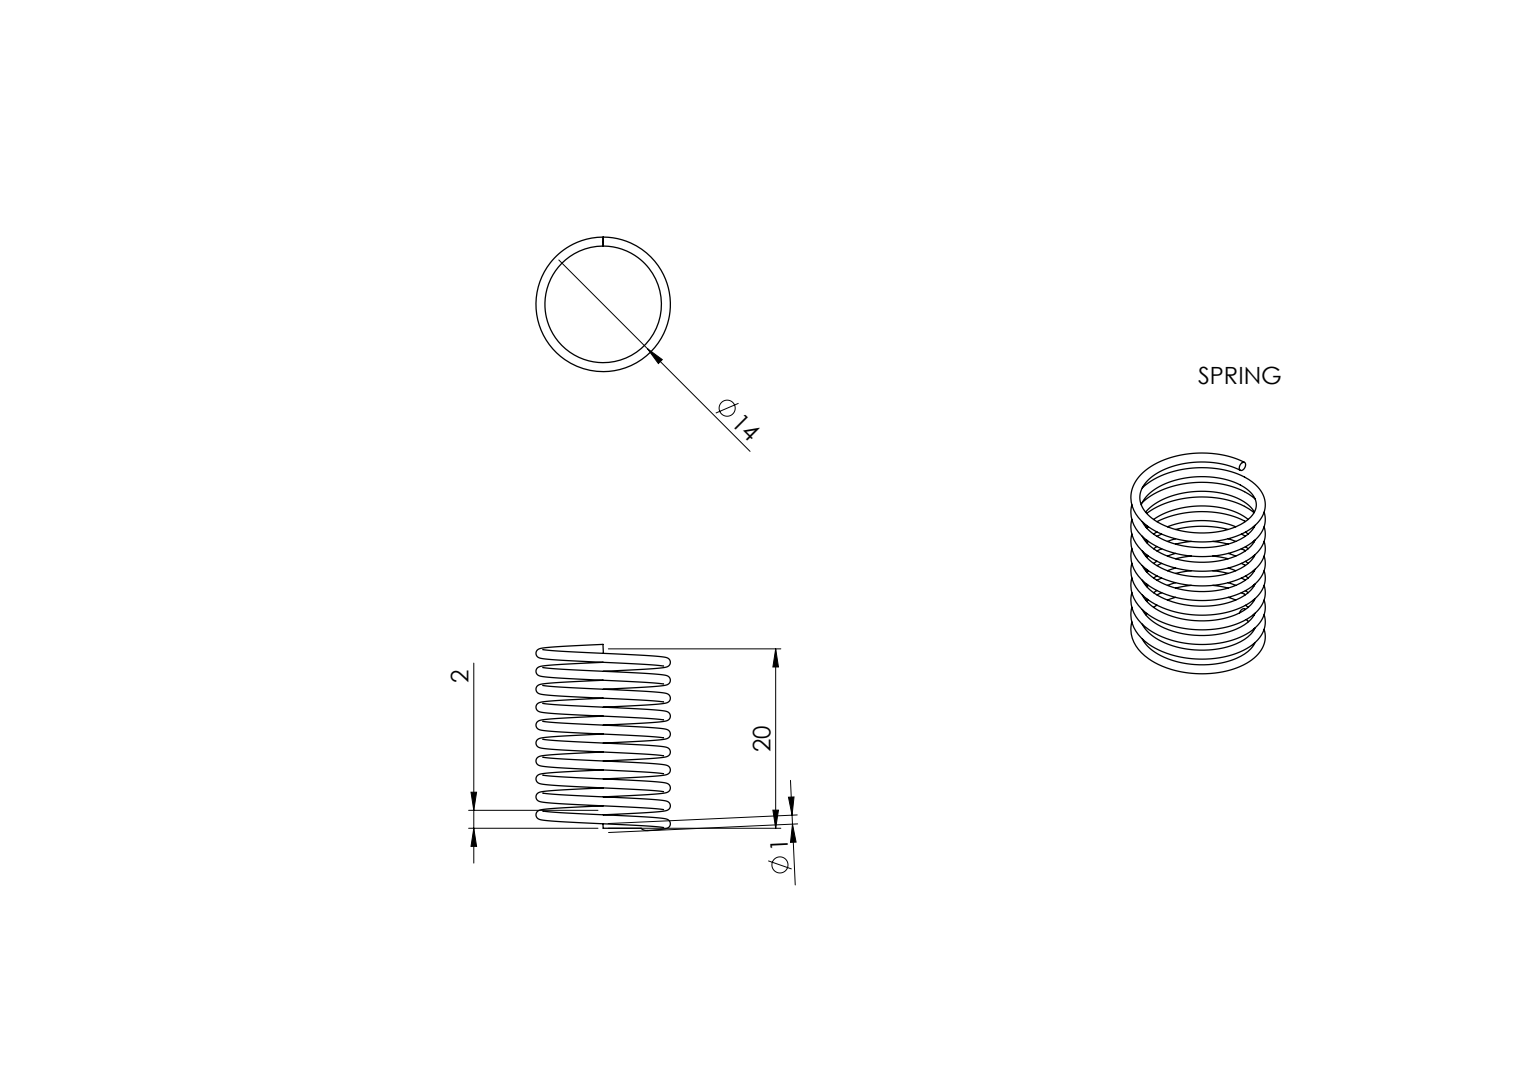
ISO-10303-21;
HEADER;
FILE_DESCRIPTION (('STEP AP214'),
    '1' );
FILE_NAME ('spring.step',
    '2026-10-25T07:12:54',
    ( '' ),
    ( '' ),
    'SwSTEP 2.0',
    'SolidWorks 2026',
    '' );
FILE_SCHEMA (( 'AUTOMOTIVE_DESIGN' ));
ENDSEC;

DATA;
#1=CARTESIAN_POINT ( 'NONE',  ( 44.30067958973594955, 46.10051614449766078, -1.875703265242155693 ) ) ;
#2=CARTESIAN_POINT ( 'NONE',  ( 43.33558569842706021, 59.90051614449766504, 2.141517661632167169 ) ) ;
#3=CARTESIAN_POINT ( 'NONE',  ( 56.81924384183011512, 48.19948385550240744, 4.924951120819313743 ) ) ;
#5=CARTESIAN_POINT ( 'NONE',  ( 49.97728705011495265, 53.50051614449767357, 8.000000000000001776 ) ) ;
#17=CARTESIAN_POINT ( 'NONE',  ( 44.28664221472220675, 51.09948385550240602, -1.832500667257165317 ) ) ;
#18=CARTESIAN_POINT ( 'NONE',  ( 44.03140696652193498, 63.19948385550240744, -4.306917132069424170 ) ) ;
#20=CARTESIAN_POINT ( 'NONE',  ( 47.70284917648459100, 63.60051614449766078, 6.992620115222796251 ) ) ;
#22=EDGE_CURVE ( 'NONE', #9726, #725, #6704, .T. ) ;
#26=CARTESIAN_POINT ( 'NONE',  ( 57.36023556966787851, 57.00051614449766646, 0.02388180880515038476 ) ) ;
#27=CARTESIAN_POINT ( 'NONE',  ( 55.69932041026404335, 55.89948385550241028, -1.875703265242203432 ) ) ;
#39=CARTESIAN_POINT ( 'NONE',  ( 54.13287192849676188, 50.29948385550240175, 5.649768623646098220 ) ) ;
#42=CARTESIAN_POINT ( 'NONE',  ( 51.97223112728249816, 54.60051614449766788, -5.992620115222793586 ) ) ;
#44=CARTESIAN_POINT ( 'NONE',  ( 49.97728705011488159, 65.49948385550240459, -7.000000000000000888 ) ) ;
#45=CARTESIAN_POINT ( 'NONE',  ( 56.65037692655918988, 61.89948385550241028, -2.184720259617163762 ) ) ;
#46=CARTESIAN_POINT ( 'NONE',  ( 56.65037692655918988, 57.89948385550240317, -2.184720259617163762 ) ) ;
#58=CARTESIAN_POINT ( 'NONE',  ( 56.66441430157296821, 48.09948385550240602, 2.141517661632100111 ) ) ;
#60=CARTESIAN_POINT ( 'NONE',  ( 56.66441430157294690, 48.90051614449766504, -2.141517661632166281 ) ) ;
#62=CARTESIAN_POINT ( 'NONE',  ( 47.42335538002188144, 62.59948385550238470, 8.007379884777233059 ) ) ;
#64=CARTESIAN_POINT ( 'NONE',  ( 56.79116909180255135, 53.79948385550241596, -4.963592699179005585 ) ) ;
#72=CARTESIAN_POINT ( 'NONE',  ( 55.08986747509849380, 47.20051614449766220, 3.727524721679155384 ) ) ;
#73=CARTESIAN_POINT ( 'NONE',  ( 52.25172492374528588, 57.40051614449765793, 7.007379884777204637 ) ) ;
#74=CARTESIAN_POINT ( 'NONE',  ( 52.57664461997811856, 45.59948385550240602, -8.007379884777229506 ) ) ;
#76=CARTESIAN_POINT ( 'NONE',  ( 58.41169779390614281, 55.00051614449766646, 0.02388180880515032231 ) ) ;
#86=CARTESIAN_POINT ( 'NONE',  ( 48.02776887271745210, 49.39948385550241028, -5.992620115222778487 ) ) ;
#88=CARTESIAN_POINT ( 'NONE',  ( 54.72065718078918906, 48.70051614449766930, -6.458785618021089192 ) ) ;
#91=CARTESIAN_POINT ( 'NONE',  ( 47.74827507625469281, 54.40051614449766504, -7.007379884777203749 ) ) ;
#92=CARTESIAN_POINT ( 'NONE',  ( 50.02271294988511841, 56.49948385550240459, 6.000000000000000888 ) ) ;
#107=CARTESIAN_POINT ( 'NONE',  ( 54.13287192849676188, 52.29948385550240886, 5.649768623646098220 ) ) ;
#109=CARTESIAN_POINT ( 'NONE',  ( 53.50833635130544508, 51.30051614449765651, 4.867452303228181343 ) ) ;
#113=CARTESIAN_POINT ( 'NONE',  ( 47.74827507625478518, 60.59948385550239891, 7.007379884777227730 ) ) ;
#125=CARTESIAN_POINT ( 'NONE',  ( 56.65037692655918988, 49.89948385550240317, -2.184720259617163762 ) ) ;
#126=CARTESIAN_POINT ( 'NONE',  ( 56.65037692655921120, 45.10051614449766078, 2.184720259617097593 ) ) ;
#128=CARTESIAN_POINT ( 'NONE',  ( 50.02271294988512551, 48.49948385550240459, 7.000000000000000888 ) ) ;
#130=CARTESIAN_POINT ( 'NONE',  ( 56.81924384183011512, 54.19948385550241454, 4.924951120819313743 ) ) ;
#138=CARTESIAN_POINT ( 'NONE',  ( 46.45491332379576477, 49.70051614449766220, 4.840751629271188961 ) ) ;
#139=CARTESIAN_POINT ( 'NONE',  ( 47.74827507625470702, 60.40051614449766504, -7.007379884777204637 ) ) ;
#140=CARTESIAN_POINT ( 'NONE',  ( 47.37792948025170858, 63.60051614449764656, 7.992620115222797139 ) ) ;
#143=CARTESIAN_POINT ( 'NONE',  ( 47.37792948025170858, 53.60051614449765367, 7.992620115222797139 ) ) ;
#144=B_SPLINE_CURVE_WITH_KNOTS ( 'NONE', 3,
 ( #13141, #2570, #7772, #10101, #12115, #12051, #4654, #11983, #6798, #4863, #3822, #8039 ),
 .UNSPECIFIED., .F., .F.,
 ( 4, 2, 2, 2, 2, 4 ),
 ( 0.01755862241325779893, 0.01812962329865995884, 0.01870062418406211874, 0.01984262595486643854, 0.02098462772567075835, 0.02212662949647507815 ),
 .UNSPECIFIED. ) ;
#155=CARTESIAN_POINT ( 'NONE',  ( 55.71335778527780747, 50.09948385550240602, 1.832500667257165983 ) ) ;
#156=CARTESIAN_POINT ( 'NONE',  ( 47.74827507625477807, 64.59948385550239891, 7.007379884777229506 ) ) ;
#158=CARTESIAN_POINT ( 'NONE',  ( 45.90387839640208512, 64.30051614449766362, -5.676469297603124353 ) ) ;
#161=CARTESIAN_POINT ( 'NONE',  ( 45.90387839640208512, 54.30051614449765651, -5.676469297603124353 ) ) ;
#162=CARTESIAN_POINT ( 'NONE',  ( 55.11794222512601493, 60.19948385550240744, 3.688883143319541702 ) ) ;
#170=CARTESIAN_POINT ( 'NONE',  ( 45.86712807150323812, 53.29948385550240886, -5.649768623646098220 ) ) ;
#172=CARTESIAN_POINT ( 'NONE',  ( 48.02776887271750184, 51.60051614449766788, 5.992620115222795363 ) ) ;
#176=CARTESIAN_POINT ( 'NONE',  ( 55.94051828345050836, 57.79948385550238754, -4.345558710429104465 ) ) ;
#185=( NAMED_UNIT ( * ) SI_UNIT ( $, .STERADIAN. ) SOLID_ANGLE_UNIT ( ) );
#187=CARTESIAN_POINT ( 'NONE',  ( 45.86712807150323812, 51.29948385550240175, -5.649768623646098220 ) ) ;
#188=CARTESIAN_POINT ( 'NONE',  ( 47.74827507625469281, 56.40051614449766504, -7.007379884777203749 ) ) ;
#191=CARTESIAN_POINT ( 'NONE',  ( 54.72065718078924590, 64.29948385550240175, 6.458785618021043895 ) ) ;
#196=CARTESIAN_POINT ( 'NONE',  ( 45.27934281921075410, 57.29948385550240175, -6.458785618021043895 ) ) ;
#203=CARTESIAN_POINT ( 'NONE',  ( 43.69122665457040000, 56.00051614449765935, -0.02388180880515696977 ) ) ;
#206=CARTESIAN_POINT ( 'NONE',  ( 54.68390685589033495, 45.69948385550240033, -6.485486291978119766 ) ) ;
#209=CARTESIAN_POINT ( 'NONE',  ( 45.27934281921082516, 53.70051614449766220, 6.458785618021089192 ) ) ;
#210=ORIENTED_EDGE ( 'NONE', *, *, #1266, .T. ) ;
#222=CARTESIAN_POINT ( 'NONE',  ( 51.97223112728254790, 50.39948385550241738, 5.992620115222778487 ) ) ;
#223=CARTESIAN_POINT ( 'NONE',  ( 43.33558569842703179, 63.09948385550240602, -2.141517661632099223 ) ) ;
#224=CARTESIAN_POINT ( 'NONE',  ( 41.58830220609386430, 48.00051614449766646, -0.02388180880514929535 ) ) ;
#228=CARTESIAN_POINT ( 'NONE',  ( 56.65037692655921120, 57.10051614449766078, 2.184720259617097593 ) ) ;
#230=CARTESIAN_POINT ( 'NONE',  ( 55.71335778527780747, 58.09948385550241312, 1.832500667257165983 ) ) ;
#238=CARTESIAN_POINT ( 'NONE',  ( 45.90387839640214196, 48.69948385550240744, 5.676469297603166098 ) ) ;
#240=CARTESIAN_POINT ( 'NONE',  ( 43.69122665457040000, 60.00051614449765935, -0.02388180880515696977 ) ) ;
#243=CARTESIAN_POINT ( 'NONE',  ( 52.29715082351547295, 60.39948385550239607, 6.992620115222774047 ) ) ;
#253=CARTESIAN_POINT ( 'NONE',  ( 43.34962307344081012, 54.89948385550240317, 2.184720259617164650 ) ) ;
#254=CARTESIAN_POINT ( 'NONE',  ( 56.65037692655921120, 55.10051614449766078, 2.184720259617097593 ) ) ;
#257=CARTESIAN_POINT ( 'NONE',  ( 43.33558569842703179, 49.09948385550240602, -2.141517661632099223 ) ) ;
#259=CARTESIAN_POINT ( 'NONE',  ( 47.42335538002188144, 62.59948385550238470, 8.007379884777233059 ) ) ;
#269=CARTESIAN_POINT ( 'NONE',  ( 46.45491332379576477, 51.70051614449765509, 4.840751629271188961 ) ) ;
#271=CARTESIAN_POINT ( 'NONE',  ( 52.57664461997811856, 51.59948385550240602, -8.007379884777229506 ) ) ;
#273=CARTESIAN_POINT ( 'NONE',  ( 55.96859303347804371, 56.19948385550241454, 4.306917132069425946 ) ) ;
#275=CARTESIAN_POINT ( 'NONE',  ( 47.42335538002180328, 58.40051614449765793, -8.007379884777206414 ) ) ;
#287=CARTESIAN_POINT ( 'NONE',  ( 50.02271294988511841, 54.49948385550240459, 6.000000000000000888 ) ) ;
#288=CARTESIAN_POINT ( 'NONE',  ( 44.03140696652198471, 47.80051614449764941, 4.306917132069485454 ) ) ;
#289=CARTESIAN_POINT ( 'NONE',  ( 52.25172492374527877, 63.40051614449765793, 7.007379884777203749 ) ) ;
#292=CARTESIAN_POINT ( 'NONE',  ( 47.70284917648459100, 59.60051614449765367, 6.992620115222796251 ) ) ;
#300=CARTESIAN_POINT ( 'NONE',  ( 55.94051828345050836, 55.79948385550238044, -4.345558710429104465 ) ) ;
#302=CARTESIAN_POINT ( 'NONE',  ( 48.07319477248762496, 60.40051614449765793, -6.007379884777208190 ) ) ;
#307=CARTESIAN_POINT ( 'NONE',  ( 56.65037692655918988, 63.89948385550239607, -2.184720259617163762 ) ) ;
#321=CARTESIAN_POINT ( 'NONE',  ( 50.02271294988512551, 54.49948385550240459, 7.000000000000000888 ) ) ;
#323=CARTESIAN_POINT ( 'NONE',  ( 56.66441430157294690, 54.90051614449765793, -2.141517661632166281 ) ) ;
#326=CARTESIAN_POINT ( 'NONE',  ( 45.90387839640214196, 54.69948385550240744, 5.676469297603166098 ) ) ;
#327=CARTESIAN_POINT ( 'NONE',  ( 55.94051828345050836, 49.79948385550240175, -4.345558710429104465 ) ) ;
#329=CARTESIAN_POINT ( 'NONE',  ( 50.02271294988513972, 64.49948385550239038, 8.000000000000001776 ) ) ;
#334=AXIS2_PLACEMENT_3D ( 'NONE', #11503, #2020, #12598 ) ;
#336=CARTESIAN_POINT ( 'NONE',  ( 48.07319477248762496, 54.40051614449765793, -6.007379884777208190 ) ) ;
#337=CARTESIAN_POINT ( 'NONE',  ( 47.74827507625470702, 64.40051614449765793, -7.007379884777204637 ) ) ;
#338=CARTESIAN_POINT ( 'NONE',  ( 56.79116909180255135, 49.79948385550240175, -4.963592699179005585 ) ) ;
#339=CARTESIAN_POINT ( 'NONE',  ( 43.33558569842703179, 59.09948385550240602, -2.141517661632099223 ) ) ;
#342=CARTESIAN_POINT ( 'NONE',  ( 47.42335538002180328, 60.40051614449765793, -8.007379884777206414 ) ) ;
#353=CARTESIAN_POINT ( 'NONE',  ( 53.50833635130540955, 59.69948385550240744, -4.867452303228209765 ) ) ;
#354=CARTESIAN_POINT ( 'NONE',  ( 43.34962307344078880, 50.10051614449766078, -2.184720259617096705 ) ) ;
#355=CARTESIAN_POINT ( 'NONE',  ( 52.57664461997821093, 55.40051614449767214, 8.007379884777206414 ) ) ;
#359=CARTESIAN_POINT ( 'NONE',  ( 52.29715082351538769, 62.60051614449766078, -6.992620115222796251 ) ) ;
#368=CARTESIAN_POINT ( 'NONE',  ( 47.74827507625478518, 54.59948385550239180, 7.007379884777227730 ) ) ;
#369=CARTESIAN_POINT ( 'NONE',  ( 44.91013252490150620, 58.20051614449766220, -3.727524721679154940 ) ) ;
#372=CARTESIAN_POINT ( 'NONE',  ( 43.33558569842706021, 45.90051614449765793, 2.141517661632167169 ) ) ;
#373=CARTESIAN_POINT ( 'NONE',  ( 55.71335778527780747, 46.09948385550240602, 1.832500667257165983 ) ) ;
#383=ADVANCED_BREP_SHAPE_REPRESENTATION ( '', ( #5648, #430 ), #3304 ) ;
#384=CARTESIAN_POINT ( 'NONE',  ( 44.05948171654945611, 52.20051614449764799, -4.345558710429044069 ) ) ;
#386=CARTESIAN_POINT ( 'NONE',  ( 55.94051828345050836, 49.79948385550240175, -4.345558710429104465 ) ) ;
#387=CARTESIAN_POINT ( 'NONE',  ( 57.36023556966787851, 47.99948385550239038, -0.02388180880522424582 ) ) ;
#388=CARTESIAN_POINT ( 'NONE',  ( 58.41169779390614281, 59.99948385550241170, -0.02388180880523160798 ) ) ;
#397=STYLED_ITEM('',(#13705),#5648);
#398=CARTESIAN_POINT ( 'NONE',  ( 48.02776887271750184, 55.60051614449765367, 5.992620115222795363 ) ) ;
#399=CARTESIAN_POINT ( 'NONE',  ( 45.86712807150329496, 63.70051614449766220, 5.649768623646139964 ) ) ;
#400=CARTESIAN_POINT ( 'NONE',  ( 49.97728705011486738, 51.49948385550240459, -8.000000000000001776 ) ) ;
#401=CARTESIAN_POINT ( 'NONE',  ( 54.13287192849676188, 56.29948385550240175, 5.649768623646098220 ) ) ;
#403=CARTESIAN_POINT ( 'NONE',  ( 56.81924384183006538, 60.80051614449766362, -4.924951120819380357 ) ) ;
#412=CARTESIAN_POINT ( 'NONE',  ( 49.97728705011488870, 53.49948385550240459, -6.000000000000000888 ) ) ;
#413=CARTESIAN_POINT ( 'NONE',  ( 56.13503143586221000, 44.82443585060838132, -3.788959942617806220 ) ) ;
#414=CARTESIAN_POINT ( 'NONE',  ( 56.79116909180259398, 53.20051614449766220, 4.963592699178938972 ) ) ;
#418=CARTESIAN_POINT ( 'NONE',  ( 54.13287192849671214, 60.70051614449766220, -5.649768623646139964 ) ) ;
#429=CARTESIAN_POINT ( 'NONE',  ( 52.29715082351547295, 60.39948385550239607, 6.992620115222774047 ) ) ;
#430=AXIS2_PLACEMENT_3D ( 'NONE', #5828, #10990, #3471 ) ;
#433=CARTESIAN_POINT ( 'NONE',  ( 43.69122665457040000, 56.00051614449765935, -0.02388180880515696977 ) ) ;
#436=CARTESIAN_POINT ( 'NONE',  ( 55.71335778527780036, 62.90051614449765083, -1.832500667257213056 ) ) ;
#437=CARTESIAN_POINT ( 'NONE',  ( 55.08986747509847248, 45.79948385550240886, -3.727524721679197572 ) ) ;
#449=CARTESIAN_POINT ( 'NONE',  ( 52.29715082351538769, 54.60051614449766788, -6.992620115222796251 ) ) ;
#451=CARTESIAN_POINT ( 'NONE',  ( 55.96859303347804371, 54.19948385550240033, 4.306917132069425946 ) ) ;
#452=CARTESIAN_POINT ( 'NONE',  ( 55.96859303347804371, 50.19948385550240744, 4.306917132069425946 ) ) ;
#455=CARTESIAN_POINT ( 'NONE',  ( 57.36023556966787851, 45.99948385550238328, -0.02388180880522424582 ) ) ;
#464=CARTESIAN_POINT ( 'NONE',  ( 50.02271294988506156, 52.50051614449766646, -6.000000000000000888 ) ) ;
#466=CARTESIAN_POINT ( 'NONE',  ( 52.62207051974839089, 50.39948385550241738, 7.992620115222770494 ) ) ;
#467=CARTESIAN_POINT ( 'NONE',  ( 43.34962307344081012, 58.89948385550241028, 2.184720259617164650 ) ) ;
#469=CARTESIAN_POINT ( 'NONE',  ( 45.31609314410960820, 64.30051614449766362, -6.485486291978072693 ) ) ;
#479=CARTESIAN_POINT ( 'NONE',  ( 48.07319477248768180, 54.59948385550240602, 6.007379884777225953 ) ) ;
#480=CARTESIAN_POINT ( 'NONE',  ( 42.63976443033212149, 48.00051614449766646, -0.02388180880514948964 ) ) ;
#481=CARTESIAN_POINT ( 'NONE',  ( 52.62207051974829852, 54.60051614449766788, -7.992620115222797139 ) ) ;
#485=CARTESIAN_POINT ( 'NONE',  ( 45.90387839640208512, 64.30051614449766362, -5.676469297603124353 ) ) ;
#494=CARTESIAN_POINT ( 'NONE',  ( 43.33558569842703179, 55.09948385550241312, -2.141517661632099223 ) ) ;
#496=CARTESIAN_POINT ( 'NONE',  ( 49.97728705011494554, 57.50051614449766646, 6.000000000000000888 ) ) ;
#500=CARTESIAN_POINT ( 'NONE',  ( 48.02776887271750184, 63.60051614449764656, 5.992620115222795363 ) ) ;
#501=CARTESIAN_POINT ( 'NONE',  ( 47.70284917648453415, 63.39948385550240317, -6.992620115222774047 ) ) ;
#506=UNCERTAINTY_MEASURE_WITH_UNIT (LENGTH_MEASURE( 1.000000000000000082E-05 ), #4482, 'distance_accuracy_value', 'NONE');
#514=CARTESIAN_POINT ( 'NONE',  ( 57.36023556966787851, 57.00051614449766646, 0.02388180880515038476 ) ) ;
#518=CARTESIAN_POINT ( 'NONE',  ( 43.34962307344081012, 48.89948385550240317, 2.184720259617164650 ) ) ;
#519=CARTESIAN_POINT ( 'NONE',  ( 56.81924384183011512, 60.19948385550240744, 4.924951120819313743 ) ) ;
#527=CARTESIAN_POINT ( 'NONE',  ( 43.69122665457040000, 64.00051614449765225, -0.02388180880515696977 ) ) ;
#530=CARTESIAN_POINT ( 'NONE',  ( 45.27934281921075410, 53.29948385550240886, -6.458785618021043895 ) ) ;
#531=CARTESIAN_POINT ( 'NONE',  ( 54.09612160359786515, 53.69948385550240744, -5.676469297603166098 ) ) ;
#534=CARTESIAN_POINT ( 'NONE',  ( 42.39856655714564226, 62.10051614449765367, -2.493737253992044156 ) ) ;
#544=CARTESIAN_POINT ( 'NONE',  ( 51.97223112728254790, 56.39948385550241028, 5.992620115222778487 ) ) ;
#545=CARTESIAN_POINT ( 'NONE',  ( 56.65037692655921120, 53.10051614449766078, 2.184720259617097593 ) ) ;
#546=CARTESIAN_POINT ( 'NONE',  ( 41.58830220609386430, 54.00051614449765935, -0.02388180880514929535 ) ) ;
#549=CARTESIAN_POINT ( 'NONE',  ( 43.33558569842706021, 63.90051614449765793, 2.141517661632167169 ) ) ;
#556=CARTESIAN_POINT ( 'NONE',  ( 55.96859303347804371, 58.19948385550241454, 4.306917132069425946 ) ) ;
#557=CARTESIAN_POINT ( 'NONE',  ( 43.33558569842703179, 55.09948385550241312, -2.141517661632099223 ) ) ;
#563=CARTESIAN_POINT ( 'NONE',  ( 44.03140696652198471, 45.80051614449764230, 4.306917132069485454 ) ) ;
#564=CARTESIAN_POINT ( 'NONE',  ( 47.70284917648453415, 65.39948385550239607, -6.992620115222774047 ) ) ;
#574=CARTESIAN_POINT ( 'NONE',  ( 54.09612160359792199, 61.30051614449766362, 5.676469297603124353 ) ) ;
#577=CARTESIAN_POINT ( 'NONE',  ( 45.90387839640214196, 60.69948385550240033, 5.676469297603166098 ) ) ;
#578=CARTESIAN_POINT ( 'NONE',  ( 47.74827507625478518, 50.59948385550238470, 7.007379884777227730 ) ) ;
#586=CARTESIAN_POINT ( 'NONE',  ( 51.92680522751238925, 59.40051614449765793, 6.007379884777208190 ) ) ;
#589=CARTESIAN_POINT ( 'NONE',  ( 50.02271294988513972, 62.49948385550240459, 8.000000000000001776 ) ) ;
#591=CARTESIAN_POINT ( 'NONE',  ( 43.34962307344081012, 62.89948385550241028, 2.184720259617164650 ) ) ;
#593=CARTESIAN_POINT ( 'NONE',  ( 43.20883090819745576, 50.79948385550240175, 4.963592699179006473 ) ) ;
#605=CARTESIAN_POINT ( 'NONE',  ( 51.97223112728254790, 60.39948385550241028, 5.992620115222778487 ) ) ;
#606=CARTESIAN_POINT ( 'NONE',  ( 56.66441430157294690, 52.90051614449765793, -2.141517661632166281 ) ) ;
#607=CARTESIAN_POINT ( 'NONE',  ( 42.38452918213190657, 61.90051614449766504, 2.450534656007115508 ) ) ;
#611=CARTESIAN_POINT ( 'NONE',  ( 54.09612160359792199, 63.30051614449766362, 5.676469297603124353 ) ) ;
#621=CARTESIAN_POINT ( 'NONE',  ( 53.50833635130540955, 45.69948385550240033, -4.867452303228209765 ) ) ;
#622=CARTESIAN_POINT ( 'NONE',  ( 56.66441430157296821, 56.09948385550240602, 2.141517661632100111 ) ) ;
#628=CARTESIAN_POINT ( 'NONE',  ( 53.50833635130544508, 63.30051614449767072, 4.867452303228181343 ) ) ;
#629=CARTESIAN_POINT ( 'NONE',  ( 48.02776887271745210, 51.39948385550241028, -5.992620115222778487 ) ) ;
#641=CARTESIAN_POINT ( 'NONE',  ( 45.86712807150329496, 59.70051614449766220, 5.649768623646139964 ) ) ;
#643=CARTESIAN_POINT ( 'NONE',  ( 44.88205777487398507, 65.19948385550240744, -3.688883143319540814 ) ) ;
#645=CARTESIAN_POINT ( 'NONE',  ( 44.03140696652192787, 61.19948385550239323, -4.306917132069425058 ) ) ;
#646=CARTESIAN_POINT ( 'NONE',  ( 54.09612160359786515, 51.69948385550240744, -5.676469297603166098 ) ) ;
#647=CARTESIAN_POINT ( 'NONE',  ( 56.66441430157296821, 50.09948385550240602, 2.141517661632100111 ) ) ;
#657=CARTESIAN_POINT ( 'NONE',  ( 55.11794222512599362, 60.80051614449766362, -3.688883143319583446 ) ) ;
#659=CARTESIAN_POINT ( 'NONE',  ( 47.37792948025162332, 61.39948385550240317, -7.992620115222770494 ) ) ;
#663=CARTESIAN_POINT ( 'NONE',  ( 56.79116909180255135, 47.79948385550240886, -4.963592699179005585 ) ) ;
#676=CARTESIAN_POINT ( 'NONE',  ( 55.11794222512599362, 44.80051614449766362, -3.688883143319583446 ) ) ;
#677=CARTESIAN_POINT ( 'NONE',  ( 45.86712807150329496, 53.70051614449766220, 5.649768623646139964 ) ) ;
#678=CARTESIAN_POINT ( 'NONE',  ( 42.39856655714564226, 56.10051614449766078, -2.493737253992044156 ) ) ;
#684=CARTESIAN_POINT ( 'NONE',  ( 42.38452918213190657, 49.90051614449766504, 2.450534656007115508 ) ) ;
#697=CARTESIAN_POINT ( 'NONE',  ( 43.33558569842703179, 65.09948385550239891, -2.141517661632099223 ) ) ;
#698=CARTESIAN_POINT ( 'NONE',  ( 42.63976443033212149, 58.99948385550239038, 0.02388180880522514787 ) ) ;
#702=CARTESIAN_POINT ( 'NONE',  ( 49.97728705011495265, 53.50051614449765935, 7.000000000000000888 ) ) ;
#703=CARTESIAN_POINT ( 'NONE',  ( 51.92680522751233951, 49.59948385550241312, -6.007379884777223289 ) ) ;
#716=CARTESIAN_POINT ( 'NONE',  ( 55.71335778527780036, 44.90051614449765793, -1.832500667257213056 ) ) ;
#718=CARTESIAN_POINT ( 'NONE',  ( 43.33558569842703179, 57.09948385550240602, -2.141517661632099223 ) ) ;
#719=CARTESIAN_POINT ( 'NONE',  ( 44.03140696652192787, 53.19948385550238612, -4.306917132069425058 ) ) ;
#721=CARTESIAN_POINT ( 'NONE',  ( 44.03140696652192787, 51.19948385550238612, -4.306917132069425058 ) ) ;
#724=CARTESIAN_POINT ( 'NONE',  ( 62.49999999999998579, 45.00000000000001421, -5.000000000000000000 ) ) ;
#725=VERTEX_POINT ( 'NONE', #11778 ) ;
#731=CARTESIAN_POINT ( 'NONE',  ( 44.28664221472221385, 57.90051614449765793, 1.832500667257213722 ) ) ;
#733=CARTESIAN_POINT ( 'NONE',  ( 42.39856655714566358, 56.89948385550240317, 2.493737253992119207 ) ) ;
#734=CARTESIAN_POINT ( 'NONE',  ( 45.86712807150323812, 63.29948385550240886, -5.649768623646098220 ) ) ;
#737=CARTESIAN_POINT ( 'NONE',  ( 54.68390685589033495, 51.69948385550241454, -6.485486291978119766 ) ) ;
#745=B_SPLINE_CURVE_WITH_KNOTS ( 'NONE', 3,
 ( #13610, #3044, #9471, #11483, #1864, #10442 ),
 .UNSPECIFIED., .F., .F.,
 ( 4, 2, 4 ),
 ( 0.000000000000000000, 0.0003657767439067419277, 0.0007315534878134838555 ),
 .UNSPECIFIED. ) ;
#750=CARTESIAN_POINT ( 'NONE',  ( 43.69122665457040000, 64.99948385550240459, 0.02388180880521036456 ) ) ;
#751=CARTESIAN_POINT ( 'NONE',  ( 47.74827507625470702, 52.40051614449765083, -7.007379884777204637 ) ) ;
#753=CARTESIAN_POINT ( 'NONE',  ( 45.27934281921082516, 57.70051614449766930, 6.458785618021089192 ) ) ;
#756=CARTESIAN_POINT ( 'NONE',  ( 56.81924384183006538, 52.80051614449766362, -4.924951120819380357 ) ) ;
#767=CARTESIAN_POINT ( 'NONE',  ( 44.91013252490152752, 46.79948385550240886, 3.727524721679198461 ) ) ;
#768=CARTESIAN_POINT ( 'NONE',  ( 45.90387839640214196, 60.69948385550240033, 5.676469297603166098 ) ) ;
#774=CARTESIAN_POINT ( 'NONE',  ( 47.70284917648459100, 53.60051614449765367, 6.992620115222796251 ) ) ;
#775=CARTESIAN_POINT ( 'NONE',  ( 44.28664221472220675, 55.09948385550241312, -1.832500667257165317 ) ) ;
#786=CARTESIAN_POINT ( 'NONE',  ( 49.97728705011488159, 47.49948385550240459, -7.000000000000000888 ) ) ;
#789=CARTESIAN_POINT ( 'NONE',  ( 48.02776887271750184, 45.60051614449765367, 5.992620115222795363 ) ) ;
#791=CARTESIAN_POINT ( 'NONE',  ( 54.09612160359786515, 55.69948385550240744, -5.676469297603166098 ) ) ;
#792=CARTESIAN_POINT ( 'NONE',  ( 55.94051828345050836, 51.79948385550240175, -4.345558710429104465 ) ) ;
#794=CARTESIAN_POINT ( 'NONE',  ( 54.13287192849676188, 52.29948385550240886, 5.649768623646098220 ) ) ;
#797=LINE ( 'NONE', #724, #5719 ) ;
#802=CARTESIAN_POINT ( 'NONE',  ( 43.69122665457040000, 60.00051614449765935, -0.02388180880515696977 ) ) ;
#804=CARTESIAN_POINT ( 'NONE',  ( 58.41169779390614281, 61.99948385550241170, -0.02388180880523160798 ) ) ;
#806=CARTESIAN_POINT ( 'NONE',  ( 45.31609314410967926, 50.69948385550240744, 6.485486291978119766 ) ) ;
#815=CARTESIAN_POINT ( 'NONE',  ( 46.49166364869460466, 64.69948385550240744, 4.867452303228209765 ) ) ;
#816=CARTESIAN_POINT ( 'NONE',  ( 44.05948171654945611, 56.20051614449765509, -4.345558710429044069 ) ) ;
#817=CARTESIAN_POINT ( 'NONE',  ( 52.57664461997821093, 61.40051614449765793, 8.007379884777206414 ) ) ;
#819=CARTESIAN_POINT ( 'NONE',  ( 57.60143344285435774, 47.10051614449766078, 2.493737253992045044 ) ) ;
#829=CARTESIAN_POINT ( 'NONE',  ( 47.74827507625478518, 64.59948385550239891, 7.007379884777227730 ) ) ;
#831=CARTESIAN_POINT ( 'NONE',  ( 52.29715082351547295, 56.39948385550239607, 6.992620115222774047 ) ) ;
#836=CARTESIAN_POINT ( 'NONE',  ( 55.48859070151218020, 45.00000000000002132, -4.999999999999993783 ) ) ;
#837=CARTESIAN_POINT ( 'NONE',  ( 54.13287192849671214, 50.70051614449766220, -5.649768623646139964 ) ) ;
#838=CARTESIAN_POINT ( 'NONE',  ( 49.97728705011488870, 49.49948385550241170, -6.000000000000000888 ) ) ;
#839=CARTESIAN_POINT ( 'NONE',  ( 55.00886502606627459, 44.74918607449495767, -5.000000000000008882 ) ) ;
#858=CARTESIAN_POINT ( 'NONE',  ( 51.92680522751233951, 63.59948385550239891, -6.007379884777223289 ) ) ;
#861=CARTESIAN_POINT ( 'NONE',  ( 55.96859303347804371, 56.19948385550241454, 4.306917132069425946 ) ) ;
#863=CARTESIAN_POINT ( 'NONE',  ( 44.05948171654949874, 50.79948385550238754, 4.345558710429105354 ) ) ;
#872=CARTESIAN_POINT ( 'NONE',  ( 55.96859303347805081, 46.19948385550240033, 4.306917132069425058 ) ) ;
#873=CARTESIAN_POINT ( 'NONE',  ( 54.09612160359792199, 49.30051614449765651, 5.676469297603124353 ) ) ;
#874=CARTESIAN_POINT ( 'NONE',  ( 54.23491683972284960, 45.00000000000001421, -4.999999999999999112 ) ) ;
#875=CARTESIAN_POINT ( 'NONE',  ( 56.79116909180255135, 61.79948385550240175, -4.963592699179005585 ) ) ;
#879=CARTESIAN_POINT ( 'NONE',  ( 47.42335538002188144, 48.59948385550239891, 8.007379884777233059 ) ) ;
#890=CARTESIAN_POINT ( 'NONE',  ( 55.71335778527780747, 60.09948385550240602, 1.832500667257165983 ) ) ;
#891=CARTESIAN_POINT ( 'NONE',  ( 55.94051828345054389, 57.20051614449766220, 4.345558710429044957 ) ) ;
#892=CARTESIAN_POINT ( 'NONE',  ( 42.38452918213190657, 57.90051614449765793, 2.450534656007115508 ) ) ;
#894=CARTESIAN_POINT ( 'NONE',  ( 50.02271294988505446, 52.50051614449766646, -8.000000000000001776 ) ) ;
#903=DIRECTION ( 'NONE',  ( -0.04542589977017699732, 0.9989677110047501252, 0.000000000000000000 ) ) ;
#906=CARTESIAN_POINT ( 'NONE',  ( 49.97728705011488159, 61.49948385550240459, -7.000000000000000888 ) ) ;
#908=CARTESIAN_POINT ( 'NONE',  ( 43.33558569842703179, 57.09948385550240602, -2.141517661632099223 ) ) ;
#911=CARTESIAN_POINT ( 'NONE',  ( 54.09612160359792199, 57.30051614449765651, 5.676469297603124353 ) ) ;
#915=CARTESIAN_POINT ( 'NONE',  ( 47.74827507625469281, 50.40051614449764372, -7.007379884777203749 ) ) ;
#916=CARTESIAN_POINT ( 'NONE',  ( 55.71335778527780747, 50.09948385550240602, 1.832500667257165983 ) ) ;
#930=CARTESIAN_POINT ( 'NONE',  ( 44.91013252490150620, 48.20051614449766930, -3.727524721679154940 ) ) ;
#933=CARTESIAN_POINT ( 'NONE',  ( 55.94051828345050836, 61.79948385550239465, -4.345558710429104465 ) ) ;
#934=CARTESIAN_POINT ( 'NONE',  ( 55.96859303347804371, 54.19948385550240033, 4.306917132069425946 ) ) ;
#937=ORIENTED_EDGE ( 'NONE', *, *, #11649, .F. ) ;
#938=CARTESIAN_POINT ( 'NONE',  ( 49.97728705011488159, 53.49948385550240459, -7.000000000000000888 ) ) ;
#946=CARTESIAN_POINT ( 'NONE',  ( 55.96859303347802239, 48.80051614449766362, -4.306917132069484566 ) ) ;
#948=CARTESIAN_POINT ( 'NONE',  ( 42.38452918213188525, 65.09948385550239891, -2.450534656007040013 ) ) ;
#949=CARTESIAN_POINT ( 'NONE',  ( 42.39856655714566358, 56.89948385550240317, 2.493737253992119207 ) ) ;
#956=CARTESIAN_POINT ( 'NONE',  ( 44.28664221472221385, 47.90051614449765793, 1.832500667257213722 ) ) ;
#957=CARTESIAN_POINT ( 'NONE',  ( 44.05948171654945611, 62.20051614449765509, -4.345558710429044069 ) ) ;
#959=CARTESIAN_POINT ( 'NONE',  ( 47.42335538002188144, 46.59948385550239891, 8.007379884777233059 ) ) ;
#964=CARTESIAN_POINT ( 'NONE',  ( 52.57664461997821093, 47.40051614449765793, 8.007379884777206414 ) ) ;
#976=CARTESIAN_POINT ( 'NONE',  ( 49.97728705011488870, 47.49948385550240459, -6.000000000000000888 ) ) ;
#978=CARTESIAN_POINT ( 'NONE',  ( 42.63976443033212860, 58.00051614449765225, -0.02388180880514948964 ) ) ;
#982=CARTESIAN_POINT ( 'NONE',  ( 50.02271294988505446, 52.50051614449765935, -7.000000000000000888 ) ) ;
#983=CARTESIAN_POINT ( 'NONE',  ( 55.71335778527780747, 56.09948385550240602, 1.832500667257165983 ) ) ;
#997=CARTESIAN_POINT ( 'NONE',  ( 49.97728705011494554, 53.50051614449767357, 6.000000000000000888 ) ) ;
#999=CARTESIAN_POINT ( 'NONE',  ( 54.13287192849676188, 62.29948385550240886, 5.649768623646098220 ) ) ;
#1000=CARTESIAN_POINT ( 'NONE',  ( 45.90387839640214196, 60.69948385550240033, 5.676469297603166098 ) ) ;
#1001=CARTESIAN_POINT ( 'NONE',  ( 52.25172492374522903, 61.59948385550239891, -7.007379884777225953 ) ) ;
#1008=CARTESIAN_POINT ( 'NONE',  ( 50.02271294988512551, 46.49948385550240459, 7.000000000000000888 ) ) ;
#1010=CARTESIAN_POINT ( 'NONE',  ( 45.90387839640208512, 50.30051614449766362, -5.676469297603124353 ) ) ;
#1014=CARTESIAN_POINT ( 'NONE',  ( 45.90387839640214196, 46.69948385550240744, 5.676469297603166098 ) ) ;
#1016=PLANE ( 'NONE',  #1563 ) ;
#1017=CARTESIAN_POINT ( 'NONE',  ( 42.39856655714566358, 58.89948385550241028, 2.493737253992119207 ) ) ;
#1026=CARTESIAN_POINT ( 'NONE',  ( 44.30067958973594955, 50.10051614449766078, -1.875703265242155693 ) ) ;
#1027=CARTESIAN_POINT ( 'NONE',  ( 45.90387839640208512, 58.30051614449766362, -5.676469297603124353 ) ) ;
#1028=CARTESIAN_POINT ( 'NONE',  ( 42.39856655714566358, 46.89948385550240317, 2.493737253992119207 ) ) ;
#1031=CARTESIAN_POINT ( 'NONE',  ( 45.27934281921082516, 57.70051614449766930, 6.458785618021089192 ) ) ;
#1039=CARTESIAN_POINT ( 'NONE',  ( 49.97728705011488870, 51.49948385550240459, -6.000000000000000888 ) ) ;
#1041=CARTESIAN_POINT ( 'NONE',  ( 50.02271294988505446, 46.50051614449766646, -8.000000000000001776 ) ) ;
#1045=CARTESIAN_POINT ( 'NONE',  ( 52.25172492374527877, 55.40051614449764372, 7.007379884777203749 ) ) ;
#1046=CARTESIAN_POINT ( 'NONE',  ( 46.45491332379572924, 61.29948385550240886, -4.840751629271157874 ) ) ;
#1058=CARTESIAN_POINT ( 'NONE',  ( 42.63976443033212860, 50.99948385550240459, 0.02388180880522514787 ) ) ;
#1060=CARTESIAN_POINT ( 'NONE',  ( 44.30067958973594955, 52.10051614449766788, -1.875703265242155693 ) ) ;
#1062=CARTESIAN_POINT ( 'NONE',  ( 43.33558569842703179, 63.09948385550240602, -2.141517661632099223 ) ) ;
#1063=CARTESIAN_POINT ( 'NONE',  ( 54.09612160359786515, 61.69948385550240744, -5.676469297603166098 ) ) ;
#1064=CARTESIAN_POINT ( 'NONE',  ( 45.90387839640214196, 62.69948385550240744, 5.676469297603166098 ) ) ;
#1072=CARTESIAN_POINT ( 'NONE',  ( 44.05948171654949874, 46.79948385550240175, 4.345558710429104465 ) ) ;
#1073=CARTESIAN_POINT ( 'NONE',  ( 47.70284917648459100, 49.60051614449763946, 6.992620115222796251 ) ) ;
#1075=CARTESIAN_POINT ( 'NONE',  ( 43.33558569842703179, 47.09948385550240602, -2.141517661632099223 ) ) ;
#1078=CARTESIAN_POINT ( 'NONE',  ( 42.38452918213188525, 59.09948385550240602, -2.450534656007040013 ) ) ;
#1089=CARTESIAN_POINT ( 'NONE',  ( 48.02776887271750184, 49.60051614449766788, 5.992620115222795363 ) ) ;
#1090=CARTESIAN_POINT ( 'NONE',  ( 56.66441430157294690, 60.90051614449766504, -2.141517661632166281 ) ) ;
#1092=CARTESIAN_POINT ( 'NONE',  ( 57.61547081786810764, 62.90051614449765083, -2.450534656007114176 ) ) ;
#1096=CARTESIAN_POINT ( 'NONE',  ( 43.20883090819742023, 58.20051614449766220, -4.963592699178938972 ) ) ;
#1107=CARTESIAN_POINT ( 'NONE',  ( 55.69932041026404335, 47.89948385550240317, -1.875703265242203432 ) ) ;
#1108=CARTESIAN_POINT ( 'NONE',  ( 50.02271294988512551, 64.49948385550240459, 7.000000000000000888 ) ) ;
#1109=CARTESIAN_POINT ( 'NONE',  ( 56.81924384183006538, 46.80051614449766362, -4.924951120819380357 ) ) ;
#1113=CARTESIAN_POINT ( 'NONE',  ( 45.90387839640208512, 60.30051614449766362, -5.676469297603124353 ) ) ;
#1114=CARTESIAN_POINT ( 'NONE',  ( 48.02776887271745210, 61.39948385550240317, -5.992620115222778487 ) ) ;
#1126=CARTESIAN_POINT ( 'NONE',  ( 44.03140696652192787, 49.19948385550240033, -4.306917132069425058 ) ) ;
#1128=CARTESIAN_POINT ( 'NONE',  ( 43.69122665457040000, 50.00051614449765935, -0.02388180880515696977 ) ) ;
#1132=CARTESIAN_POINT ( 'NONE',  ( 52.25172492374522903, 59.59948385550240602, -7.007379884777225953 ) ) ;
#1147=CARTESIAN_POINT ( 'NONE',  ( 56.65037692655918988, 53.89948385550240317, -2.184720259617163762 ) ) ;
#1150=CARTESIAN_POINT ( 'NONE',  ( 52.29715082351538769, 44.60051614449766788, -6.992620115222796251 ) ) ;
#1152=CARTESIAN_POINT ( 'NONE',  ( 47.37792948025162332, 63.39948385550238896, -7.992620115222770494 ) ) ;
#1154=CARTESIAN_POINT ( 'NONE',  ( 45.31609314410967926, 58.69948385550240033, 6.485486291978119766 ) ) ;
#1157=ORIENTED_EDGE ( 'NONE', *, *, #10798, .T. ) ;
#1164=CARTESIAN_POINT ( 'NONE',  ( 48.07319477248762496, 48.40051614449766504, -6.007379884777208190 ) ) ;
#1165=CARTESIAN_POINT ( 'NONE',  ( 45.86712807150329496, 61.70051614449766220, 5.649768623646139964 ) ) ;
#1166=CARTESIAN_POINT ( 'NONE',  ( 47.37792948025162332, 47.39948385550241028, -7.992620115222770494 ) ) ;
#1168=CARTESIAN_POINT ( 'NONE',  ( 50.02271294988505446, 58.50051614449765225, -8.000000000000001776 ) ) ;
#1178=CARTESIAN_POINT ( 'NONE',  ( 44.28664221472220675, 47.09948385550240602, -1.832500667257165317 ) ) ;
#1179=CARTESIAN_POINT ( 'NONE',  ( 50.02271294988512551, 62.49948385550240459, 7.000000000000000888 ) ) ;
#1180=CARTESIAN_POINT ( 'NONE',  ( 49.97728705011495265, 45.50051614449766646, 8.000000000000001776 ) ) ;
#1183=CARTESIAN_POINT ( 'NONE',  ( 47.70284917648459100, 55.60051614449764656, 6.992620115222796251 ) ) ;
#1184=CARTESIAN_POINT ( 'NONE',  ( 44.30067958973596376, 60.89948385550241028, 1.875703265242204099 ) ) ;
#1198=CARTESIAN_POINT ( 'NONE',  ( 44.05948171654949874, 50.79948385550238754, 4.345558710429105354 ) ) ;
#1202=CARTESIAN_POINT ( 'NONE',  ( 43.69122665457040000, 52.00051614449766646, -0.02388180880515696977 ) ) ;
#1206=CARTESIAN_POINT ( 'NONE',  ( 50.02271294988512551, 58.49948385550241170, 7.000000000000000888 ) ) ;
#1216=CARTESIAN_POINT ( 'NONE',  ( 47.70284917648453415, 55.39948385550239607, -6.992620115222774047 ) ) ;
#1217=CARTESIAN_POINT ( 'NONE',  ( 47.70284917648459100, 55.60051614449764656, 6.992620115222796251 ) ) ;
#1219=CARTESIAN_POINT ( 'NONE',  ( 56.66441430157296821, 46.09948385550240602, 2.141517661632100111 ) ) ;
#1221=CARTESIAN_POINT ( 'NONE',  ( 42.38452918213188525, 57.09948385550240602, -2.450534656007040013 ) ) ;
#1222=ORIENTED_EDGE ( 'NONE', *, *, #8044, .T. ) ;
#1228=CARTESIAN_POINT ( 'NONE',  ( 44.91013252490150620, 46.20051614449766220, -3.727524721679154940 ) ) ;
#1229=CARTESIAN_POINT ( 'NONE',  ( 50.02271294988505446, 64.50051614449765225, -7.000000000000000888 ) ) ;
#1230=CARTESIAN_POINT ( 'NONE',  ( 49.97728705011486738, 47.49948385550240459, -8.000000000000001776 ) ) ;
#1231=CARTESIAN_POINT ( 'NONE',  ( 52.62207051974829852, 56.60051614449765367, -7.992620115222797139 ) ) ;
#1240=CARTESIAN_POINT ( 'NONE',  ( 55.11794222512601493, 52.19948385550240744, 3.688883143319541702 ) ) ;
#1241=CARTESIAN_POINT ( 'NONE',  ( 43.33558569842703179, 65.09948385550239891, -2.141517661632099223 ) ) ;
#1242=CARTESIAN_POINT ( 'NONE',  ( 43.18075615816994173, 47.80051614449764941, 4.924951120819380357 ) ) ;
#1245=CARTESIAN_POINT ( 'NONE',  ( 47.74827507625469281, 58.40051614449766504, -7.007379884777203749 ) ) ;
#1246=CARTESIAN_POINT ( 'NONE',  ( 55.08986747509847248, 55.79948385550239465, -3.727524721679197572 ) ) ;
#1253=CARTESIAN_POINT ( 'NONE',  ( 49.97728705011488159, 49.49948385550240459, -7.000000000000000888 ) ) ;
#1256=CARTESIAN_POINT ( 'NONE',  ( 56.30877334542961421, 49.00051614449765935, 0.02388180880515774693 ) ) ;
#1261=CARTESIAN_POINT ( 'NONE',  ( 43.34962307344081012, 58.89948385550241028, 2.184720259617164650 ) ) ;
#1266=EDGE_CURVE ( 'NONE', #9956, #9726, #6857, .T. ) ;
#1275=CARTESIAN_POINT ( 'NONE',  ( 47.70284917648453415, 53.39948385550239607, -6.992620115222774047 ) ) ;
#1277=CARTESIAN_POINT ( 'NONE',  ( 54.13287192849671214, 54.70051614449766220, -5.649768623646139964 ) ) ;
#1280=CARTESIAN_POINT ( 'NONE',  ( 45.90387839640214196, 52.69948385550240033, 5.676469297603166098 ) ) ;
#1284=CARTESIAN_POINT ( 'NONE',  ( 42.39856655714566358, 64.89948385550239607, 2.493737253992119207 ) ) ;
#1292=CARTESIAN_POINT ( 'NONE',  ( 55.08986747509849380, 53.20051614449766220, 3.727524721679155384 ) ) ;
#1295=CARTESIAN_POINT ( 'NONE',  ( 42.39856655714566358, 50.89948385550240317, 2.493737253992119207 ) ) ;
#1297=CARTESIAN_POINT ( 'NONE',  ( 52.29715082351547295, 54.39948385550239607, 6.992620115222774047 ) ) ;
#1299=CARTESIAN_POINT ( 'NONE',  ( 43.18075615816994173, 55.80051614449766362, 4.924951120819380357 ) ) ;
#1309=CARTESIAN_POINT ( 'NONE',  ( 51.92680522751233951, 53.59948385550240602, -6.007379884777223289 ) ) ;
#1310=CARTESIAN_POINT ( 'NONE',  ( 42.63976443033212149, 46.00051614449765225, -0.02388180880514948964 ) ) ;
#1311=CARTESIAN_POINT ( 'NONE',  ( 47.42335538002180328, 46.40051614449765793, -8.007379884777206414 ) ) ;
#1314=CARTESIAN_POINT ( 'NONE',  ( 52.29715082351538769, 58.60051614449766078, -6.992620115222796251 ) ) ;
#1316=CARTESIAN_POINT ( 'NONE',  ( 48.07319477248768180, 62.59948385550238470, 6.007379884777225953 ) ) ;
#1325=CARTESIAN_POINT ( 'NONE',  ( 44.03140696652192787, 51.19948385550238612, -4.306917132069425058 ) ) ;
#1327=CARTESIAN_POINT ( 'NONE',  ( 43.69122665457040000, 58.00051614449765935, -0.02388180880515696977 ) ) ;
#1332=CARTESIAN_POINT ( 'NONE',  ( 48.02776887271745210, 47.39948385550241028, -5.992620115222778487 ) ) ;
#1345=CARTESIAN_POINT ( 'NONE',  ( 57.36023556966787851, 51.99948385550239749, -0.02388180880522424582 ) ) ;
#1347=CARTESIAN_POINT ( 'NONE',  ( 43.33558569842706021, 55.90051614449765793, 2.141517661632167169 ) ) ;
#1352=CARTESIAN_POINT ( 'NONE',  ( 42.63976443033212860, 52.99948385550240459, 0.02388180880522514787 ) ) ;
#1354=CARTESIAN_POINT ( 'NONE',  ( 47.37792948025162332, 65.39948385550239607, -7.992620115222770494 ) ) ;
#1361=CARTESIAN_POINT ( 'NONE',  ( 48.07319477248762496, 52.40051614449767214, -6.007379884777208190 ) ) ;
#1364=CARTESIAN_POINT ( 'NONE',  ( 47.37792948025162332, 55.39948385550240317, -7.992620115222770494 ) ) ;
#1365=CARTESIAN_POINT ( 'NONE',  ( 56.66441430157296821, 56.09948385550240602, 2.141517661632100111 ) ) ;
#1367=CARTESIAN_POINT ( 'NONE',  ( 42.38452918213190657, 63.90051614449765793, 2.450534656007115508 ) ) ;
#1378=CARTESIAN_POINT ( 'NONE',  ( 46.49166364869460466, 58.69948385550240033, 4.867452303228209765 ) ) ;
#1379=CARTESIAN_POINT ( 'NONE',  ( 52.25172492374528588, 45.40051614449766504, 7.007379884777204637 ) ) ;
#1380=CARTESIAN_POINT ( 'NONE',  ( 52.62207051974829852, 50.60051614449765367, -7.992620115222797139 ) ) ;
#1383=CARTESIAN_POINT ( 'NONE',  ( 45.27934281921082516, 45.70051614449766220, 6.458785618021089192 ) ) ;
#1391=CARTESIAN_POINT ( 'NONE',  ( 47.70284917648453415, 55.39948385550238896, -6.992620115222774047 ) ) ;
#1393=CARTESIAN_POINT ( 'NONE',  ( 53.50833635130544508, 55.30051614449765651, 4.867452303228181343 ) ) ;
#1398=CARTESIAN_POINT ( 'NONE',  ( 52.29715082351547295, 64.39948385550239607, 6.992620115222774047 ) ) ;
#1415=CARTESIAN_POINT ( 'NONE',  ( 57.36023556966787851, 51.00051614449763804, 0.02388180880515038476 ) ) ;
#1417=CARTESIAN_POINT ( 'NONE',  ( 54.09612160359786515, 51.69948385550240744, -5.676469297603166098 ) ) ;
#1418=CARTESIAN_POINT ( 'NONE',  ( 45.90387839640214196, 46.69948385550240744, 5.676469297603166098 ) ) ;
#1420=CARTESIAN_POINT ( 'NONE',  ( 55.94051828345050836, 45.79948385550240886, -4.345558710429104465 ) ) ;
#1422=EDGE_LOOP ( 'NONE', ( #5240, #8901, #12422, #11501, #9871, #1222 ) ) ;
#1428=CARTESIAN_POINT ( 'NONE',  ( 56.30877334542961421, 53.00051614449765935, 0.02388180880515774693 ) ) ;
#1430=CARTESIAN_POINT ( 'NONE',  ( 57.60143344285433642, 55.89948385550241028, -2.493737253992118319 ) ) ;
#1431=CARTESIAN_POINT ( 'NONE',  ( 43.34962307344081012, 54.89948385550240317, 2.184720259617164650 ) ) ;
#1433=CARTESIAN_POINT ( 'NONE',  ( 41.58830220609386430, 64.00051614449765225, -0.02388180880514929535 ) ) ;
#1447=CARTESIAN_POINT ( 'NONE',  ( 48.07319477248768180, 58.59948385550239891, 6.007379884777225953 ) ) ;
#1448=CARTESIAN_POINT ( 'NONE',  ( 54.13287192849671214, 46.70051614449766220, -5.649768623646139964 ) ) ;
#1450=CARTESIAN_POINT ( 'NONE',  ( 42.38452918213190657, 55.90051614449766504, 2.450534656007115508 ) ) ;
#1454=CARTESIAN_POINT ( 'NONE',  ( 42.38452918213190657, 45.90051614449766504, 2.450534656007115508 ) ) ;
#1463=CARTESIAN_POINT ( 'NONE',  ( 54.09612160359786515, 59.69948385550240033, -5.676469297603166098 ) ) ;
#1465=CARTESIAN_POINT ( 'NONE',  ( 44.88205777487401349, 59.80051614449766362, 3.688883143319584779 ) ) ;
#1468=CARTESIAN_POINT ( 'NONE',  ( 56.66441430157294690, 46.90051614449765793, -2.141517661632166281 ) ) ;
#1469=CARTESIAN_POINT ( 'NONE',  ( 50.02271294988511841, 48.49948385550241170, 6.000000000000000888 ) ) ;
#1476=CARTESIAN_POINT ( 'NONE',  ( 54.89903213687075834, 44.74560054925188268, -5.000000000000007105 ) ) ;
#1480=CARTESIAN_POINT ( 'NONE',  ( 52.25172492374527877, 55.40051614449764372, 7.007379884777203749 ) ) ;
#1482=CARTESIAN_POINT ( 'NONE',  ( 57.36023556966787851, 53.99948385550239038, -0.02388180880522424582 ) ) ;
#1483=CARTESIAN_POINT ( 'NONE',  ( 54.13287192849676188, 48.29948385550240175, 5.649768623646098220 ) ) ;
#1485=CARTESIAN_POINT ( 'NONE',  ( 42.38452918213188525, 65.09948385550239891, -2.450534656007040013 ) ) ;
#1495=CARTESIAN_POINT ( 'NONE',  ( 53.50833635130544508, 57.30051614449767072, 4.867452303228181343 ) ) ;
#1497=CARTESIAN_POINT ( 'NONE',  ( 57.61547081786812896, 54.09948385550241312, 2.450534656007040901 ) ) ;
#1498=CARTESIAN_POINT ( 'NONE',  ( 44.05948171654949874, 58.79948385550240886, 4.345558710429105354 ) ) ;
#1501=CARTESIAN_POINT ( 'NONE',  ( 47.37792948025170858, 61.60051614449765367, 7.992620115222797139 ) ) ;
#1505=AXIS2_PLACEMENT_3D ( 'NONE', #10752, #2313, #13087 ) ;
#1517=CARTESIAN_POINT ( 'NONE',  ( 55.71335778527780747, 54.09948385550241312, 1.832500667257165983 ) ) ;
#1518=CARTESIAN_POINT ( 'NONE',  ( 43.33558569842706021, 47.90051614449765793, 2.141517661632167169 ) ) ;
#1520=CARTESIAN_POINT ( 'NONE',  ( 45.31609314410960820, 54.30051614449765651, -6.485486291978072693 ) ) ;
#1524=CARTESIAN_POINT ( 'NONE',  ( 42.63976443033212860, 62.00051614449764514, -0.02388180880514948964 ) ) ;
#1533=CARTESIAN_POINT ( 'NONE',  ( 45.86712807150323812, 59.29948385550240175, -5.649768623646098220 ) ) ;
#1535=CARTESIAN_POINT ( 'NONE',  ( 51.92680522751238925, 61.40051614449765793, 6.007379884777208190 ) ) ;
#1538=CARTESIAN_POINT ( 'NONE',  ( 55.94051828345053679, 47.20051614449766220, 4.345558710429044069 ) ) ;
#1539=CARTESIAN_POINT ( 'NONE',  ( 55.96859303347804371, 64.19948385550239323, 4.306917132069425946 ) ) ;
#1550=CARTESIAN_POINT ( 'NONE',  ( 43.33558569842706021, 61.90051614449766504, 2.141517661632167169 ) ) ;
#1553=CARTESIAN_POINT ( 'NONE',  ( 47.74827507625478518, 52.59948385550239180, 7.007379884777227730 ) ) ;
#1554=CARTESIAN_POINT ( 'NONE',  ( 54.09612160359786515, 45.69948385550240744, -5.676469297603166098 ) ) ;
#1556=CARTESIAN_POINT ( 'NONE',  ( 43.20883090819745576, 62.79948385550240175, 4.963592699179006473 ) ) ;
#1563=AXIS2_PLACEMENT_3D ( 'NONE', #6311, #8038, #3749 ) ;
#1566=CARTESIAN_POINT ( 'NONE',  ( 55.71335778527780036, 54.90051614449765793, -1.832500667257213056 ) ) ;
#1568=CARTESIAN_POINT ( 'NONE',  ( 43.20883090819745576, 52.79948385550240175, 4.963592699179006473 ) ) ;
#1569=CARTESIAN_POINT ( 'NONE',  ( 42.63976443033212860, 54.99948385550241170, 0.02388180880522514787 ) ) ;
#1571=CARTESIAN_POINT ( 'NONE',  ( 47.42335538002188144, 46.59948385550239891, 8.007379884777233059 ) ) ;
#1584=CARTESIAN_POINT ( 'NONE',  ( 43.69122665457040000, 58.99948385550239749, 0.02388180880521036456 ) ) ;
#1585=CARTESIAN_POINT ( 'NONE',  ( 56.66441430157294690, 48.90051614449766504, -2.141517661632166281 ) ) ;
#1586=CARTESIAN_POINT ( 'NONE',  ( 45.27934281921082516, 53.70051614449766220, 6.458785618021089192 ) ) ;
#1590=CARTESIAN_POINT ( 'NONE',  ( 55.96859303347802239, 60.80051614449764941, -4.306917132069484566 ) ) ;
#1599=CARTESIAN_POINT ( 'NONE',  ( 45.86712807150323812, 57.29948385550240175, -5.649768623646098220 ) ) ;
#1600=CARTESIAN_POINT ( 'NONE',  ( 54.13287192849676188, 52.29948385550240886, 5.649768623646098220 ) ) ;
#1601=CARTESIAN_POINT ( 'NONE',  ( 44.88205777487401349, 57.80051614449766362, 3.688883143319584779 ) ) ;
#1604=CARTESIAN_POINT ( 'NONE',  ( 51.92680522751238925, 63.40051614449765083, 6.007379884777208190 ) ) ;
#1605=CARTESIAN_POINT ( 'NONE',  ( 51.97223112728254790, 46.39948385550240317, 5.992620115222778487 ) ) ;
#1616=SURFACE_STYLE_FILL_AREA ( #7027 ) ;
#1621=CARTESIAN_POINT ( 'NONE',  ( 56.65037692655921120, 61.10051614449766078, 2.184720259617097593 ) ) ;
#1625=CARTESIAN_POINT ( 'NONE',  ( 54.09612160359786515, 59.69948385550240033, -5.676469297603166098 ) ) ;
#1626=CARTESIAN_POINT ( 'NONE',  ( 44.03140696652192787, 49.19948385550240033, -4.306917132069425058 ) ) ;
#1627=CARTESIAN_POINT ( 'NONE',  ( 52.25172492374522903, 51.59948385550240602, -7.007379884777225953 ) ) ;
#1636=CARTESIAN_POINT ( 'NONE',  ( 44.91013252490150620, 60.20051614449766220, -3.727524721679154940 ) ) ;
#1639=CARTESIAN_POINT ( 'NONE',  ( 52.62207051974839089, 58.39948385550241028, 7.992620115222770494 ) ) ;
#1641=CARTESIAN_POINT ( 'NONE',  ( 43.34962307344081012, 60.89948385550241028, 2.184720259617164650 ) ) ;
#1643=CARTESIAN_POINT ( 'NONE',  ( 56.79116909180259398, 63.20051614449766220, 4.963592699178938972 ) ) ;
#1655=CARTESIAN_POINT ( 'NONE',  ( 46.49166364869460466, 62.69948385550240744, 4.867452303228209765 ) ) ;
#1656=CARTESIAN_POINT ( 'NONE',  ( 57.36023556966787851, 53.00051614449765225, 0.02388180880515038476 ) ) ;
#1657=CARTESIAN_POINT ( 'NONE',  ( 42.38452918213190657, 53.90051614449765793, 2.450534656007115508 ) ) ;
#1660=CARTESIAN_POINT ( 'NONE',  ( 43.34962307344078880, 64.10051614449766078, -2.184720259617096705 ) ) ;
#1670=CARTESIAN_POINT ( 'NONE',  ( 55.94051828345050836, 59.79948385550238754, -4.345558710429104465 ) ) ;
#1671=CARTESIAN_POINT ( 'NONE',  ( 43.34962307344081012, 58.89948385550241028, 2.184720259617164650 ) ) ;
#1676=CARTESIAN_POINT ( 'NONE',  ( 54.13287192849671214, 46.70051614449766220, -5.649768623646139964 ) ) ;
#1677=CARTESIAN_POINT ( 'NONE',  ( 55.08986747509847248, 53.79948385550241596, -3.727524721679197572 ) ) ;
#1690=CARTESIAN_POINT ( 'NONE',  ( 52.25172492374527877, 57.40051614449765083, 7.007379884777203749 ) ) ;
#1692=CARTESIAN_POINT ( 'NONE',  ( 53.50833635130540955, 63.69948385550240033, -4.867452303228209765 ) ) ;
#1695=CARTESIAN_POINT ( 'NONE',  ( 43.33558569842703179, 59.09948385550240602, -2.141517661632099223 ) ) ;
#1696=CARTESIAN_POINT ( 'NONE',  ( 47.70284917648453415, 47.39948385550238896, -6.992620115222774047 ) ) ;
#1698=CARTESIAN_POINT ( 'NONE',  ( 43.33558569842703179, 47.09948385550240602, -2.141517661632099223 ) ) ;
#1706=CARTESIAN_POINT ( 'NONE',  ( 44.91013252490150620, 64.20051614449766930, -3.727524721679154940 ) ) ;
#1709=CARTESIAN_POINT ( 'NONE',  ( 45.31609314410967926, 56.69948385550240744, 6.485486291978119766 ) ) ;
#1713=CARTESIAN_POINT ( 'NONE',  ( 45.27934281921075410, 49.29948385550240886, -6.458785618021043895 ) ) ;
#1725=CARTESIAN_POINT ( 'NONE',  ( 48.02776887271745210, 65.39948385550239607, -5.992620115222778487 ) ) ;
#1726=CARTESIAN_POINT ( 'NONE',  ( 52.29715082351539479, 52.60051614449766078, -6.992620115222796251 ) ) ;
#1727=CARTESIAN_POINT ( 'NONE',  ( 45.31609314410960820, 56.30051614449766362, -6.485486291978072693 ) ) ;
#1732=CARTESIAN_POINT ( 'NONE',  ( 42.39856655714564226, 48.10051614449766078, -2.493737253992044156 ) ) ;
#1742=CARTESIAN_POINT ( 'NONE',  ( 51.92680522751233951, 45.59948385550240602, -6.007379884777223289 ) ) ;
#1743=CARTESIAN_POINT ( 'NONE',  ( 44.03140696652193498, 59.19948385550240033, -4.306917132069424170 ) ) ;
#1748=CARTESIAN_POINT ( 'NONE',  ( 54.13287192849671214, 44.70051614449766220, -5.649768623646139964 ) ) ;
#1749=CARTESIAN_POINT ( 'NONE',  ( 46.49166364869460466, 50.69948385550240744, 4.867452303228209765 ) ) ;
#1753=EDGE_CURVE ( 'NONE', #3958, #5739, #10479, .T. ) ;
#1761=CARTESIAN_POINT ( 'NONE',  ( 56.66441430157296821, 46.09948385550240602, 2.141517661632100111 ) ) ;
#1764=CARTESIAN_POINT ( 'NONE',  ( 55.11794222512601493, 64.19948385550240744, 3.688883143319541702 ) ) ;
#1766=CARTESIAN_POINT ( 'NONE',  ( 52.25172492374522903, 59.59948385550240602, -7.007379884777225953 ) ) ;
#1767=CARTESIAN_POINT ( 'NONE',  ( 45.86712807150323812, 55.29948385550240175, -5.649768623646098220 ) ) ;
#1769=CARTESIAN_POINT ( 'NONE',  ( 57.36023556966787851, 49.99948385550238328, -0.02388180880522424582 ) ) ;
#1781=CARTESIAN_POINT ( 'NONE',  ( 56.30877334542961421, 61.00051614449765935, 0.02388180880515774693 ) ) ;
#1783=CARTESIAN_POINT ( 'NONE',  ( 43.20883090819745576, 58.79948385550240175, 4.963592699179006473 ) ) ;
#1784=CARTESIAN_POINT ( 'NONE',  ( 44.05948171654949874, 60.79948385550240886, 4.345558710429105354 ) ) ;
#1786=CARTESIAN_POINT ( 'NONE',  ( 50.02271294988513972, 48.49948385550241170, 8.000000000000001776 ) ) ;
#1795=CARTESIAN_POINT ( 'NONE',  ( 49.99999999999997158, 45.00000000000003553, -7.000000000000000888 ) ) ;
#1797=CARTESIAN_POINT ( 'NONE',  ( 50.02271294988511841, 62.49948385550240459, 6.000000000000000888 ) ) ;
#1799=CARTESIAN_POINT ( 'NONE',  ( 43.34962307344078880, 56.10051614449766078, -2.184720259617096705 ) ) ;
#1800=CARTESIAN_POINT ( 'NONE',  ( 45.27934281921082516, 59.70051614449766220, 6.458785618021089192 ) ) ;
#1805=CARTESIAN_POINT ( 'NONE',  ( 43.18075615816994173, 49.80051614449765651, 4.924951120819380357 ) ) ;
#1807=ORIENTED_EDGE ( 'NONE', *, *, #4185, .F. ) ;
#1816=CARTESIAN_POINT ( 'NONE',  ( 47.70284917648453415, 65.39948385550239607, -6.992620115222774047 ) ) ;
#1817=CARTESIAN_POINT ( 'NONE',  ( 50.02271294988512551, 56.49948385550240459, 7.000000000000000888 ) ) ;
#1821=CARTESIAN_POINT ( 'NONE',  ( 54.09612160359792199, 53.30051614449766362, 5.676469297603124353 ) ) ;
#1822=CARTESIAN_POINT ( 'NONE',  ( 53.54508667620428497, 54.29948385550241596, 4.840751629271157874 ) ) ;
#1832=CARTESIAN_POINT ( 'NONE',  ( 45.90387839640214196, 46.69948385550240744, 5.676469297603166098 ) ) ;
#1835=CARTESIAN_POINT ( 'NONE',  ( 48.07319477248768180, 64.59948385550241312, 6.007379884777225953 ) ) ;
#1837=CARTESIAN_POINT ( 'NONE',  ( 54.13287192849676188, 58.29948385550240175, 5.649768623646098220 ) ) ;
#1838=CARTESIAN_POINT ( 'NONE',  ( 52.29715082351547295, 54.39948385550239607, 6.992620115222774047 ) ) ;
#1841=CARTESIAN_POINT ( 'NONE',  ( 56.66441430157296821, 52.09948385550240602, 2.141517661632100111 ) ) ;
#1850=CARTESIAN_POINT ( 'NONE',  ( 55.71335778527780036, 62.90051614449765083, -1.832500667257213056 ) ) ;
#1852=CARTESIAN_POINT ( 'NONE',  ( 58.41169779390614281, 57.99948385550241170, -0.02388180880523160798 ) ) ;
#1853=CARTESIAN_POINT ( 'NONE',  ( 47.74827507625478518, 60.59948385550239891, 7.007379884777227730 ) ) ;
#1856=CARTESIAN_POINT ( 'NONE',  ( 42.38452918213188525, 49.09948385550241312, -2.450534656007040013 ) ) ;
#1864=CARTESIAN_POINT ( 'NONE',  ( 54.77701766759913227, 44.74161735293615294, -5.000000000000010658 ) ) ;
#1870=CARTESIAN_POINT ( 'NONE',  ( 44.28664221472220675, 65.09948385550239891, -1.832500667257165317 ) ) ;
#1871=CARTESIAN_POINT ( 'NONE',  ( 56.66441430157294690, 54.90051614449765793, -2.141517661632166281 ) ) ;
#1873=CARTESIAN_POINT ( 'NONE',  ( 56.79116909180259398, 61.20051614449766220, 4.963592699178938972 ) ) ;
#1876=CARTESIAN_POINT ( 'NONE',  ( 52.62207051974829852, 48.60051614449766788, -7.992620115222797139 ) ) ;
#1887=CARTESIAN_POINT ( 'NONE',  ( 44.03140696652192787, 61.19948385550239323, -4.306917132069425058 ) ) ;
#1888=CARTESIAN_POINT ( 'NONE',  ( 44.03140696652193498, 61.19948385550240033, -4.306917132069424170 ) ) ;
#1891=CARTESIAN_POINT ( 'NONE',  ( 53.49409602498213445, 45.00000000000000711, -6.629536405711814240 ) ) ;
#1892=CARTESIAN_POINT ( 'NONE',  ( 44.05948171654945611, 48.20051614449764799, -4.345558710429044069 ) ) ;
#1893=CARTESIAN_POINT ( 'NONE',  ( 51.92680522751233951, 55.59948385550240602, -6.007379884777223289 ) ) ;
#1908=CARTESIAN_POINT ( 'NONE',  ( 43.69122665457040000, 46.00051614449764514, -0.02388180880515696977 ) ) ;
#1910=CARTESIAN_POINT ( 'NONE',  ( 52.25172492374522903, 57.59948385550241312, -7.007379884777225953 ) ) ;
#1911=CARTESIAN_POINT ( 'NONE',  ( 54.09612160359786515, 55.69948385550240744, -5.676469297603166098 ) ) ;
#1913=CARTESIAN_POINT ( 'NONE',  ( 43.33558569842703179, 49.09948385550240602, -2.141517661632099223 ) ) ;
#1921=CARTESIAN_POINT ( 'NONE',  ( 46.45491332379576477, 63.70051614449766930, 4.840751629271188961 ) ) ;
#1923=CARTESIAN_POINT ( 'NONE',  ( 47.37792948025162332, 57.39948385550241028, -7.992620115222770494 ) ) ;
#1925=CARTESIAN_POINT ( 'NONE',  ( 56.81924384183011512, 52.19948385550240744, 4.924951120819313743 ) ) ;
#1935=CARTESIAN_POINT ( 'NONE',  ( 53.54508667620428497, 64.29948385550240175, 4.840751629271157874 ) ) ;
#1936=CARTESIAN_POINT ( 'NONE',  ( 52.25172492374528588, 53.40051614449765083, 7.007379884777204637 ) ) ;
#1938=CARTESIAN_POINT ( 'NONE',  ( 41.58830220609386430, 62.00051614449766646, -0.02388180880514929535 ) ) ;
#1940=CARTESIAN_POINT ( 'NONE',  ( 45.31609314410960820, 52.30051614449766362, -6.485486291978072693 ) ) ;
#1954=CARTESIAN_POINT ( 'NONE',  ( 49.97728705011488159, 63.49948385550241170, -7.000000000000000888 ) ) ;
#1956=CARTESIAN_POINT ( 'NONE',  ( 45.86712807150323812, 57.29948385550240175, -5.649768623646098220 ) ) ;
#1957=CARTESIAN_POINT ( 'NONE',  ( 43.34962307344078880, 60.10051614449766078, -2.184720259617096705 ) ) ;
#1961=CARTESIAN_POINT ( 'NONE',  ( 55.13865474201621453, 45.00000000000007816, -5.383573523308436748 ) ) ;
#1962=CARTESIAN_POINT ( 'NONE',  ( 43.33558569842706021, 51.90051614449765793, 2.141517661632167169 ) ) ;
#1963=CARTESIAN_POINT ( 'NONE',  ( 44.30067958973596376, 54.89948385550240317, 1.875703265242204099 ) ) ;
#1978=CARTESIAN_POINT ( 'NONE',  ( 44.30067958973594955, 48.10051614449766078, -1.875703265242155693 ) ) ;
#1980=CARTESIAN_POINT ( 'NONE',  ( 52.25172492374522903, 63.59948385550237759, -7.007379884777225953 ) ) ;
#1981=CARTESIAN_POINT ( 'NONE',  ( 56.66441430157296821, 54.09948385550240602, 2.141517661632100111 ) ) ;
#1984=CARTESIAN_POINT ( 'NONE',  ( 44.03140696652192787, 53.19948385550238612, -4.306917132069425058 ) ) ;
#1994=CARTESIAN_POINT ( 'NONE',  ( 42.63976443033212860, 48.00051614449766646, -0.02388180880514948964 ) ) ;
#1996=CARTESIAN_POINT ( 'NONE',  ( 44.05948171654949874, 48.79948385550238754, 4.345558710429105354 ) ) ;
#2000=CARTESIAN_POINT ( 'NONE',  ( 47.37792948025162332, 49.39948385550241028, -7.992620115222770494 ) ) ;
#2009=CARTESIAN_POINT ( 'NONE',  ( 51.92680522751238925, 51.40051614449767214, 6.007379884777208190 ) ) ;
#2010=CARTESIAN_POINT ( 'NONE',  ( 55.96859303347802239, 56.80051614449764941, -4.306917132069484566 ) ) ;
#2011=CARTESIAN_POINT ( 'NONE',  ( 57.61547081786810764, 60.90051614449766504, -2.450534656007114176 ) ) ;
#2012=CARTESIAN_POINT ( 'NONE',  ( 54.72065718078918906, 48.70051614449766930, -6.458785618021089192 ) ) ;
#2020=DIRECTION ( 'NONE',  ( 0.9989677110047502362, 0.04542589977017699732, -6.931730960091013400E-15 ) ) ;
#2024=CARTESIAN_POINT ( 'NONE',  ( 44.30067958973596376, 52.89948385550241028, 1.875703265242204099 ) ) ;
#2028=CARTESIAN_POINT ( 'NONE',  ( 44.05948171654945611, 58.20051614449764799, -4.345558710429044069 ) ) ;
#2032=CARTESIAN_POINT ( 'NONE',  ( 47.74827507625469281, 48.40051614449764372, -7.007379884777203749 ) ) ;
#2033=CARTESIAN_POINT ( 'NONE',  ( 55.71335778527780747, 62.09948385550240602, 1.832500667257165983 ) ) ;
#2045=CARTESIAN_POINT ( 'NONE',  ( 55.69932041026405045, 53.10051614449767499, 1.875703265242156359 ) ) ;
#2047=CARTESIAN_POINT ( 'NONE',  ( 54.09612160359786515, 63.69948385550240744, -5.676469297603166098 ) ) ;
#2048=CARTESIAN_POINT ( 'NONE',  ( 57.36023556966787851, 55.99948385550239038, -0.02388180880522424582 ) ) ;
#2060=CARTESIAN_POINT ( 'NONE',  ( 52.29715082351547295, 48.39948385550240317, 6.992620115222774047 ) ) ;
#2062=CARTESIAN_POINT ( 'NONE',  ( 45.86712807150329496, 47.70051614449766220, 5.649768623646139964 ) ) ;
#2064=CARTESIAN_POINT ( 'NONE',  ( 45.86712807150323812, 47.29948385550240886, -5.649768623646098220 ) ) ;
#2066=CARTESIAN_POINT ( 'NONE',  ( 47.37792948025162332, 55.39948385550240317, -7.992620115222770494 ) ) ;
#2073=CARTESIAN_POINT ( 'NONE',  ( 53.54508667620424234, 50.70051614449766220, -4.840751629271188961 ) ) ;
#2074=CARTESIAN_POINT ( 'NONE',  ( 50.02271294988505446, 58.50051614449765935, -7.000000000000000888 ) ) ;
#2076=CARTESIAN_POINT ( 'NONE',  ( 43.20883090819742023, 64.20051614449766930, -4.963592699178938972 ) ) ;
#2079=CARTESIAN_POINT ( 'NONE',  ( 42.39856655714564226, 56.10051614449766078, -2.493737253992044156 ) ) ;
#2090=CARTESIAN_POINT ( 'NONE',  ( 44.30067958973596376, 48.89948385550241028, 1.875703265242204099 ) ) ;
#2092=CARTESIAN_POINT ( 'NONE',  ( 56.79116909180259398, 47.20051614449766220, 4.963592699178938972 ) ) ;
#2096=CARTESIAN_POINT ( 'NONE',  ( 56.65037692655921120, 53.10051614449766078, 2.184720259617097593 ) ) ;
#2097=CARTESIAN_POINT ( 'NONE',  ( 46.49166364869460466, 58.69948385550240033, 4.867452303228209765 ) ) ;
#2106=CARTESIAN_POINT ( 'NONE',  ( 47.74827507625478518, 50.59948385550238470, 7.007379884777227730 ) ) ;
#2108=CARTESIAN_POINT ( 'NONE',  ( 55.11794222512599362, 48.80051614449767072, -3.688883143319583446 ) ) ;
#2112=CARTESIAN_POINT ( 'NONE',  ( 47.74827507625478518, 62.59948385550240602, 7.007379884777227730 ) ) ;
#2113=CARTESIAN_POINT ( 'NONE',  ( 55.96859303347804371, 62.19948385550240744, 4.306917132069425946 ) ) ;
#2121=DIRECTION ( 'NONE',  ( -0.9989677110047502362, -0.04542589977017699732, 6.931730960091013400E-15 ) ) ;
#2123=CARTESIAN_POINT ( 'NONE',  ( 43.33558569842703179, 47.09948385550240602, -2.141517661632099223 ) ) ;
#2125=CARTESIAN_POINT ( 'NONE',  ( 54.09612160359792199, 45.30051614449766362, 5.676469297603124353 ) ) ;
#2128=CARTESIAN_POINT ( 'NONE',  ( 50.02271294988513972, 64.49948385550239038, 8.000000000000001776 ) ) ;
#2131=CARTESIAN_POINT ( 'NONE',  ( 56.81924384183011512, 58.19948385550240744, 4.924951120819313743 ) ) ;
#2133=ORIENTED_EDGE ( 'NONE', *, *, #1753, .F. ) ;
#2138=CARTESIAN_POINT ( 'NONE',  ( 53.50833635130544508, 47.30051614449766362, 4.867452303228181343 ) ) ;
#2140=CARTESIAN_POINT ( 'NONE',  ( 43.34962307344078880, 58.10051614449766078, -2.184720259617096705 ) ) ;
#2141=CARTESIAN_POINT ( 'NONE',  ( 54.68390685589033495, 49.69948385550240744, -6.485486291978119766 ) ) ;
#2143=CARTESIAN_POINT ( 'NONE',  ( 49.97728705011495265, 55.50051614449766646, 8.000000000000001776 ) ) ;
#2153=CARTESIAN_POINT ( 'NONE',  ( 43.69122665457040000, 46.99948385550239749, 0.02388180880521036456 ) ) ;
#2155=CARTESIAN_POINT ( 'NONE',  ( 55.96859303347805081, 64.19948385550239323, 4.306917132069425058 ) ) ;
#2156=CARTESIAN_POINT ( 'NONE',  ( 52.62207051974829852, 46.60051614449764656, -7.992620115222797139 ) ) ;
#2160=CARTESIAN_POINT ( 'NONE',  ( 56.66441430157294690, 58.90051614449766504, -2.141517661632166281 ) ) ;
#2161=CARTESIAN_POINT ( 'NONE',  ( 43.69122665457040000, 60.99948385550241170, 0.02388180880521036456 ) ) ;
#2162=CARTESIAN_POINT ( 'NONE',  ( 55.41777406314699306, 44.91366546079681399, -4.999999999999999112 ) ) ;
#2172=CARTESIAN_POINT ( 'NONE',  ( 56.65037692655918988, 53.89948385550240317, -2.184720259617163762 ) ) ;
#2174=CARTESIAN_POINT ( 'NONE',  ( 55.71335778527780036, 50.90051614449765793, -1.832500667257213056 ) ) ;
#2176=CARTESIAN_POINT ( 'NONE',  ( 42.63976443033212860, 64.99948385550240459, 0.02388180880522514787 ) ) ;
#2178=CARTESIAN_POINT ( 'NONE',  ( 54.13287192849676188, 60.29948385550240886, 5.649768623646098220 ) ) ;
#2190=CARTESIAN_POINT ( 'NONE',  ( 45.90387839640214196, 52.69948385550240033, 5.676469297603166098 ) ) ;
#2191=CARTESIAN_POINT ( 'NONE',  ( 43.33558569842706021, 45.90051614449765793, 2.141517661632167169 ) ) ;
#2193=CARTESIAN_POINT ( 'NONE',  ( 50.02271294988512551, 46.49948385550240459, 7.000000000000000888 ) ) ;
#2196=CARTESIAN_POINT ( 'NONE',  ( 52.62207051974839089, 54.39948385550241028, 7.992620115222770494 ) ) ;
#2204=CARTESIAN_POINT ( 'NONE',  ( 51.97223112728249816, 46.60051614449764656, -5.992620115222793586 ) ) ;
#2205=CARTESIAN_POINT ( 'NONE',  ( 56.65037692655921120, 61.10051614449766078, 2.184720259617097593 ) ) ;
#2206=CARTESIAN_POINT ( 'NONE',  ( 56.81924384183006538, 62.80051614449766362, -4.924951120819380357 ) ) ;
#2208=CARTESIAN_POINT ( 'NONE',  ( 43.20883090819742023, 56.20051614449766220, -4.963592699178938972 ) ) ;
#2221=CARTESIAN_POINT ( 'NONE',  ( 43.69122665457040000, 50.99948385550241170, 0.02388180880521036456 ) ) ;
#2223=CARTESIAN_POINT ( 'NONE',  ( 50.02271294988505446, 64.50051614449765225, -7.000000000000000888 ) ) ;
#2227=CARTESIAN_POINT ( 'NONE',  ( 44.03140696652198471, 57.80051614449766362, 4.306917132069485454 ) ) ;
#2228=CARTESIAN_POINT ( 'NONE',  ( 48.07319477248768180, 58.59948385550239891, 6.007379884777225953 ) ) ;
#2238=CARTESIAN_POINT ( 'NONE',  ( 56.65037692655918988, 49.89948385550240317, -2.184720259617163762 ) ) ;
#2241=CARTESIAN_POINT ( 'NONE',  ( 56.30877334542961421, 51.00051614449765935, 0.02388180880515774693 ) ) ;
#2243=CARTESIAN_POINT ( 'NONE',  ( 44.05948171654949874, 64.79948385550240175, 4.345558710429105354 ) ) ;
#2244=CARTESIAN_POINT ( 'NONE',  ( 54.13287192849676188, 58.29948385550240175, 5.649768623646098220 ) ) ;
#2254=CARTESIAN_POINT ( 'NONE',  ( 47.74827507625477807, 54.59948385550239891, 7.007379884777229506 ) ) ;
#2256=CARTESIAN_POINT ( 'NONE',  ( 42.63976443033212860, 54.00051614449766646, -0.02388180880514948964 ) ) ;
#2259=CARTESIAN_POINT ( 'NONE',  ( 47.74827507625478518, 48.59948385550239180, 7.007379884777227730 ) ) ;
#2262=CARTESIAN_POINT ( 'NONE',  ( 54.72065718078924590, 54.29948385550241596, 6.458785618021043895 ) ) ;
#2269=CARTESIAN_POINT ( 'NONE',  ( 55.11794222512599362, 50.80051614449766362, -3.688883143319583446 ) ) ;
#2270=CARTESIAN_POINT ( 'NONE',  ( 45.90387839640208512, 62.30051614449766362, -5.676469297603124353 ) ) ;
#2272=CARTESIAN_POINT ( 'NONE',  ( 50.02271294988513972, 48.49948385550241170, 8.000000000000001776 ) ) ;
#2274=CARTESIAN_POINT ( 'NONE',  ( 52.57664461997821093, 53.40051614449765793, 8.007379884777206414 ) ) ;
#2287=CARTESIAN_POINT ( 'NONE',  ( 44.88205777487398507, 47.19948385550240744, -3.688883143319540814 ) ) ;
#2291=CARTESIAN_POINT ( 'NONE',  ( 45.86712807150329496, 63.70051614449766220, 5.649768623646139964 ) ) ;
#2296=CARTESIAN_POINT ( 'NONE',  ( 42.63976443033212860, 58.00051614449765225, -0.02388180880514948964 ) ) ;
#2297=CARTESIAN_POINT ( 'NONE',  ( 44.88205777487398507, 61.19948385550241454, -3.688883143319540814 ) ) ;
#2308=CARTESIAN_POINT ( 'NONE',  ( 56.66441430157296821, 48.09948385550240602, 2.141517661632100111 ) ) ;
#2311=CARTESIAN_POINT ( 'NONE',  ( 44.28664221472221385, 49.90051614449766504, 1.832500667257213722 ) ) ;
#2313=DIRECTION ( 'NONE',  ( 0.000000000000000000, 1.000000000000000000, 0.000000000000000000 ) ) ;
#2315=CARTESIAN_POINT ( 'NONE',  ( 55.94051828345050836, 61.79948385550239465, -4.345558710429104465 ) ) ;
#2325=CARTESIAN_POINT ( 'NONE',  ( 54.09612160359786515, 53.69948385550240744, -5.676469297603166098 ) ) ;
#2326=CARTESIAN_POINT ( 'NONE',  ( 45.90387839640208512, 54.30051614449765651, -5.676469297603124353 ) ) ;
#2329=CARTESIAN_POINT ( 'NONE',  ( 56.65037692655918988, 51.89948385550241028, -2.184720259617163762 ) ) ;
#2331=CARTESIAN_POINT ( 'NONE',  ( 47.37792948025162332, 59.39948385550240317, -7.992620115222770494 ) ) ;
#2338=CARTESIAN_POINT ( 'NONE',  ( 55.11794222512599362, 52.80051614449766362, -3.688883143319583446 ) ) ;
#2339=CARTESIAN_POINT ( 'NONE',  ( 43.34962307344078880, 64.10051614449766078, -2.184720259617096705 ) ) ;
#2340=CARTESIAN_POINT ( 'NONE',  ( 41.58830220609386430, 64.00051614449765225, -0.02388180880514929535 ) ) ;
#2341=CARTESIAN_POINT ( 'NONE',  ( 47.70284917648453415, 57.39948385550241028, -6.992620115222774047 ) ) ;
#2343=CARTESIAN_POINT ( 'NONE',  ( 56.79116909180259398, 55.20051614449766220, 4.963592699178938972 ) ) ;
#2355=CARTESIAN_POINT ( 'NONE',  ( 44.91013252490152752, 56.79948385550240175, 3.727524721679198461 ) ) ;
#2356=CARTESIAN_POINT ( 'NONE',  ( 52.25172492374528588, 49.40051614449766504, 7.007379884777204637 ) ) ;
#2357=CARTESIAN_POINT ( 'NONE',  ( 43.34962307344078880, 64.10051614449766078, -2.184720259617096705 ) ) ;
#2360=CARTESIAN_POINT ( 'NONE',  ( 54.09612160359792199, 57.30051614449765651, 5.676469297603124353 ) ) ;
#2361=CARTESIAN_POINT ( 'NONE',  ( 53.54508667620428497, 62.29948385550241596, 4.840751629271157874 ) ) ;
#2363=ORIENTED_EDGE ( 'NONE', *, *, #3106, .T. ) ;
#2372=CARTESIAN_POINT ( 'NONE',  ( 56.65037692655918988, 47.89948385550240317, -2.184720259617163762 ) ) ;
#2375=CARTESIAN_POINT ( 'NONE',  ( 48.02776887271750184, 57.60051614449765367, 5.992620115222795363 ) ) ;
#2379=CARTESIAN_POINT ( 'NONE',  ( 56.30877334542961421, 47.99948385550239038, -0.02388180880520959434 ) ) ;
#2390=CARTESIAN_POINT ( 'NONE',  ( 44.03140696652193498, 51.19948385550240033, -4.306917132069424170 ) ) ;
#2391=CARTESIAN_POINT ( 'NONE',  ( 42.63976443033212860, 52.00051614449766646, -0.02388180880514948964 ) ) ;
#2394=CARTESIAN_POINT ( 'NONE',  ( 44.05948171654949874, 52.79948385550240175, 4.345558710429105354 ) ) ;
#2398=CARTESIAN_POINT ( 'NONE',  ( 43.20883090819745576, 64.79948385550240175, 4.963592699179006473 ) ) ;
#2406=CARTESIAN_POINT ( 'NONE',  ( 44.88205777487401349, 55.80051614449766362, 3.688883143319584779 ) ) ;
#2407=CARTESIAN_POINT ( 'NONE',  ( 45.90387839640208512, 64.30051614449766362, -5.676469297603124353 ) ) ;
#2408=CARTESIAN_POINT ( 'NONE',  ( 42.38452918213188525, 55.09948385550241312, -2.450534656007040013 ) ) ;
#2410=CARTESIAN_POINT ( 'NONE',  ( 56.65037692655918988, 59.89948385550241028, -2.184720259617163762 ) ) ;
#2412=CARTESIAN_POINT ( 'NONE',  ( 42.39856655714566358, 46.89948385550240317, 2.493737253992119207 ) ) ;
#2424=CARTESIAN_POINT ( 'NONE',  ( 44.91013252490152752, 58.79948385550240175, 3.727524721679198461 ) ) ;
#2425=CARTESIAN_POINT ( 'NONE',  ( 42.63976443033212149, 50.00051614449765935, -0.02388180880514948964 ) ) ;
#2426=CARTESIAN_POINT ( 'NONE',  ( 42.39856655714564226, 52.10051614449766788, -2.493737253992044156 ) ) ;
#2430=CARTESIAN_POINT ( 'NONE',  ( 47.70284917648459100, 63.60051614449766078, 6.992620115222796251 ) ) ;
#2440=CARTESIAN_POINT ( 'NONE',  ( 56.66441430157296821, 60.09948385550240602, 2.141517661632100111 ) ) ;
#2442=CARTESIAN_POINT ( 'NONE',  ( 49.97728705011494554, 55.50051614449766646, 6.000000000000000888 ) ) ;
#2446=CARTESIAN_POINT ( 'NONE',  ( 57.36023556966787851, 63.99948385550241881, -0.02388180880522424582 ) ) ;
#2458=CARTESIAN_POINT ( 'NONE',  ( 44.05948171654949874, 54.79948385550240886, 4.345558710429104465 ) ) ;
#2460=CARTESIAN_POINT ( 'NONE',  ( 55.94051828345053679, 51.20051614449766220, 4.345558710429044069 ) ) ;
#2464=CARTESIAN_POINT ( 'NONE',  ( 56.65037692655918988, 53.89948385550240317, -2.184720259617163762 ) ) ;
#2466=CARTESIAN_POINT ( 'NONE',  ( 49.97728705011488159, 45.49948385550240459, -7.000000000000000888 ) ) ;
#2468=CARTESIAN_POINT ( 'NONE',  ( 52.57664461997811856, 63.59948385550239891, -8.007379884777229506 ) ) ;
#2478=CARTESIAN_POINT ( 'NONE',  ( 48.07319477248762496, 56.40051614449765793, -6.007379884777208190 ) ) ;
#2479=CARTESIAN_POINT ( 'NONE',  ( 42.63976443033212149, 64.00051614449765225, -0.02388180880514948964 ) ) ;
#2480=CARTESIAN_POINT ( 'NONE',  ( 45.31609314410967926, 54.69948385550240033, 6.485486291978119766 ) ) ;
#2482=CARTESIAN_POINT ( 'NONE',  ( 57.36023556966787851, 57.99948385550239038, -0.02388180880522424582 ) ) ;
#2484=CARTESIAN_POINT ( 'NONE',  ( 52.57664461997821093, 63.40051614449765083, 8.007379884777206414 ) ) ;
#2497=CARTESIAN_POINT ( 'NONE',  ( 55.69932041026404335, 57.89948385550241028, -1.875703265242203432 ) ) ;
#2498=CARTESIAN_POINT ( 'NONE',  ( 44.05948171654945611, 50.20051614449765509, -4.345558710429044069 ) ) ;
#2499=CARTESIAN_POINT ( 'NONE',  ( 43.20883090819742023, 50.20051614449766220, -4.963592699178938972 ) ) ;
#2502=CARTESIAN_POINT ( 'NONE',  ( 56.66441430157294690, 60.90051614449766504, -2.141517661632166281 ) ) ;
#2511=CARTESIAN_POINT ( 'NONE',  ( 50.02271294988512551, 58.49948385550241170, 7.000000000000000888 ) ) ;
#2512=CARTESIAN_POINT ( 'NONE',  ( 44.28664221472221385, 59.90051614449767214, 1.832500667257213722 ) ) ;
#2516=CARTESIAN_POINT ( 'NONE',  ( 48.02776887271750184, 61.60051614449765367, 5.992620115222795363 ) ) ;
#2517=CARTESIAN_POINT ( 'NONE',  ( 55.71335778527780747, 48.09948385550240602, 1.832500667257165983 ) ) ;
#2530=CARTESIAN_POINT ( 'NONE',  ( 45.86712807150329496, 55.70051614449766220, 5.649768623646139964 ) ) ;
#2532=CARTESIAN_POINT ( 'NONE',  ( 44.03140696652192787, 49.19948385550240033, -4.306917132069425058 ) ) ;
#2533=CARTESIAN_POINT ( 'NONE',  ( 43.34962307344081012, 46.89948385550240317, 2.184720259617164650 ) ) ;
#2535=CARTESIAN_POINT ( 'NONE',  ( 52.62207051974839089, 60.39948385550241028, 7.992620115222770494 ) ) ;
#2546=CARTESIAN_POINT ( 'NONE',  ( 50.02271294988506156, 54.50051614449765935, -6.000000000000000888 ) ) ;
#2549=CARTESIAN_POINT ( 'NONE',  ( 54.72065718078924590, 52.29948385550240886, 6.458785618021043895 ) ) ;
#2550=CARTESIAN_POINT ( 'NONE',  ( 45.90387839640214196, 54.69948385550240744, 5.676469297603166098 ) ) ;
#2552=CARTESIAN_POINT ( 'NONE',  ( 50.02271294988505446, 64.50051614449766646, -8.000000000000001776 ) ) ;
#2565=CARTESIAN_POINT ( 'NONE',  ( 53.50833635130540955, 57.69948385550241454, -4.867452303228209765 ) ) ;
#2566=CARTESIAN_POINT ( 'NONE',  ( 50.02271294988505446, 46.50051614449765935, -7.000000000000000888 ) ) ;
#2567=CARTESIAN_POINT ( 'NONE',  ( 41.58830220609386430, 52.00051614449766646, -0.02388180880514929535 ) ) ;
#2570=CARTESIAN_POINT ( 'NONE',  ( 54.08601618280673051, 45.00000000000005684, -5.120135501906166731 ) ) ;
#2572=CARTESIAN_POINT ( 'NONE',  ( 45.31609314410960820, 46.30051614449766362, -6.485486291978072693 ) ) ;
#2581=CARTESIAN_POINT ( 'NONE',  ( 44.05948171654949874, 54.79948385550241596, 4.345558710429105354 ) ) ;
#2582=CARTESIAN_POINT ( 'NONE',  ( 56.30877334542961421, 61.00051614449765935, 0.02388180880515774693 ) ) ;
#2585=CARTESIAN_POINT ( 'NONE',  ( 55.08986747509849380, 63.20051614449766220, 3.727524721679155384 ) ) ;
#2586=CARTESIAN_POINT ( 'NONE',  ( 44.91013252490152752, 48.79948385550240175, 3.727524721679198461 ) ) ;
#2594=( NAMED_UNIT ( * ) PLANE_ANGLE_UNIT ( ) SI_UNIT ( $, .RADIAN. ) );
#2597=CARTESIAN_POINT ( 'NONE',  ( 55.96859303347802239, 58.80051614449764941, -4.306917132069484566 ) ) ;
#2601=CARTESIAN_POINT ( 'NONE',  ( 52.25172492374522903, 49.59948385550240602, -7.007379884777225953 ) ) ;
#2602=CARTESIAN_POINT ( 'NONE',  ( 52.29715082351547295, 48.39948385550240317, 6.992620115222774047 ) ) ;
#2604=CARTESIAN_POINT ( 'NONE',  ( 54.68390685589033495, 61.69948385550240744, -6.485486291978119766 ) ) ;
#2613=CARTESIAN_POINT ( 'NONE',  ( 49.97728705011494554, 51.50051614449765935, 6.000000000000000888 ) ) ;
#2615=CARTESIAN_POINT ( 'NONE',  ( 42.38452918213188525, 51.09948385550240602, -2.450534656007040013 ) ) ;
#2616=CARTESIAN_POINT ( 'NONE',  ( 44.05948171654949874, 56.79948385550240886, 4.345558710429105354 ) ) ;
#2618=CARTESIAN_POINT ( 'NONE',  ( 50.02271294988513972, 46.49948385550240459, 8.000000000000001776 ) ) ;
#2632=CARTESIAN_POINT ( 'NONE',  ( 51.97223112728254790, 58.39948385550241028, 5.992620115222778487 ) ) ;
#2633=CARTESIAN_POINT ( 'NONE',  ( 49.97728705011495265, 45.50051614449765935, 7.000000000000000888 ) ) ;
#2634=CARTESIAN_POINT ( 'NONE',  ( 54.72065718078918906, 50.70051614449766220, -6.458785618021089192 ) ) ;
#2637=B_SPLINE_CURVE_WITH_KNOTS ( 'NONE', 3,
 ( #5166, #11372, #9434, #1891, #3072, #6136, #3006, #1961, #11437, #836 ),
 .UNSPECIFIED., .F., .F.,
 ( 4, 2, 2, 2, 4 ),
 ( 0.000000000000000000, 0.003112635120760290971, 0.004668952681140444913, 0.005447111461330522535, 0.006225270241520600156 ),
 .UNSPECIFIED. ) ;
#2639=CARTESIAN_POINT ( 'NONE',  ( 43.33558569842706021, 61.90051614449766504, 2.141517661632167169 ) ) ;
#2650=CARTESIAN_POINT ( 'NONE',  ( 43.33558569842703179, 57.09948385550240602, -2.141517661632099223 ) ) ;
#2652=CARTESIAN_POINT ( 'NONE',  ( 53.54508667620424234, 58.70051614449765509, -4.840751629271188961 ) ) ;
#2655=CARTESIAN_POINT ( 'NONE',  ( 44.05948171654945611, 46.20051614449766930, -4.345558710429044069 ) ) ;
#2656=CARTESIAN_POINT ( 'NONE',  ( 47.74827507625478518, 64.59948385550239891, 7.007379884777227730 ) ) ;
#2669=CARTESIAN_POINT ( 'NONE',  ( 56.65037692655921120, 63.10051614449766078, 2.184720259617097593 ) ) ;
#2672=CARTESIAN_POINT ( 'NONE',  ( 54.13287192849676188, 56.29948385550240175, 5.649768623646098220 ) ) ;
#2673=CARTESIAN_POINT ( 'NONE',  ( 50.02271294988512551, 46.49948385550240459, 7.000000000000000888 ) ) ;
#2676=CARTESIAN_POINT ( 'NONE',  ( 45.86712807150323812, 51.29948385550240175, -5.649768623646098220 ) ) ;
#2686=CARTESIAN_POINT ( 'NONE',  ( 51.97223112728249816, 60.60051614449765367, -5.992620115222793586 ) ) ;
#2688=CARTESIAN_POINT ( 'NONE',  ( 49.97728705011486738, 61.49948385550241170, -8.000000000000001776 ) ) ;
#2689=CARTESIAN_POINT ( 'NONE',  ( 55.96859303347804371, 60.19948385550240744, 4.306917132069425946 ) ) ;
#2691=CARTESIAN_POINT ( 'NONE',  ( 43.18075615816994173, 63.80051614449766362, 4.924951120819380357 ) ) ;
#2703=CARTESIAN_POINT ( 'NONE',  ( 51.92680522751233951, 63.59948385550239891, -6.007379884777223289 ) ) ;
#2704=CARTESIAN_POINT ( 'NONE',  ( 45.90387839640208512, 52.30051614449766362, -5.676469297603124353 ) ) ;
#2705=CARTESIAN_POINT ( 'NONE',  ( 58.41169779390614281, 51.00051614449765935, 0.02388180880515032231 ) ) ;
#2709=CARTESIAN_POINT ( 'NONE',  ( 43.20883090819742023, 46.20051614449766220, -4.963592699178938972 ) ) ;
#2717=PLANE ( 'NONE',  #7832 ) ;
#2722=CARTESIAN_POINT ( 'NONE',  ( 54.09612160359786515, 55.69948385550240744, -5.676469297603166098 ) ) ;
#2723=CARTESIAN_POINT ( 'NONE',  ( 52.29715082351547295, 58.39948385550240317, 6.992620115222774047 ) ) ;
#2728=CARTESIAN_POINT ( 'NONE',  ( 44.28664221472221385, 61.90051614449766504, 1.832500667257213722 ) ) ;
#2729=CARTESIAN_POINT ( 'NONE',  ( 44.28664221472220675, 53.09948385550240602, -1.832500667257165317 ) ) ;
#2742=CARTESIAN_POINT ( 'NONE',  ( 56.66441430157294690, 60.90051614449766504, -2.141517661632166281 ) ) ;
#2744=CARTESIAN_POINT ( 'NONE',  ( 53.54508667620424234, 44.70051614449765509, -4.840751629271188961 ) ) ;
#2747=CARTESIAN_POINT ( 'NONE',  ( 52.29715082351547295, 56.39948385550238896, 6.992620115222774047 ) ) ;
#2748=CARTESIAN_POINT ( 'NONE',  ( 54.09612160359786515, 49.69948385550240744, -5.676469297603166098 ) ) ;
#2750=CARTESIAN_POINT ( 'NONE',  ( 52.25172492374522903, 47.59948385550239891, -7.007379884777225953 ) ) ;
#2760=CARTESIAN_POINT ( 'NONE',  ( 55.71335778527780036, 60.90051614449766504, -1.832500667257213056 ) ) ;
#2762=CARTESIAN_POINT ( 'NONE',  ( 54.72065718078924590, 60.29948385550240175, 6.458785618021043895 ) ) ;
#2763=CARTESIAN_POINT ( 'NONE',  ( 49.97728705011488159, 65.49948385550240459, -7.000000000000000888 ) ) ;
#2766=CARTESIAN_POINT ( 'NONE',  ( 42.39856655714566358, 48.89948385550241028, 2.493737253992119207 ) ) ;
#2778=CARTESIAN_POINT ( 'NONE',  ( 50.02271294988506156, 44.50051614449765935, -6.000000000000000888 ) ) ;
#2779=CARTESIAN_POINT ( 'NONE',  ( 56.66441430157294690, 50.90051614449766504, -2.141517661632166281 ) ) ;
#2780=CARTESIAN_POINT ( 'NONE',  ( 56.81924384183006538, 58.80051614449766362, -4.924951120819380357 ) ) ;
#2784=CARTESIAN_POINT ( 'NONE',  ( 57.60143344285435774, 51.10051614449766078, 2.493737253992045044 ) ) ;
#2794=CARTESIAN_POINT ( 'NONE',  ( 55.94051828345050836, 63.79948385550240886, -4.345558710429104465 ) ) ;
#2795=CARTESIAN_POINT ( 'NONE',  ( 49.97728705011488159, 59.49948385550240459, -7.000000000000000888 ) ) ;
#2800=CARTESIAN_POINT ( 'NONE',  ( 46.45491332379576477, 63.70051614449766930, 4.840751629271188961 ) ) ;
#2801=CARTESIAN_POINT ( 'NONE',  ( 44.30067958973596376, 52.89948385550241028, 1.875703265242204099 ) ) ;
#2811=PRESENTATION_STYLE_ASSIGNMENT (( #7928 ) ) ;
#2812=CARTESIAN_POINT ( 'NONE',  ( 55.94051828345050836, 45.79948385550240886, -4.345558710429104465 ) ) ;
#2814=CARTESIAN_POINT ( 'NONE',  ( 51.97223112728249816, 44.60051614449766078, -5.992620115222793586 ) ) ;
#2816=CARTESIAN_POINT ( 'NONE',  ( 45.86712807150323812, 57.29948385550240175, -5.649768623646098220 ) ) ;
#2817=CARTESIAN_POINT ( 'NONE',  ( 45.86712807150323812, 53.29948385550240886, -5.649768623646098220 ) ) ;
#2819=CARTESIAN_POINT ( 'NONE',  ( 54.13287192849676188, 48.29948385550240175, 5.649768623646098220 ) ) ;
#2827=CARTESIAN_POINT ( 'NONE',  ( 48.02776887271750184, 59.60051614449765367, 5.992620115222795363 ) ) ;
#2830=CARTESIAN_POINT ( 'NONE',  ( 57.60143344285433642, 57.89948385550241028, -2.493737253992118319 ) ) ;
#2833=CARTESIAN_POINT ( 'NONE',  ( 42.38452918213188525, 47.09948385550240602, -2.450534656007040013 ) ) ;
#2844=CARTESIAN_POINT ( 'NONE',  ( 55.71335778527780036, 44.90051614449765793, -1.832500667257213056 ) ) ;
#2845=CARTESIAN_POINT ( 'NONE',  ( 44.05948171654945611, 54.20051614449765509, -4.345558710429044069 ) ) ;
#2846=CARTESIAN_POINT ( 'NONE',  ( 47.42335538002180328, 60.40051614449765793, -8.007379884777206414 ) ) ;
#2849=CARTESIAN_POINT ( 'NONE',  ( 57.60143344285435774, 53.10051614449767499, 2.493737253992045044 ) ) ;
#2859=PRODUCT_CONTEXT ( 'NONE', #11835, 'mechanical' ) ;
#2860=CARTESIAN_POINT ( 'NONE',  ( 44.03140696652192787, 63.19948385550240744, -4.306917132069425058 ) ) ;
#2862=CARTESIAN_POINT ( 'NONE',  ( 44.05948171654949874, 58.79948385550240175, 4.345558710429104465 ) ) ;
#2867=CARTESIAN_POINT ( 'NONE',  ( 52.29715082351538769, 48.60051614449766788, -6.992620115222796251 ) ) ;
#2868=CARTESIAN_POINT ( 'NONE',  ( 55.71335778527780747, 52.09948385550241312, 1.832500667257165983 ) ) ;
#2879=CARTESIAN_POINT ( 'NONE',  ( 43.33558569842703179, 47.09948385550240602, -2.141517661632099223 ) ) ;
#2882=CARTESIAN_POINT ( 'NONE',  ( 55.69932041026405045, 45.10051614449766788, 1.875703265242156359 ) ) ;
#2884=CARTESIAN_POINT ( 'NONE',  ( 50.02271294988512551, 58.49948385550241170, 7.000000000000000888 ) ) ;
#2885=CARTESIAN_POINT ( 'NONE',  ( 47.70284917648453415, 51.39948385550238896, -6.992620115222774047 ) ) ;
#2888=CARTESIAN_POINT ( 'NONE',  ( 54.13287192849676188, 50.29948385550240175, 5.649768623646098220 ) ) ;
#2898=CARTESIAN_POINT ( 'NONE',  ( 44.28664221472221385, 61.90051614449766504, 1.832500667257213722 ) ) ;
#2901=CARTESIAN_POINT ( 'NONE',  ( 52.57664461997811856, 61.59948385550240602, -8.007379884777229506 ) ) ;
#2902=CARTESIAN_POINT ( 'NONE',  ( 44.05948171654949874, 64.79948385550240175, 4.345558710429105354 ) ) ;
#2903=DIRECTION ( 'NONE',  ( -0.9989677110047504582, -0.04542589977017007230, 1.386346192018204258E-14 ) ) ;
#2904=CARTESIAN_POINT ( 'NONE',  ( 45.31609314410967926, 52.69948385550240744, 6.485486291978119766 ) ) ;
#2915=CARTESIAN_POINT ( 'NONE',  ( 49.97728705011488870, 63.49948385550241170, -6.000000000000000888 ) ) ;
#2916=CARTESIAN_POINT ( 'NONE',  ( 47.74827507625470702, 50.40051614449765793, -7.007379884777204637 ) ) ;
#2917=CARTESIAN_POINT ( 'NONE',  ( 41.58830220609386430, 58.00051614449765935, -0.02388180880514929535 ) ) ;
#2921=CARTESIAN_POINT ( 'NONE',  ( 45.27934281921082516, 51.70051614449765509, 6.458785618021089192 ) ) ;
#2934=CARTESIAN_POINT ( 'NONE',  ( 56.30877334542961421, 45.99948385550240459, -0.02388180880520959434 ) ) ;
#2935=CARTESIAN_POINT ( 'NONE',  ( 44.05948171654949874, 60.79948385550240886, 4.345558710429104465 ) ) ;
#2939=CARTESIAN_POINT ( 'NONE',  ( 57.36023556966787851, 53.00051614449765225, 0.02388180880515038476 ) ) ;
#2940=CARTESIAN_POINT ( 'NONE',  ( 44.91013252490152752, 54.79948385550240175, 3.727524721679198461 ) ) ;
#2941=CARTESIAN_POINT ( 'NONE',  ( 54.89903213687075834, 44.74560054925188268, -5.000000000000007105 ) ) ;
#2955=CARTESIAN_POINT ( 'NONE',  ( 53.54508667620428497, 64.29948385550240175, 4.840751629271157874 ) ) ;
#2957=CARTESIAN_POINT ( 'NONE',  ( 49.97728705011488159, 59.49948385550240459, -7.000000000000000888 ) ) ;
#2958=CARTESIAN_POINT ( 'NONE',  ( 54.13287192849676188, 52.29948385550240886, 5.649768623646098220 ) ) ;
#2960=CARTESIAN_POINT ( 'NONE',  ( 57.36023556966787851, 47.99948385550239038, -0.02388180880522424582 ) ) ;
#2968=CARTESIAN_POINT ( 'NONE',  ( 54.09612160359786515, 45.69948385550240744, -5.676469297603166098 ) ) ;
#2969=CARTESIAN_POINT ( 'NONE',  ( 50.02271294988506156, 60.50051614449766646, -6.000000000000000888 ) ) ;
#2971=CARTESIAN_POINT ( 'NONE',  ( 57.61547081786812896, 58.09948385550241312, 2.450534656007040901 ) ) ;
#2976=CARTESIAN_POINT ( 'NONE',  ( 41.58830220609386430, 46.99948385550239749, 0.02388180880523263147 ) ) ;
#2988=CARTESIAN_POINT ( 'NONE',  ( 44.28664221472220675, 61.09948385550241312, -1.832500667257165317 ) ) ;
#2989=CARTESIAN_POINT ( 'NONE',  ( 47.70284917648459810, 51.60051614449765367, 6.992620115222797139 ) ) ;
#2990=CARTESIAN_POINT ( 'NONE',  ( 57.60143344285435774, 59.10051614449766078, 2.493737253992045044 ) ) ;
#2992=CARTESIAN_POINT ( 'NONE',  ( 47.42335538002180328, 48.40051614449766504, -8.007379884777206414 ) ) ;
#3001=CARTESIAN_POINT ( 'NONE',  ( 43.34962307344081012, 62.89948385550241028, 2.184720259617164650 ) ) ;
#3002=CARTESIAN_POINT ( 'NONE',  ( 44.03140696652193498, 57.19948385550239323, -4.306917132069424170 ) ) ;
#3003=CARTESIAN_POINT ( 'NONE',  ( 52.29715082351538769, 60.60051614449764656, -6.992620115222796251 ) ) ;
#3006=CARTESIAN_POINT ( 'NONE',  ( 54.76112626223286384, 45.00000000000007816, -5.734953493745535091 ) ) ;
#3007=CARTESIAN_POINT ( 'NONE',  ( 44.03140696652198471, 51.80051614449766362, 4.306917132069485454 ) ) ;
#3008=CARTESIAN_POINT ( 'NONE',  ( 50.02271294988511841, 52.49948385550241170, 6.000000000000000888 ) ) ;
#3020=CARTESIAN_POINT ( 'NONE',  ( 49.97728705011488159, 45.49948385550240459, -7.000000000000000888 ) ) ;
#3022=CARTESIAN_POINT ( 'NONE',  ( 44.28664221472220675, 65.09948385550239891, -1.832500667257165317 ) ) ;
#3024=CARTESIAN_POINT ( 'NONE',  ( 45.86712807150323812, 65.29948385550241596, -5.649768623646098220 ) ) ;
#3025=CARTESIAN_POINT ( 'NONE',  ( 47.74827507625478518, 54.59948385550239180, 7.007379884777227730 ) ) ;
#3027=CARTESIAN_POINT ( 'NONE',  ( 47.74827507625478518, 52.59948385550239180, 7.007379884777227730 ) ) ;
#3033=CARTESIAN_POINT ( 'NONE',  ( 52.29715082351547295, 46.39948385550240317, 6.992620115222774047 ) ) ;
#3034=CARTESIAN_POINT ( 'NONE',  ( 47.74827507625469281, 46.40051614449764372, -7.007379884777203749 ) ) ;
#3036=CARTESIAN_POINT ( 'NONE',  ( 57.61547081786812896, 64.09948385550239891, 2.450534656007040901 ) ) ;
#3040=CARTESIAN_POINT ( 'NONE',  ( 52.57664461997811856, 47.59948385550239891, -8.007379884777229506 ) ) ;
#3044=CARTESIAN_POINT ( 'NONE',  ( 54.31203442848995877, 44.90264883920728778, -4.999999999999999112 ) ) ;
#3049=CARTESIAN_POINT ( 'NONE',  ( 55.11794222512599362, 48.80051614449767072, -3.688883143319583446 ) ) ;
#3050=CARTESIAN_POINT ( 'NONE',  ( 54.09612160359792199, 59.30051614449766362, 5.676469297603124353 ) ) ;
#3051=CARTESIAN_POINT ( 'NONE',  ( 58.41169779390614281, 57.00051614449766646, 0.02388180880515032231 ) ) ;
#3053=CARTESIAN_POINT ( 'NONE',  ( 50.02271294988505446, 50.50051614449765935, -8.000000000000001776 ) ) ;
#3058=UNCERTAINTY_MEASURE_WITH_UNIT (LENGTH_MEASURE( 1.000000000000000082E-05 ), #12513, 'distance_accuracy_value', 'NONE');
#3064=CARTESIAN_POINT ( 'NONE',  ( 54.09612160359786515, 61.69948385550240744, -5.676469297603166098 ) ) ;
#3066=CARTESIAN_POINT ( 'NONE',  ( 54.13287192849676188, 64.29948385550241596, 5.649768623646098220 ) ) ;
#3068=CARTESIAN_POINT ( 'NONE',  ( 43.34962307344078880, 58.10051614449766078, -2.184720259617096705 ) ) ;
#3072=CARTESIAN_POINT ( 'NONE',  ( 53.94396537754659704, 44.99999999999997158, -6.362703256440709332 ) ) ;
#3073=CARTESIAN_POINT ( 'NONE',  ( 44.05948171654945611, 52.20051614449764799, -4.345558710429044069 ) ) ;
#3074=CARTESIAN_POINT ( 'NONE',  ( 50.02271294988511841, 60.49948385550240459, 6.000000000000000888 ) ) ;
#3090=CARTESIAN_POINT ( 'NONE',  ( 51.92680522751238925, 49.40051614449766504, 6.007379884777208190 ) ) ;
#3092=CARTESIAN_POINT ( 'NONE',  ( 56.65037692655918988, 63.89948385550239607, -2.184720259617163762 ) ) ;
#3093=CARTESIAN_POINT ( 'NONE',  ( 42.63976443033212860, 54.99948385550241170, 0.02388180880522514787 ) ) ;
#3102=CARTESIAN_POINT ( 'NONE',  ( 56.65037692655918988, 45.89948385550240317, -2.184720259617163762 ) ) ;
#3104=CARTESIAN_POINT ( 'NONE',  ( 43.33558569842706021, 49.90051614449766504, 2.141517661632167169 ) ) ;
#3106=EDGE_CURVE ( 'NONE', #9468, #9956, #144, .T. ) ;
#3107=CARTESIAN_POINT ( 'NONE',  ( 54.13287192849676188, 46.29948385550240886, 5.649768623646098220 ) ) ;
#3111=CARTESIAN_POINT ( 'NONE',  ( 54.72065718078924590, 58.29948385550240886, 6.458785618021043895 ) ) ;
#3118=CARTESIAN_POINT ( 'NONE',  ( 55.69932041026405045, 47.10051614449766078, 1.875703265242156359 ) ) ;
#3119=CARTESIAN_POINT ( 'NONE',  ( 56.66441430157294690, 56.90051614449766504, -2.141517661632166281 ) ) ;
#3120=CARTESIAN_POINT ( 'NONE',  ( 52.62207051974829852, 62.60051614449765367, -7.992620115222797139 ) ) ;
#3122=CARTESIAN_POINT ( 'NONE',  ( 50.02271294988505446, 56.50051614449767357, -8.000000000000001776 ) ) ;
#3124=PRODUCT_DEFINITION_SHAPE ( 'NONE', 'NONE',  #10642 ) ;
#3134=CARTESIAN_POINT ( 'NONE',  ( 48.02776887271745210, 47.39948385550241028, -5.992620115222778487 ) ) ;
#3139=CARTESIAN_POINT ( 'NONE',  ( 57.61547081786810764, 44.90051614449765793, -2.450534656007114176 ) ) ;
#3143=CARTESIAN_POINT ( 'NONE',  ( 43.34962307344078880, 50.10051614449766078, -2.184720259617096705 ) ) ;
#3144=CARTESIAN_POINT ( 'NONE',  ( 55.08986747509847248, 59.79948385550240175, -3.727524721679197572 ) ) ;
#3157=CARTESIAN_POINT ( 'NONE',  ( 54.09612160359786515, 53.69948385550240744, -5.676469297603166098 ) ) ;
#3158=CARTESIAN_POINT ( 'NONE',  ( 49.99999999999997158, 45.00000000000001421, -6.500000000000004441 ) ) ;
#3159=CARTESIAN_POINT ( 'NONE',  ( 44.91013252490150620, 52.20051614449766220, -3.727524721679154940 ) ) ;
#3162=CARTESIAN_POINT ( 'NONE',  ( 56.66441430157296821, 62.09948385550239891, 2.141517661632100111 ) ) ;
#3163=CARTESIAN_POINT ( 'NONE',  ( 54.09612160359786515, 57.69948385550240744, -5.676469297603166098 ) ) ;
#3168=CLOSED_SHELL ( 'NONE', ( #5681, #5378, #3734, #5913, #6032, #13101 ) ) ;
#3174=CARTESIAN_POINT ( 'NONE',  ( 42.63976443033212860, 46.00051614449766646, -0.02388180880514948964 ) ) ;
#3176=CARTESIAN_POINT ( 'NONE',  ( 42.38452918213188525, 63.09948385550240602, -2.450534656007040013 ) ) ;
#3178=CARTESIAN_POINT ( 'NONE',  ( 47.42335538002188144, 56.59948385550239891, 8.007379884777233059 ) ) ;
#3188=CARTESIAN_POINT ( 'NONE',  ( 55.08986747509849380, 49.20051614449766220, 3.727524721679155384 ) ) ;
#3189=CARTESIAN_POINT ( 'NONE',  ( 54.13287192849671214, 56.70051614449766220, -5.649768623646139964 ) ) ;
#3191=CARTESIAN_POINT ( 'NONE',  ( 52.62207051974839089, 48.39948385550240317, 7.992620115222770494 ) ) ;
#3194=CARTESIAN_POINT ( 'NONE',  ( 42.39856655714564226, 58.10051614449765367, -2.493737253992044156 ) ) ;
#3206=CARTESIAN_POINT ( 'NONE',  ( 51.92680522751233951, 51.59948385550240602, -6.007379884777223289 ) ) ;
#3209=CARTESIAN_POINT ( 'NONE',  ( 43.33558569842706021, 63.90051614449765793, 2.141517661632167169 ) ) ;
#3214=CARTESIAN_POINT ( 'NONE',  ( 55.96859303347802239, 54.80051614449764230, -4.306917132069484566 ) ) ;
#3215=CARTESIAN_POINT ( 'NONE',  ( 51.97223112728254790, 60.39948385550241028, 5.992620115222778487 ) ) ;
#3225=CARTESIAN_POINT ( 'NONE',  ( 45.86712807150323812, 49.29948385550240175, -5.649768623646098220 ) ) ;
#3227=CARTESIAN_POINT ( 'NONE',  ( 43.69122665457040000, 54.00051614449765935, -0.02388180880515696977 ) ) ;
#3230=CARTESIAN_POINT ( 'NONE',  ( 57.36023556966787851, 63.99948385550241881, -0.02388180880522424582 ) ) ;
#3232=CARTESIAN_POINT ( 'NONE',  ( 42.63976443033212860, 62.99948385550241170, 0.02388180880522514787 ) ) ;
#3242=CARTESIAN_POINT ( 'NONE',  ( 44.03140696652193498, 49.19948385550240744, -4.306917132069424170 ) ) ;
#3243=CARTESIAN_POINT ( 'NONE',  ( 45.86712807150329496, 45.70051614449766220, 5.649768623646139964 ) ) ;
#3245=CARTESIAN_POINT ( 'NONE',  ( 44.05948171654949874, 46.79948385550238754, 4.345558710429105354 ) ) ;
#3250=CARTESIAN_POINT ( 'NONE',  ( 54.72065718078924590, 56.29948385550240886, 6.458785618021043895 ) ) ;
#3257=CARTESIAN_POINT ( 'NONE',  ( 44.30067958973594955, 48.10051614449766078, -1.875703265242155693 ) ) ;
#3258=CARTESIAN_POINT ( 'NONE',  ( 52.25172492374528588, 61.40051614449765793, 7.007379884777204637 ) ) ;
#3259=CARTESIAN_POINT ( 'NONE',  ( 42.38452918213188525, 47.09948385550240602, -2.450534656007040013 ) ) ;
#3262=CARTESIAN_POINT ( 'NONE',  ( 47.42335538002180328, 54.40051614449765793, -8.007379884777206414 ) ) ;
#3269=DIRECTION ( 'NONE',  ( -0.9989677110047502362, -0.04542589977017699732, 6.931730960091013400E-15 ) ) ;
#3271=CARTESIAN_POINT ( 'NONE',  ( 44.30067958973596376, 50.89948385550240317, 1.875703265242204099 ) ) ;
#3273=CARTESIAN_POINT ( 'NONE',  ( 57.60143344285435774, 45.10051614449766788, 2.493737253992045044 ) ) ;
#3276=CARTESIAN_POINT ( 'NONE',  ( 42.63976443033212860, 56.00051614449765935, -0.02388180880514948964 ) ) ;
#3277=CARTESIAN_POINT ( 'NONE',  ( 46.45491332379572924, 59.29948385550240886, -4.840751629271157874 ) ) ;
#3288=CARTESIAN_POINT ( 'NONE',  ( 43.33558569842703179, 51.09948385550240602, -2.141517661632099223 ) ) ;
#3290=CARTESIAN_POINT ( 'NONE',  ( 51.92680522751238925, 53.40051614449765793, 6.007379884777208190 ) ) ;
#3294=CARTESIAN_POINT ( 'NONE',  ( 47.74827507625478518, 62.59948385550240602, 7.007379884777227730 ) ) ;
#3304=( GEOMETRIC_REPRESENTATION_CONTEXT ( 3 ) GLOBAL_UNCERTAINTY_ASSIGNED_CONTEXT ( ( #3058 ) ) GLOBAL_UNIT_ASSIGNED_CONTEXT ( ( #12513, #12583, #185 ) ) REPRESENTATION_CONTEXT ( 'NONE', 'WORKASPACE' ) );
#3307=CARTESIAN_POINT ( 'NONE',  ( 49.97728705011488159, 51.49948385550240459, -7.000000000000000888 ) ) ;
#3308=CARTESIAN_POINT ( 'NONE',  ( 45.90387839640208512, 46.30051614449766362, -5.676469297603124353 ) ) ;
#3311=CARTESIAN_POINT ( 'NONE',  ( 49.97728705011486738, 63.49948385550241170, -8.000000000000001776 ) ) ;
#3314=CARTESIAN_POINT ( 'NONE',  ( 42.38452918213188525, 55.09948385550241312, -2.450534656007040013 ) ) ;
#3323=CARTESIAN_POINT ( 'NONE',  ( 44.88205777487401349, 47.80051614449764941, 3.688883143319584779 ) ) ;
#3324=CARTESIAN_POINT ( 'NONE',  ( 55.94051828345054389, 59.20051614449765509, 4.345558710429044957 ) ) ;
#3325=CARTESIAN_POINT ( 'NONE',  ( 49.97728705011495265, 63.50051614449765935, 8.000000000000001776 ) ) ;
#3327=CARTESIAN_POINT ( 'NONE',  ( 45.31609314410960820, 54.30051614449765651, -6.485486291978072693 ) ) ;
#3338=CARTESIAN_POINT ( 'NONE',  ( 55.69932041026404335, 51.89948385550241028, -1.875703265242203432 ) ) ;
#3339=CARTESIAN_POINT ( 'NONE',  ( 45.90387839640214196, 62.69948385550240744, 5.676469297603166098 ) ) ;
#3340=CARTESIAN_POINT ( 'NONE',  ( 49.97728705011495265, 47.50051614449765935, 8.000000000000001776 ) ) ;
#3345=CARTESIAN_POINT ( 'NONE',  ( 54.13287192849671214, 56.70051614449766220, -5.649768623646139964 ) ) ;
#3346=CARTESIAN_POINT ( 'NONE',  ( 44.91013252490152752, 56.79948385550240175, 3.727524721679198461 ) ) ;
#3355=CARTESIAN_POINT ( 'NONE',  ( 55.94051828345050836, 53.79948385550238754, -4.345558710429104465 ) ) ;
#3357=CARTESIAN_POINT ( 'NONE',  ( 53.54508667620424234, 52.70051614449766220, -4.840751629271188961 ) ) ;
#3359=PLANE ( 'NONE',  #1505 ) ;
#3361=CARTESIAN_POINT ( 'NONE',  ( 43.33558569842703179, 61.09948385550240602, -2.141517661632099223 ) ) ;
#3374=CARTESIAN_POINT ( 'NONE',  ( 55.96859303347805081, 52.19948385550240033, 4.306917132069425058 ) ) ;
#3376=CARTESIAN_POINT ( 'NONE',  ( 50.02271294988505446, 54.50051614449765935, -7.000000000000000888 ) ) ;
#3377=CARTESIAN_POINT ( 'NONE',  ( 49.99999999999997158, 45.00000000000001421, -7.499999999999998224 ) ) ;
#3378=CARTESIAN_POINT ( 'NONE',  ( 50.02271294988512551, 50.49948385550240459, 7.000000000000000888 ) ) ;
#3381=CARTESIAN_POINT ( 'NONE',  ( 50.02271294988513972, 56.49948385550240459, 8.000000000000001776 ) ) ;
#3389=CARTESIAN_POINT ( 'NONE',  ( 44.88205777487401349, 57.80051614449766362, 3.688883143319584779 ) ) ;
#3392=CARTESIAN_POINT ( 'NONE',  ( 54.72065718078918906, 62.70051614449766220, -6.458785618021089192 ) ) ;
#3395=CARTESIAN_POINT ( 'NONE',  ( 56.79116909180259398, 57.20051614449766220, 4.963592699178938972 ) ) ;
#3406=CARTESIAN_POINT ( 'NONE',  ( 48.07319477248768180, 52.59948385550240602, 6.007379884777225953 ) ) ;
#3407=CARTESIAN_POINT ( 'NONE',  ( 56.66441430157294690, 44.90051614449765793, -2.141517661632166281 ) ) ;
#3409=CARTESIAN_POINT ( 'NONE',  ( 42.39856655714564226, 48.10051614449766078, -2.493737253992044156 ) ) ;
#3413=CARTESIAN_POINT ( 'NONE',  ( 56.65037692655921120, 55.10051614449766078, 2.184720259617097593 ) ) ;
#3414=CARTESIAN_POINT ( 'NONE',  ( 44.88205777487398507, 63.19948385550240744, -3.688883143319540814 ) ) ;
#3424=CARTESIAN_POINT ( 'NONE',  ( 47.74827507625478518, 52.59948385550239180, 7.007379884777227730 ) ) ;
#3427=CARTESIAN_POINT ( 'NONE',  ( 55.69932041026405045, 55.10051614449765367, 1.875703265242156359 ) ) ;
#3432=CARTESIAN_POINT ( 'NONE',  ( 45.86712807150323812, 57.29948385550240175, -5.649768623646098220 ) ) ;
#3442=CARTESIAN_POINT ( 'NONE',  ( 49.99999999999997158, 65.00000000000002842, -7.000000000000000888 ) ) ;
#3443=CARTESIAN_POINT ( 'NONE',  ( 52.29715082351547295, 50.39948385550241028, 6.992620115222774047 ) ) ;
#3444=CARTESIAN_POINT ( 'NONE',  ( 56.66441430157294690, 56.90051614449766504, -2.141517661632166281 ) ) ;
#3446=CARTESIAN_POINT ( 'NONE',  ( 47.70284917648453415, 49.39948385550238896, -6.992620115222774047 ) ) ;
#3448=CARTESIAN_POINT ( 'NONE',  ( 58.41169779390614281, 61.99948385550241170, -0.02388180880523160798 ) ) ;
#3457=CARTESIAN_POINT ( 'NONE',  ( 44.30067958973594955, 52.10051614449766788, -1.875703265242155693 ) ) ;
#3460=CARTESIAN_POINT ( 'NONE',  ( 57.60143344285433642, 49.89948385550241028, -2.493737253992118319 ) ) ;
#3461=CARTESIAN_POINT ( 'NONE',  ( 42.63976443033212860, 56.99948385550241170, 0.02388180880522514787 ) ) ;
#3463=CARTESIAN_POINT ( 'NONE',  ( 42.39856655714564226, 60.10051614449766788, -2.493737253992044156 ) ) ;
#3471=DIRECTION ( 'NONE',  ( 1.000000000000000000, 0.000000000000000000, 0.000000000000000000 ) ) ;
#3474=CARTESIAN_POINT ( 'NONE',  ( 46.45491332379572924, 55.29948385550240175, -4.840751629271157874 ) ) ;
#3475=CARTESIAN_POINT ( 'NONE',  ( 55.94051828345054389, 45.20051614449765509, 4.345558710429044957 ) ) ;
#3476=CARTESIAN_POINT ( 'NONE',  ( 54.68390685589039890, 55.30051614449765651, 6.485486291978072693 ) ) ;
#3480=CARTESIAN_POINT ( 'NONE',  ( 44.05948171654945611, 60.20051614449764799, -4.345558710429044069 ) ) ;
#3489=CARTESIAN_POINT ( 'NONE',  ( 49.97728705011488159, 59.49948385550240459, -7.000000000000000888 ) ) ;
#3492=CARTESIAN_POINT ( 'NONE',  ( 55.69932041026405045, 59.10051614449766078, 1.875703265242156359 ) ) ;
#3495=CARTESIAN_POINT ( 'NONE',  ( 44.30067958973596376, 46.89948385550240317, 1.875703265242204099 ) ) ;
#3509=CARTESIAN_POINT ( 'NONE',  ( 45.86712807150323812, 53.29948385550240886, -5.649768623646098220 ) ) ;
#3510=CARTESIAN_POINT ( 'NONE',  ( 56.65037692655921120, 53.10051614449766078, 2.184720259617097593 ) ) ;
#3513=CARTESIAN_POINT ( 'NONE',  ( 45.86712807150323812, 51.29948385550240175, -5.649768623646098220 ) ) ;
#3515=CARTESIAN_POINT ( 'NONE',  ( 50.02271294988512551, 48.49948385550240459, 7.000000000000000888 ) ) ;
#3516=CARTESIAN_POINT ( 'NONE',  ( 47.37792948025162332, 61.39948385550240317, -7.992620115222770494 ) ) ;
#3524=CARTESIAN_POINT ( 'NONE',  ( 44.28664221472221385, 55.90051614449766504, 1.832500667257213722 ) ) ;
#3525=CARTESIAN_POINT ( 'NONE',  ( 44.05948171654945611, 64.20051614449766930, -4.345558710429044069 ) ) ;
#3527=CARTESIAN_POINT ( 'NONE',  ( 50.02271294988513972, 54.49948385550240459, 8.000000000000001776 ) ) ;
#3529=CARTESIAN_POINT ( 'NONE',  ( 57.36023556966787851, 53.99948385550239038, -0.02388180880522424582 ) ) ;
#3531=CARTESIAN_POINT ( 'NONE',  ( 43.20883090819742023, 60.20051614449766220, -4.963592699178938972 ) ) ;
#3541=CARTESIAN_POINT ( 'NONE',  ( 55.71335778527780747, 58.09948385550241312, 1.832500667257165983 ) ) ;
#3542=CARTESIAN_POINT ( 'NONE',  ( 45.86712807150329496, 49.70051614449766220, 5.649768623646139964 ) ) ;
#3543=CARTESIAN_POINT ( 'NONE',  ( 43.18075615816994173, 55.80051614449766362, 4.924951120819380357 ) ) ;
#3547=CARTESIAN_POINT ( 'NONE',  ( 55.94051828345053679, 63.20051614449765509, 4.345558710429044069 ) ) ;
#3554=DIRECTION ( 'NONE',  ( -1.000000000000000000, 0.000000000000000000, 1.224646799147353207E-16 ) ) ;
#3558=CARTESIAN_POINT ( 'NONE',  ( 49.97728705011488159, 57.49948385550241170, -7.000000000000000888 ) ) ;
#3559=CARTESIAN_POINT ( 'NONE',  ( 46.45491332379576477, 57.70051614449766930, 4.840751629271188961 ) ) ;
#3564=CARTESIAN_POINT ( 'NONE',  ( 46.49166364869456913, 62.30051614449766362, -4.867452303228181343 ) ) ;
#3565=CARTESIAN_POINT ( 'NONE',  ( 45.86712807150323812, 63.29948385550240886, -5.649768623646098220 ) ) ;
#3580=CARTESIAN_POINT ( 'NONE',  ( 56.66441430157294690, 50.90051614449766504, -2.141517661632166281 ) ) ;
#3583=CARTESIAN_POINT ( 'NONE',  ( 54.09612160359786515, 53.69948385550240744, -5.676469297603166098 ) ) ;
#3584=CARTESIAN_POINT ( 'NONE',  ( 45.27934281921075410, 65.29948385550241596, -6.458785618021043895 ) ) ;
#3594=CARTESIAN_POINT ( 'NONE',  ( 55.69932041026405045, 57.10051614449766788, 1.875703265242156359 ) ) ;
#3596=CARTESIAN_POINT ( 'NONE',  ( 41.58830220609386430, 54.99948385550239749, 0.02388180880523263147 ) ) ;
#3597=CARTESIAN_POINT ( 'NONE',  ( 47.70284917648453415, 59.39948385550241028, -6.992620115222774047 ) ) ;
#3600=CARTESIAN_POINT ( 'NONE',  ( 47.42335538002180328, 64.40051614449764372, -8.007379884777206414 ) ) ;
#3614=CARTESIAN_POINT ( 'NONE',  ( 44.91013252490152752, 54.79948385550240175, 3.727524721679198461 ) ) ;
#3616=CARTESIAN_POINT ( 'NONE',  ( 41.58830220609386430, 56.00051614449765935, -0.02388180880514929535 ) ) ;
#3619=CARTESIAN_POINT ( 'NONE',  ( 50.02271294988505446, 64.50051614449765225, -7.000000000000000888 ) ) ;
#3628=CARTESIAN_POINT ( 'NONE',  ( 42.63976443033212860, 56.99948385550241170, 0.02388180880522514787 ) ) ;
#3629=CARTESIAN_POINT ( 'NONE',  ( 53.54508667620424234, 60.70051614449766930, -4.840751629271188961 ) ) ;
#3634=CARTESIAN_POINT ( 'NONE',  ( 46.49166364869456913, 64.30051614449766362, -4.867452303228181343 ) ) ;
#3635=CARTESIAN_POINT ( 'NONE',  ( 51.97223112728254790, 48.39948385550240317, 5.992620115222778487 ) ) ;
#3647=CARTESIAN_POINT ( 'NONE',  ( 54.13287192849671214, 52.70051614449766220, -5.649768623646139964 ) ) ;
#3650=CARTESIAN_POINT ( 'NONE',  ( 54.13287192849676188, 54.29948385550240886, 5.649768623646098220 ) ) ;
#3651=CARTESIAN_POINT ( 'NONE',  ( 55.94051828345050836, 45.79948385550240886, -4.345558710429104465 ) ) ;
#3652=CARTESIAN_POINT ( 'NONE',  ( 42.38452918213188525, 61.09948385550241312, -2.450534656007040013 ) ) ;
#3660=CARTESIAN_POINT ( 'NONE',  ( 51.92680522751238925, 57.40051614449767214, 6.007379884777208190 ) ) ;
#3664=CARTESIAN_POINT ( 'NONE',  ( 54.68390685589033495, 53.69948385550240744, -6.485486291978119766 ) ) ;
#3666=CARTESIAN_POINT ( 'NONE',  ( 43.34962307344081012, 56.89948385550240317, 2.184720259617164650 ) ) ;
#3668=CARTESIAN_POINT ( 'NONE',  ( 45.27934281921082516, 59.70051614449766220, 6.458785618021089192 ) ) ;
#3678=CARTESIAN_POINT ( 'NONE',  ( 55.11794222512601493, 54.19948385550241454, 3.688883143319541702 ) ) ;
#3679=CARTESIAN_POINT ( 'NONE',  ( 43.33558569842706021, 45.90051614449765793, 2.141517661632167169 ) ) ;
#3680=CARTESIAN_POINT ( 'NONE',  ( 45.31609314410960820, 50.30051614449766362, -6.485486291978072693 ) ) ;
#3683=CARTESIAN_POINT ( 'NONE',  ( 56.65037692655921120, 61.10051614449766078, 2.184720259617097593 ) ) ;
#3691=CARTESIAN_POINT ( 'NONE',  ( 43.34962307344081012, 54.89948385550240317, 2.184720259617164650 ) ) ;
#3693=CARTESIAN_POINT ( 'NONE',  ( 51.97223112728249816, 58.60051614449766788, -5.992620115222793586 ) ) ;
#3696=CARTESIAN_POINT ( 'NONE',  ( 43.69122665457040000, 62.00051614449766646, -0.02388180880515696977 ) ) ;
#3697=CARTESIAN_POINT ( 'NONE',  ( 43.69122665457040000, 46.99948385550239749, 0.02388180880521036456 ) ) ;
#3708=CARTESIAN_POINT ( 'NONE',  ( 57.36023556966787851, 63.00051614449767357, 0.02388180880515038476 ) ) ;
#3711=CARTESIAN_POINT ( 'NONE',  ( 47.74827507625478518, 60.59948385550239891, 7.007379884777227730 ) ) ;
#3712=CARTESIAN_POINT ( 'NONE',  ( 44.05948171654949874, 48.79948385550238754, 4.345558710429105354 ) ) ;
#3713=CARTESIAN_POINT ( 'NONE',  ( 52.62207051974839089, 62.39948385550240317, 7.992620115222770494 ) ) ;
#3721=CARTESIAN_POINT ( 'NONE',  ( 53.50833635130544508, 61.30051614449766362, 4.867452303228181343 ) ) ;
#3723=CARTESIAN_POINT ( 'NONE',  ( 41.58830220609386430, 52.99948385550241170, 0.02388180880523263147 ) ) ;
#3724=CARTESIAN_POINT ( 'NONE',  ( 56.65037692655918988, 55.89948385550240317, -2.184720259617163762 ) ) ;
#3727=CARTESIAN_POINT ( 'NONE',  ( 49.97728705011495265, 63.50051614449765935, 8.000000000000001776 ) ) ;
#3734=ADVANCED_FACE ( 'NONE', ( #10226 ), #6244, .F. ) ;
#3745=CARTESIAN_POINT ( 'NONE',  ( 44.28664221472220675, 55.09948385550241312, -1.832500667257165317 ) ) ;
#3746=CARTESIAN_POINT ( 'NONE',  ( 49.97728705011495265, 51.50051614449765935, 7.000000000000000888 ) ) ;
#3747=CARTESIAN_POINT ( 'NONE',  ( 56.81924384183006538, 54.80051614449764941, -4.924951120819380357 ) ) ;
#3749=DIRECTION ( 'NONE',  ( 0.04542589977017006536, -0.9989677110047503472, 0.000000000000000000 ) ) ;
#3751=CARTESIAN_POINT ( 'NONE',  ( 43.18075615816994173, 45.80051614449766362, 4.924951120819380357 ) ) ;
#3759=CARTESIAN_POINT ( 'NONE',  ( 56.65037692655918988, 57.89948385550240317, -2.184720259617163762 ) ) ;
#3760=CARTESIAN_POINT ( 'NONE',  ( 49.97728705011488159, 49.49948385550240459, -7.000000000000000888 ) ) ;
#3765=CARTESIAN_POINT ( 'NONE',  ( 49.97728705011495265, 47.50051614449766646, 7.000000000000000888 ) ) ;
#3766=CARTESIAN_POINT ( 'NONE',  ( 43.34962307344081012, 64.89948385550239607, 2.184720259617164650 ) ) ;
#3778=CARTESIAN_POINT ( 'NONE',  ( 43.33558569842706021, 59.90051614449766504, 2.141517661632167169 ) ) ;
#3780=CARTESIAN_POINT ( 'NONE',  ( 44.28664221472221385, 45.90051614449766504, 1.832500667257213722 ) ) ;
#3782=CARTESIAN_POINT ( 'NONE',  ( 42.63976443033212860, 60.99948385550238328, 0.02388180880522514787 ) ) ;
#3783=CARTESIAN_POINT ( 'NONE',  ( 49.97728705011488159, 49.49948385550240459, -7.000000000000000888 ) ) ;
#3785=CARTESIAN_POINT ( 'NONE',  ( 54.09612160359786515, 49.69948385550240744, -5.676469297603166098 ) ) ;
#3796=CARTESIAN_POINT ( 'NONE',  ( 46.49166364869456913, 62.30051614449766362, -4.867452303228181343 ) ) ;
#3798=CARTESIAN_POINT ( 'NONE',  ( 50.02271294988513972, 56.49948385550240459, 8.000000000000001776 ) ) ;
#3799=CARTESIAN_POINT ( 'NONE',  ( 44.03140696652192787, 65.19948385550240744, -4.306917132069425058 ) ) ;
#3802=CARTESIAN_POINT ( 'NONE',  ( 43.18075615816989199, 53.19948385550240744, -4.924951120819313743 ) ) ;
#3815=CARTESIAN_POINT ( 'NONE',  ( 48.07319477248768180, 64.59948385550241312, 6.007379884777225953 ) ) ;
#3816=CARTESIAN_POINT ( 'NONE',  ( 55.96859303347802239, 52.80051614449765651, -4.306917132069484566 ) ) ;
#3818=CARTESIAN_POINT ( 'NONE',  ( 43.20883090819742023, 62.20051614449766220, -4.963592699178938972 ) ) ;
#3822=CARTESIAN_POINT ( 'NONE',  ( 50.38494826773854385, 45.00000000000002842, -6.500000000000005329 ) ) ;
#3823=CARTESIAN_POINT ( 'NONE',  ( 50.02271294988505446, 62.50051614449766646, -7.000000000000000888 ) ) ;
#3830=CARTESIAN_POINT ( 'NONE',  ( 57.36023556966787851, 63.99948385550241881, -0.02388180880522424582 ) ) ;
#3831=CARTESIAN_POINT ( 'NONE',  ( 45.90387839640214196, 58.69948385550240033, 5.676469297603166098 ) ) ;
#3835=CARTESIAN_POINT ( 'NONE',  ( 55.11794222512599362, 62.80051614449766362, -3.688883143319583446 ) ) ;
#3836=CARTESIAN_POINT ( 'NONE',  ( 51.97223112728254790, 50.39948385550241738, 5.992620115222778487 ) ) ;
#3847=CARTESIAN_POINT ( 'NONE',  ( 56.66441430157294690, 58.90051614449766504, -2.141517661632166281 ) ) ;
#3849=CARTESIAN_POINT ( 'NONE',  ( 56.30877334542961421, 63.99948385550241170, -0.02388180880520959434 ) ) ;
#3852=CARTESIAN_POINT ( 'NONE',  ( 52.25172492374522903, 61.59948385550239891, -7.007379884777225953 ) ) ;
#3853=CARTESIAN_POINT ( 'NONE',  ( 42.63976443033212860, 52.99948385550240459, 0.02388180880522514787 ) ) ;
#3855=CARTESIAN_POINT ( 'NONE',  ( 45.86712807150323812, 49.29948385550240175, -5.649768623646098220 ) ) ;
#3864=CARTESIAN_POINT ( 'NONE',  ( 55.08986747509849380, 61.20051614449766220, 3.727524721679155384 ) ) ;
#3866=CARTESIAN_POINT ( 'NONE',  ( 57.60143344285433642, 59.89948385550240317, -2.493737253992118319 ) ) ;
#3869=CARTESIAN_POINT ( 'NONE',  ( 56.81924384183011512, 48.19948385550240744, 4.924951120819313743 ) ) ;
#3870=EDGE_LOOP ( 'NONE', ( #12509, #1157, #2363, #210 ) ) ;
#3881=CARTESIAN_POINT ( 'NONE',  ( 53.50833635130540955, 61.69948385550240744, -4.867452303228209765 ) ) ;
#3882=CARTESIAN_POINT ( 'NONE',  ( 47.70284917648459810, 53.60051614449766078, 6.992620115222797139 ) ) ;
#3883=CARTESIAN_POINT ( 'NONE',  ( 54.68390685589039890, 59.30051614449766362, 6.485486291978072693 ) ) ;
#3885=CARTESIAN_POINT ( 'NONE',  ( 54.72065718078918906, 50.70051614449766220, -6.458785618021089192 ) ) ;
#3894=CARTESIAN_POINT ( 'NONE',  ( 50.02271294988512551, 64.49948385550240459, 7.000000000000000888 ) ) ;
#3895=CARTESIAN_POINT ( 'NONE',  ( 57.36023556966787851, 55.99948385550239749, -0.02388180880522424582 ) ) ;
#3902=CARTESIAN_POINT ( 'NONE',  ( 42.63976443033212860, 54.00051614449766646, -0.02388180880514948964 ) ) ;
#3903=CARTESIAN_POINT ( 'NONE',  ( 56.30877334542961421, 49.99948385550240459, -0.02388180880520959434 ) ) ;
#3916=CARTESIAN_POINT ( 'NONE',  ( 50.02271294988506156, 46.50051614449766646, -6.000000000000000888 ) ) ;
#3918=CARTESIAN_POINT ( 'NONE',  ( 50.02271294988512551, 56.49948385550240459, 7.000000000000000888 ) ) ;
#3919=CARTESIAN_POINT ( 'NONE',  ( 47.74827507625478518, 50.59948385550238470, 7.007379884777227730 ) ) ;
#3921=CARTESIAN_POINT ( 'NONE',  ( 56.66441430157296821, 48.09948385550240602, 2.141517661632100111 ) ) ;
#3930=CARTESIAN_POINT ( 'NONE',  ( 46.45491332379576477, 59.70051614449766220, 4.840751629271188961 ) ) ;
#3934=CARTESIAN_POINT ( 'NONE',  ( 43.20883090819745576, 60.79948385550241596, 4.963592699179006473 ) ) ;
#3935=CARTESIAN_POINT ( 'NONE',  ( 55.94051828345050836, 61.79948385550239465, -4.345558710429104465 ) ) ;
#3937=CARTESIAN_POINT ( 'NONE',  ( 41.58830220609386430, 50.99948385550241170, 0.02388180880523263147 ) ) ;
#3948=CARTESIAN_POINT ( 'NONE',  ( 55.11794222512601493, 62.19948385550240744, 3.688883143319541702 ) ) ;
#3949=CARTESIAN_POINT ( 'NONE',  ( 43.33558569842706021, 55.90051614449765793, 2.141517661632167169 ) ) ;
#3950=CARTESIAN_POINT ( 'NONE',  ( 56.79116909180259398, 59.20051614449766220, 4.963592699178938972 ) ) ;
#3953=CARTESIAN_POINT ( 'NONE',  ( 47.37792948025170858, 47.60051614449766078, 7.992620115222797139 ) ) ;
#3958=VERTEX_POINT ( 'NONE', #11725 ) ;
#3963=CARTESIAN_POINT ( 'NONE',  ( 55.94051828345050836, 61.79948385550239465, -4.345558710429104465 ) ) ;
#3964=CARTESIAN_POINT ( 'NONE',  ( 57.36023556966787851, 59.99948385550240459, -0.02388180880522424582 ) ) ;
#3969=CARTESIAN_POINT ( 'NONE',  ( 56.66441430157294690, 50.90051614449766504, -2.141517661632166281 ) ) ;
#3970=CARTESIAN_POINT ( 'NONE',  ( 48.07319477248768180, 50.59948385550240602, 6.007379884777225953 ) ) ;
#3982=CARTESIAN_POINT ( 'NONE',  ( 52.25172492374522903, 47.59948385550239891, -7.007379884777225953 ) ) ;
#3987=CARTESIAN_POINT ( 'NONE',  ( 46.45491332379576477, 45.70051614449766220, 4.840751629271188961 ) ) ;
#3990=CARTESIAN_POINT ( 'NONE',  ( 44.03140696652192787, 59.19948385550238612, -4.306917132069425058 ) ) ;
#3991=CARTESIAN_POINT ( 'NONE',  ( 43.34962307344081012, 50.89948385550241028, 2.184720259617164650 ) ) ;
#3994=CARTESIAN_POINT ( 'NONE',  ( 52.29715082351547295, 52.39948385550241738, 6.992620115222774047 ) ) ;
#4002=CARTESIAN_POINT ( 'NONE',  ( 57.36023556966787851, 47.99948385550239749, -0.02388180880522424582 ) ) ;
#4004=CARTESIAN_POINT ( 'NONE',  ( 46.45491332379576477, 61.70051614449766220, 4.840751629271188961 ) ) ;
#4007=CARTESIAN_POINT ( 'NONE',  ( 56.81924384183011512, 62.19948385550240744, 4.924951120819313743 ) ) ;
#4010=CARTESIAN_POINT ( 'NONE',  ( 54.72065718078924590, 52.29948385550240886, 6.458785618021043895 ) ) ;
#4021=CARTESIAN_POINT ( 'NONE',  ( 51.97223112728254790, 64.39948385550239607, 5.992620115222778487 ) ) ;
#4022=CARTESIAN_POINT ( 'NONE',  ( 54.13287192849671214, 52.70051614449766220, -5.649768623646139964 ) ) ;
#4023=CARTESIAN_POINT ( 'NONE',  ( 47.37792948025170858, 57.60051614449765367, 7.992620115222797139 ) ) ;
#4028=CARTESIAN_POINT ( 'NONE',  ( 49.97728705011495265, 51.50051614449765935, 8.000000000000001776 ) ) ;
#4040=CARTESIAN_POINT ( 'NONE',  ( 47.74827507625478518, 62.59948385550240602, 7.007379884777227730 ) ) ;
#4041=CARTESIAN_POINT ( 'NONE',  ( 47.70284917648453415, 59.39948385550241028, -6.992620115222774047 ) ) ;
#4045=CARTESIAN_POINT ( 'NONE',  ( 50.02271294988505446, 48.50051614449765935, -7.000000000000000888 ) ) ;
#4046=CARTESIAN_POINT ( 'NONE',  ( 53.50833635130540955, 49.69948385550240744, -4.867452303228209765 ) ) ;
#4060=CARTESIAN_POINT ( 'NONE',  ( 51.92680522751238925, 47.40051614449765793, 6.007379884777208190 ) ) ;
#4062=CARTESIAN_POINT ( 'NONE',  ( 52.29715082351547295, 62.39948385550239607, 6.992620115222774047 ) ) ;
#4063=CARTESIAN_POINT ( 'NONE',  ( 54.13287192849676188, 50.29948385550240175, 5.649768623646098220 ) ) ;
#4065=CARTESIAN_POINT ( 'NONE',  ( 55.96859303347804371, 50.19948385550240744, 4.306917132069425946 ) ) ;
#4073=CARTESIAN_POINT ( 'NONE',  ( 43.33558569842703179, 49.09948385550240602, -2.141517661632099223 ) ) ;
#4076=CARTESIAN_POINT ( 'NONE',  ( 50.02271294988505446, 48.50051614449765935, -7.000000000000000888 ) ) ;
#4078=CARTESIAN_POINT ( 'NONE',  ( 54.72065718078924590, 56.29948385550240886, 6.458785618021043895 ) ) ;
#4083=CARTESIAN_POINT ( 'NONE',  ( 45.27934281921075410, 51.29948385550240175, -6.458785618021043895 ) ) ;
#4095=CARTESIAN_POINT ( 'NONE',  ( 48.07319477248762496, 46.40051614449765793, -6.007379884777208190 ) ) ;
#4097=CARTESIAN_POINT ( 'NONE',  ( 50.02271294988505446, 60.50051614449765935, -7.000000000000000888 ) ) ;
#4098=CARTESIAN_POINT ( 'NONE',  ( 41.58830220609386430, 60.00051614449765935, -0.02388180880514929535 ) ) ;
#4100=CARTESIAN_POINT ( 'NONE',  ( 52.62207051974829852, 50.60051614449765367, -7.992620115222797139 ) ) ;
#4110=CARTESIAN_POINT ( 'NONE',  ( 49.97728705011488159, 65.49948385550240459, -7.000000000000000888 ) ) ;
#4111=CARTESIAN_POINT ( 'NONE',  ( 45.86712807150323812, 61.29948385550240886, -5.649768623646098220 ) ) ;
#4112=CARTESIAN_POINT ( 'NONE',  ( 42.63976443033212860, 60.00051614449764514, -0.02388180880514948964 ) ) ;
#4116=CARTESIAN_POINT ( 'NONE',  ( 42.63976443033212860, 52.00051614449766646, -0.02388180880514948964 ) ) ;
#4117=CARTESIAN_POINT ( 'NONE',  ( 55.11794222512601493, 52.19948385550240744, 3.688883143319541702 ) ) ;
#4131=CARTESIAN_POINT ( 'NONE',  ( 53.50833635130544508, 53.30051614449767072, 4.867452303228181343 ) ) ;
#4134=CARTESIAN_POINT ( 'NONE',  ( 44.05948171654949874, 54.79948385550241596, 4.345558710429105354 ) ) ;
#4136=CARTESIAN_POINT ( 'NONE',  ( 44.05948171654949874, 52.79948385550240175, 4.345558710429105354 ) ) ;
#4143=CARTESIAN_POINT ( 'NONE',  ( 46.49166364869456913, 64.30051614449766362, -4.867452303228181343 ) ) ;
#4145=CARTESIAN_POINT ( 'NONE',  ( 42.39856655714566358, 64.89948385550239607, 2.493737253992119207 ) ) ;
#4147=CARTESIAN_POINT ( 'NONE',  ( 57.61547081786812896, 58.09948385550241312, 2.450534656007040901 ) ) ;
#4156=CARTESIAN_POINT ( 'NONE',  ( 53.54508667620424234, 46.70051614449766220, -4.840751629271188961 ) ) ;
#4157=CARTESIAN_POINT ( 'NONE',  ( 57.36023556966787851, 63.00051614449767357, 0.02388180880515038476 ) ) ;
#4159=CARTESIAN_POINT ( 'NONE',  ( 45.27934281921075410, 47.29948385550241596, -6.458785618021043895 ) ) ;
#4162=CARTESIAN_POINT ( 'NONE',  ( 47.37792948025170858, 49.60051614449766788, 7.992620115222797139 ) ) ;
#4173=CARTESIAN_POINT ( 'NONE',  ( 55.71335778527780747, 48.09948385550240602, 1.832500667257165983 ) ) ;
#4175=CARTESIAN_POINT ( 'NONE',  ( 56.65037692655918988, 63.89948385550239607, -2.184720259617163762 ) ) ;
#4176=CARTESIAN_POINT ( 'NONE',  ( 44.05948171654945611, 62.20051614449764799, -4.345558710429044069 ) ) ;
#4182=CARTESIAN_POINT ( 'NONE',  ( 55.96859303347802239, 50.80051614449766362, -4.306917132069484566 ) ) ;
#4183=CARTESIAN_POINT ( 'NONE',  ( 50.02271294988511841, 58.49948385550241170, 6.000000000000000888 ) ) ;
#4185=EDGE_CURVE ( 'NONE', #7204, #9705, #5403, .T. ) ;
#4193=CARTESIAN_POINT ( 'NONE',  ( 42.63976443033212860, 52.99948385550240459, 0.02388180880522514787 ) ) ;
#4194=PRODUCT_DEFINITION_FORMATION_WITH_SPECIFIED_SOURCE ( 'ANY', '', #13599, .NOT_KNOWN. ) ;
#4197=CARTESIAN_POINT ( 'NONE',  ( 55.08986747509849380, 53.20051614449766220, 3.727524721679155384 ) ) ;
#4200=CARTESIAN_POINT ( 'NONE',  ( 52.29715082351547295, 60.39948385550239607, 6.992620115222774047 ) ) ;
#4201=CARTESIAN_POINT ( 'NONE',  ( 47.70284917648453415, 57.39948385550241028, -6.992620115222774047 ) ) ;
#4210=CARTESIAN_POINT ( 'NONE',  ( 43.34962307344081012, 48.89948385550240317, 2.184720259617164650 ) ) ;
#4211=CARTESIAN_POINT ( 'NONE',  ( 56.66441430157294690, 44.90051614449765793, -2.141517661632166281 ) ) ;
#4213=CARTESIAN_POINT ( 'NONE',  ( 52.25172492374522903, 45.59948385550240602, -7.007379884777225953 ) ) ;
#4216=CARTESIAN_POINT ( 'NONE',  ( 41.58830220609386430, 54.99948385550239749, 0.02388180880523263147 ) ) ;
#4224=CARTESIAN_POINT ( 'NONE',  ( 46.49166364869456913, 48.30051614449765651, -4.867452303228181343 ) ) ;
#4225=CARTESIAN_POINT ( 'NONE',  ( 43.34962307344078880, 60.10051614449766078, -2.184720259617096705 ) ) ;
#4227=CARTESIAN_POINT ( 'NONE',  ( 43.20883090819745576, 48.79948385550240175, 4.963592699179006473 ) ) ;
#4229=CARTESIAN_POINT ( 'NONE',  ( 43.18075615816994173, 57.80051614449766362, 4.924951120819380357 ) ) ;
#4241=CARTESIAN_POINT ( 'NONE',  ( 43.69122665457040000, 52.99948385550241170, 0.02388180880521036456 ) ) ;
#4243=CARTESIAN_POINT ( 'NONE',  ( 54.09612160359786515, 63.69948385550240744, -5.676469297603166098 ) ) ;
#4245=CARTESIAN_POINT ( 'NONE',  ( 42.39856655714564226, 46.10051614449766078, -2.493737253992044156 ) ) ;
#4249=CARTESIAN_POINT ( 'NONE',  ( 45.86712807150329496, 57.70051614449765509, 5.649768623646139964 ) ) ;
#4250=CARTESIAN_POINT ( 'NONE',  ( 48.02776887271745210, 57.39948385550241028, -5.992620115222778487 ) ) ;
#4264=CARTESIAN_POINT ( 'NONE',  ( 45.86712807150323812, 51.29948385550240175, -5.649768623646098220 ) ) ;
#4267=CARTESIAN_POINT ( 'NONE',  ( 55.11794222512599362, 54.80051614449764941, -3.688883143319583446 ) ) ;
#4271=CARTESIAN_POINT ( 'NONE',  ( 44.05948171654949874, 58.79948385550240886, 4.345558710429105354 ) ) ;
#4279=CARTESIAN_POINT ( 'NONE',  ( 42.63976443033212149, 48.99948385550241170, 0.02388180880522514787 ) ) ;
#4280=CARTESIAN_POINT ( 'NONE',  ( 50.02271294988505446, 50.50051614449765935, -7.000000000000000888 ) ) ;
#4282=CARTESIAN_POINT ( 'NONE',  ( 41.58830220609386430, 62.99948385550241170, 0.02388180880523263147 ) ) ;
#4284=CARTESIAN_POINT ( 'NONE',  ( 57.61547081786812896, 56.09948385550240602, 2.450534656007040901 ) ) ;
#4292=CARTESIAN_POINT ( 'NONE',  ( 55.71335778527780036, 48.90051614449766504, -1.832500667257213056 ) ) ;
#4293=CARTESIAN_POINT ( 'NONE',  ( 44.03140696652198471, 59.80051614449766362, 4.306917132069485454 ) ) ;
#4294=CARTESIAN_POINT ( 'NONE',  ( 56.79116909180255135, 45.79948385550240886, -4.963592699179005585 ) ) ;
#4297=CARTESIAN_POINT ( 'NONE',  ( 57.60143344285435774, 55.10051614449765367, 2.493737253992045044 ) ) ;
#4310=CARTESIAN_POINT ( 'NONE',  ( 46.45491332379572924, 47.29948385550241596, -4.840751629271157874 ) ) ;
#4311=CARTESIAN_POINT ( 'NONE',  ( 55.94051828345050836, 63.79948385550240886, -4.345558710429103577 ) ) ;
#4312=CARTESIAN_POINT ( 'NONE',  ( 54.68390685589039890, 47.30051614449766362, 6.485486291978072693 ) ) ;
#4316=CARTESIAN_POINT ( 'NONE',  ( 43.33558569842706021, 57.90051614449766504, 2.141517661632167169 ) ) ;
#4317=CARTESIAN_POINT ( 'NONE',  ( 55.69932041026404335, 57.89948385550241028, -1.875703265242203432 ) ) ;
#4326=CARTESIAN_POINT ( 'NONE',  ( 52.29715082351547295, 52.39948385550241738, 6.992620115222774047 ) ) ;
#4328=CARTESIAN_POINT ( 'NONE',  ( 44.28664221472221385, 51.90051614449765793, 1.832500667257213722 ) ) ;
#4331=CARTESIAN_POINT ( 'NONE',  ( 44.05948171654949874, 62.79948385550241596, 4.345558710429105354 ) ) ;
#4333=CARTESIAN_POINT ( 'NONE',  ( 43.33558569842703179, 59.09948385550240602, -2.141517661632099223 ) ) ;
#4346=CARTESIAN_POINT ( 'NONE',  ( 50.02271294988512551, 50.49948385550240459, 7.000000000000000888 ) ) ;
#4347=CARTESIAN_POINT ( 'NONE',  ( 54.13287192849671214, 48.70051614449766220, -5.649768623646139964 ) ) ;
#4349=CARTESIAN_POINT ( 'NONE',  ( 45.27934281921075410, 65.29948385550241596, -6.458785618021043895 ) ) ;
#4352=CARTESIAN_POINT ( 'NONE',  ( 43.20883090819745576, 54.79948385550240175, 4.963592699179006473 ) ) ;
#4358=CARTESIAN_POINT ( 'NONE',  ( 50.02271294988506156, 48.50051614449765935, -6.000000000000000888 ) ) ;
#4359=CARTESIAN_POINT ( 'NONE',  ( 55.94051828345054389, 61.20051614449765509, 4.345558710429044957 ) ) ;
#4360=CARTESIAN_POINT ( 'NONE',  ( 45.31609314410960820, 64.30051614449766362, -6.485486291978072693 ) ) ;
#4362=CARTESIAN_POINT ( 'NONE',  ( 56.81924384183006538, 56.80051614449764941, -4.924951120819380357 ) ) ;
#4372=CARTESIAN_POINT ( 'NONE',  ( 51.97223112728254790, 48.39948385550240317, 5.992620115222778487 ) ) ;
#4373=CARTESIAN_POINT ( 'NONE',  ( 45.86712807150323812, 65.29948385550241596, -5.649768623646098220 ) ) ;
#4374=CARTESIAN_POINT ( 'NONE',  ( 52.57664461997821093, 45.40051614449765793, 8.007379884777206414 ) ) ;
#4378=CARTESIAN_POINT ( 'NONE',  ( 44.05948171654945611, 54.20051614449764799, -4.345558710429044069 ) ) ;
#4379=CARTESIAN_POINT ( 'NONE',  ( 55.69932041026404335, 61.89948385550241738, -1.875703265242203432 ) ) ;
#4387=CARTESIAN_POINT ( 'NONE',  ( 42.63976443033212860, 48.99948385550240459, 0.02388180880522514787 ) ) ;
#4389=CARTESIAN_POINT ( 'NONE',  ( 48.07319477248762496, 52.40051614449767214, -6.007379884777208190 ) ) ;
#4394=CARTESIAN_POINT ( 'NONE',  ( 56.66441430157296821, 60.09948385550240602, 2.141517661632100111 ) ) ;
#4402=EDGE_LOOP ( 'NONE', ( #12103, #5187, #10037, #11233, #12579, #11690 ) ) ;
#4411=CARTESIAN_POINT ( 'NONE',  ( 54.09612160359786515, 55.69948385550240744, -5.676469297603166098 ) ) ;
#4412=CARTESIAN_POINT ( 'NONE',  ( 54.09612160359792199, 53.30051614449766362, 5.676469297603124353 ) ) ;
#4415=CARTESIAN_POINT ( 'NONE',  ( 52.29715082351547295, 46.39948385550240317, 6.992620115222774047 ) ) ;
#4418=CARTESIAN_POINT ( 'NONE',  ( 47.37792948025162332, 57.39948385550241028, -7.992620115222770494 ) ) ;
#4424=CARTESIAN_POINT ( 'NONE',  ( 55.71335778527780036, 56.90051614449767214, -1.832500667257213056 ) ) ;
#4427=CARTESIAN_POINT ( 'NONE',  ( 42.38452918213188525, 49.09948385550241312, -2.450534656007040013 ) ) ;
#4429=CARTESIAN_POINT ( 'NONE',  ( 43.20883090819742023, 54.20051614449766220, -4.963592699178938972 ) ) ;
#4441=CARTESIAN_POINT ( 'NONE',  ( 56.30877334542961421, 51.99948385550239749, -0.02388180880520959434 ) ) ;
#4442=CARTESIAN_POINT ( 'NONE',  ( 52.25172492374528588, 47.40051614449765793, 7.007379884777204637 ) ) ;
#4443=CARTESIAN_POINT ( 'NONE',  ( 56.81924384183006538, 48.80051614449767072, -4.924951120819380357 ) ) ;
#4446=CARTESIAN_POINT ( 'NONE',  ( 49.97728705011495265, 57.50051614449766646, 7.000000000000000888 ) ) ;
#4447=CARTESIAN_POINT ( 'NONE',  ( 50.02271294988511841, 62.49948385550240459, 6.000000000000000888 ) ) ;
#4458=CARTESIAN_POINT ( 'NONE',  ( 55.94051828345050836, 49.79948385550240175, -4.345558710429104465 ) ) ;
#4460=CARTESIAN_POINT ( 'NONE',  ( 50.02271294988506156, 56.50051614449767357, -6.000000000000000888 ) ) ;
#4464=CARTESIAN_POINT ( 'NONE',  ( 56.66441430157296821, 58.09948385550240602, 2.141517661632100111 ) ) ;
#4477=CARTESIAN_POINT ( 'NONE',  ( 52.29715082351547295, 52.39948385550240317, 6.992620115222774047 ) ) ;
#4479=CARTESIAN_POINT ( 'NONE',  ( 54.13287192849671214, 56.70051614449766220, -5.649768623646139964 ) ) ;
#4481=CARTESIAN_POINT ( 'NONE',  ( 54.13287192849676188, 52.29948385550240886, 5.649768623646098220 ) ) ;
#4482=( LENGTH_UNIT ( ) NAMED_UNIT ( * ) SI_UNIT ( .MILLI., .METRE. ) );
#4484=CARTESIAN_POINT ( 'NONE',  ( 56.81924384183011512, 62.19948385550240744, 4.924951120819313743 ) ) ;
#4491=CARTESIAN_POINT ( 'NONE',  ( 55.69932041026405045, 55.10051614449765367, 1.875703265242156359 ) ) ;
#4493=CARTESIAN_POINT ( 'NONE',  ( 54.68390685589033495, 51.69948385550241454, -6.485486291978119766 ) ) ;
#4494=CARTESIAN_POINT ( 'NONE',  ( 56.66441430157296821, 58.09948385550240602, 2.141517661632100111 ) ) ;
#4496=CARTESIAN_POINT ( 'NONE',  ( 54.72065718078924590, 46.29948385550240886, 6.458785618021043895 ) ) ;
#4503=SHAPE_REPRESENTATION ( 'spring', ( #430 ), #3304 ) ;
#4510=CARTESIAN_POINT ( 'NONE',  ( 55.11794222512601493, 58.19948385550240744, 3.688883143319541702 ) ) ;
#4511=CARTESIAN_POINT ( 'NONE',  ( 54.89903213687075834, 44.74560054925188268, -5.000000000000007105 ) ) ;
#4513=CARTESIAN_POINT ( 'NONE',  ( 56.79116909180259398, 55.20051614449766220, 4.963592699178938972 ) ) ;
#4518=CARTESIAN_POINT ( 'NONE',  ( 42.63976443033212860, 60.00051614449764514, -0.02388180880514948964 ) ) ;
#4525=CARTESIAN_POINT ( 'NONE',  ( 62.49999999999998579, 5.000000000000018652, -5.000000000000000000 ) ) ;
#4528=CARTESIAN_POINT ( 'NONE',  ( 52.25172492374522903, 59.59948385550240602, -7.007379884777225953 ) ) ;
#4531=CARTESIAN_POINT ( 'NONE',  ( 55.11794222512599362, 60.80051614449766362, -3.688883143319583446 ) ) ;
#4534=CARTESIAN_POINT ( 'NONE',  ( 49.97728705011488159, 65.49948385550240459, -7.000000000000000888 ) ) ;
#4535=CARTESIAN_POINT ( 'NONE',  ( 45.90387839640214196, 64.69948385550240744, 5.676469297603166098 ) ) ;
#4548=CARTESIAN_POINT ( 'NONE',  ( 57.36023556966787851, 49.99948385550239749, -0.02388180880522424582 ) ) ;
#4549=CARTESIAN_POINT ( 'NONE',  ( 45.90387839640208512, 52.30051614449766362, -5.676469297603124353 ) ) ;
#4551=CARTESIAN_POINT ( 'NONE',  ( 49.97728705011488159, 53.49948385550240459, -7.000000000000000888 ) ) ;
#4552=CARTESIAN_POINT ( 'NONE',  ( 44.03140696652192787, 47.19948385550240744, -4.306917132069425058 ) ) ;
#4554=CARTESIAN_POINT ( 'NONE',  ( 52.25172492374522903, 45.59948385550240602, -7.007379884777225953 ) ) ;
#4562=CARTESIAN_POINT ( 'NONE',  ( 49.97728705011494554, 53.50051614449767357, 6.000000000000000888 ) ) ;
#4564=CARTESIAN_POINT ( 'NONE',  ( 56.79116909180255135, 51.79948385550240175, -4.963592699179005585 ) ) ;
#4565=CARTESIAN_POINT ( 'NONE',  ( 55.96859303347804371, 54.19948385550240033, 4.306917132069425946 ) ) ;
#4568=CARTESIAN_POINT ( 'NONE',  ( 54.68390685589039890, 61.30051614449766362, 6.485486291978072693 ) ) ;
#4580=CARTESIAN_POINT ( 'NONE',  ( 50.02271294988511841, 56.49948385550240459, 6.000000000000000888 ) ) ;
#4581=CARTESIAN_POINT ( 'NONE',  ( 47.74827507625470702, 46.40051614449765083, -7.007379884777204637 ) ) ;
#4583=CARTESIAN_POINT ( 'NONE',  ( 47.42335538002180328, 50.40051614449766504, -8.007379884777206414 ) ) ;
#4587=CARTESIAN_POINT ( 'NONE',  ( 47.74827507625469281, 64.40051614449765793, -7.007379884777203749 ) ) ;
#4596=CARTESIAN_POINT ( 'NONE',  ( 54.13287192849676188, 60.29948385550240886, 5.649768623646098220 ) ) ;
#4600=CARTESIAN_POINT ( 'NONE',  ( 55.71335778527780036, 58.90051614449766504, -1.832500667257213056 ) ) ;
#4603=CARTESIAN_POINT ( 'NONE',  ( 43.34962307344078880, 46.10051614449766078, -2.184720259617096705 ) ) ;
#4604=CARTESIAN_POINT ( 'NONE',  ( 51.92680522751233951, 47.59948385550239891, -6.007379884777223289 ) ) ;
#4618=CARTESIAN_POINT ( 'NONE',  ( 55.94051828345053679, 53.20051614449766220, 4.345558710429044069 ) ) ;
#4622=CARTESIAN_POINT ( 'NONE',  ( 52.25172492374522903, 51.59948385550240602, -7.007379884777225953 ) ) ;
#4624=CARTESIAN_POINT ( 'NONE',  ( 55.96859303347804371, 48.19948385550240033, 4.306917132069425946 ) ) ;
#4625=CARTESIAN_POINT ( 'NONE',  ( 42.39856655714566358, 60.89948385550241028, 2.493737253992119207 ) ) ;
#4633=CARTESIAN_POINT ( 'NONE',  ( 44.88205777487401349, 53.80051614449766362, 3.688883143319584779 ) ) ;
#4635=CARTESIAN_POINT ( 'NONE',  ( 45.31609314410967926, 52.69948385550240744, 6.485486291978119766 ) ) ;
#4636=CARTESIAN_POINT ( 'NONE',  ( 55.94051828345050836, 57.79948385550238754, -4.345558710429104465 ) ) ;
#4638=CARTESIAN_POINT ( 'NONE',  ( 54.72065718078918906, 62.70051614449766220, -6.458785618021089192 ) ) ;
#4650=CARTESIAN_POINT ( 'NONE',  ( 56.30877334542961421, 53.99948385550241170, -0.02388180880520959434 ) ) ;
#4651=CARTESIAN_POINT ( 'NONE',  ( 56.65037692655921120, 47.10051614449766078, 2.184720259617097593 ) ) ;
#4652=CARTESIAN_POINT ( 'NONE',  ( 43.18075615816994173, 53.80051614449766362, 4.924951120819380357 ) ) ;
#4654=CARTESIAN_POINT ( 'NONE',  ( 52.60990417590917900, 44.99999999999999289, -5.983956152663589378 ) ) ;
#4655=CARTESIAN_POINT ( 'NONE',  ( 42.63976443033212860, 64.00051614449765225, -0.02388180880514948964 ) ) ;
#4665=CARTESIAN_POINT ( 'NONE',  ( 52.29715082351547295, 54.39948385550239607, 6.992620115222774047 ) ) ;
#4666=CARTESIAN_POINT ( 'NONE',  ( 46.45491332379576477, 59.70051614449766220, 4.840751629271188961 ) ) ;
#4669=CARTESIAN_POINT ( 'NONE',  ( 44.28664221472221385, 63.90051614449765793, 1.832500667257213722 ) ) ;
#4670=CARTESIAN_POINT ( 'NONE',  ( 55.69932041026404335, 45.89948385550240317, -1.875703265242203432 ) ) ;
#4672=EDGE_LOOP ( 'NONE', ( #5205, #6815, #8789 ) ) ;
#4687=CARTESIAN_POINT ( 'NONE',  ( 55.96859303347802239, 50.80051614449766362, -4.306917132069484566 ) ) ;
#4691=CARTESIAN_POINT ( 'NONE',  ( 42.63976443033212860, 54.99948385550241170, 0.02388180880522514787 ) ) ;
#4692=CARTESIAN_POINT ( 'NONE',  ( 55.96859303347804371, 46.19948385550238612, 4.306917132069425946 ) ) ;
#4693=CARTESIAN_POINT ( 'NONE',  ( 43.20883090819745576, 60.79948385550241596, 4.963592699179006473 ) ) ;
#4703=CARTESIAN_POINT ( 'NONE',  ( 46.45491332379576477, 55.70051614449766220, 4.840751629271188961 ) ) ;
#4705=CARTESIAN_POINT ( 'NONE',  ( 45.27934281921075410, 51.29948385550240175, -6.458785618021043895 ) ) ;
#4707=CARTESIAN_POINT ( 'NONE',  ( 45.90387839640214196, 58.69948385550240033, 5.676469297603166098 ) ) ;
#4709=CARTESIAN_POINT ( 'NONE',  ( 56.79116909180255135, 45.79948385550240886, -4.963592699179005585 ) ) ;
#4720=CARTESIAN_POINT ( 'NONE',  ( 48.02776887271745210, 55.39948385550240317, -5.992620115222778487 ) ) ;
#4721=CARTESIAN_POINT ( 'NONE',  ( 52.29715082351539479, 46.60051614449766078, -6.992620115222796251 ) ) ;
#4722=CARTESIAN_POINT ( 'NONE',  ( 58.41169779390614281, 53.00051614449765935, 0.02388180880515032231 ) ) ;
#4726=CARTESIAN_POINT ( 'NONE',  ( 56.79116909180259398, 45.20051614449766220, 4.963592699178938972 ) ) ;
#4732=FACE_OUTER_BOUND ( 'NONE', #10721, .T. ) ;
#4735=CARTESIAN_POINT ( 'NONE',  ( 44.05948171654949874, 56.79948385550240886, 4.345558710429105354 ) ) ;
#4736=CARTESIAN_POINT ( 'NONE',  ( 44.30067958973594955, 58.10051614449765367, -1.875703265242155693 ) ) ;
#4740=CARTESIAN_POINT ( 'NONE',  ( 54.09612160359792199, 47.30051614449765651, 5.676469297603124353 ) ) ;
#4741=CARTESIAN_POINT ( 'NONE',  ( 53.54508667620428497, 48.29948385550240175, 4.840751629271157874 ) ) ;
#4755=CARTESIAN_POINT ( 'NONE',  ( 55.96859303347802239, 62.80051614449766362, -4.306917132069484566 ) ) ;
#4758=CARTESIAN_POINT ( 'NONE',  ( 55.94051828345050836, 59.79948385550238754, -4.345558710429104465 ) ) ;
#4760=CARTESIAN_POINT ( 'NONE',  ( 54.09612160359786515, 47.69948385550240744, -5.676469297603166098 ) ) ;
#4762=CARTESIAN_POINT ( 'NONE',  ( 54.68390685589033495, 63.69948385550240033, -6.485486291978119766 ) ) ;
#4770=CARTESIAN_POINT ( 'NONE',  ( 48.07319477248762496, 58.40051614449765793, -6.007379884777208190 ) ) ;
#4772=CARTESIAN_POINT ( 'NONE',  ( 43.20883090819745576, 54.79948385550240175, 4.963592699179006473 ) ) ;
#4773=CARTESIAN_POINT ( 'NONE',  ( 47.74827507625478518, 54.59948385550239180, 7.007379884777227730 ) ) ;
#4775=CARTESIAN_POINT ( 'NONE',  ( 43.18075615816994173, 59.80051614449766362, 4.924951120819380357 ) ) ;
#4788=CARTESIAN_POINT ( 'NONE',  ( 44.88205777487398507, 59.19948385550240744, -3.688883143319540814 ) ) ;
#4789=CARTESIAN_POINT ( 'NONE',  ( 47.74827507625470702, 54.40051614449765793, -7.007379884777204637 ) ) ;
#4790=CARTESIAN_POINT ( 'NONE',  ( 54.72065718078918906, 54.70051614449765509, -6.458785618021089192 ) ) ;
#4794=CARTESIAN_POINT ( 'NONE',  ( 54.13287192849671214, 62.70051614449766220, -5.649768623646139964 ) ) ;
#4801=CARTESIAN_POINT ( 'NONE',  ( 47.70284917648453415, 57.39948385550241028, -6.992620115222774047 ) ) ;
#4802=CARTESIAN_POINT ( 'NONE',  ( 49.97728705011488159, 55.49948385550240459, -7.000000000000000888 ) ) ;
#4807=CARTESIAN_POINT ( 'NONE',  ( 42.63976443033212860, 46.00051614449766646, -0.02388180880514948964 ) ) ;
#4808=CARTESIAN_POINT ( 'NONE',  ( 55.94051828345050836, 63.79948385550240886, -4.345558710429104465 ) ) ;
#4820=CARTESIAN_POINT ( 'NONE',  ( 54.09612160359792199, 63.30051614449766362, 5.676469297603124353 ) ) ;
#4823=CARTESIAN_POINT ( 'NONE',  ( 47.74827507625478518, 56.59948385550238470, 7.007379884777227730 ) ) ;
#4824=CARTESIAN_POINT ( 'NONE',  ( 47.74827507625478518, 46.59948385550239891, 7.007379884777227730 ) ) ;
#4826=CARTESIAN_POINT ( 'NONE',  ( 54.13287192849676188, 46.29948385550240886, 5.649768623646098220 ) ) ;
#4838=CARTESIAN_POINT ( 'NONE',  ( 51.92680522751238925, 63.40051614449765083, 6.007379884777208190 ) ) ;
#4840=CARTESIAN_POINT ( 'NONE',  ( 41.58830220609386430, 58.99948385550239749, 0.02388180880523263147 ) ) ;
#4841=CARTESIAN_POINT ( 'NONE',  ( 52.29715082351547295, 64.39948385550239607, 6.992620115222774047 ) ) ;
#4844=CARTESIAN_POINT ( 'NONE',  ( 47.42335538002188144, 50.59948385550240602, 8.007379884777233059 ) ) ;
#4858=CARTESIAN_POINT ( 'NONE',  ( 48.02776887271745210, 61.39948385550240317, -5.992620115222778487 ) ) ;
#4859=CARTESIAN_POINT ( 'NONE',  ( 56.65037692655921120, 55.10051614449766078, 2.184720259617097593 ) ) ;
#4860=CARTESIAN_POINT ( 'NONE',  ( 52.57664461997821093, 57.40051614449767214, 8.007379884777206414 ) ) ;
#4863=CARTESIAN_POINT ( 'NONE',  ( 50.76502259767569569, 44.99999999999998579, -6.467049654501940914 ) ) ;
#4864=CARTESIAN_POINT ( 'NONE',  ( 57.36023556966787851, 61.00051614449766646, 0.02388180880515038476 ) ) ;
#4874=CARTESIAN_POINT ( 'NONE',  ( 53.54508667620428497, 46.29948385550240886, 4.840751629271157874 ) ) ;
#4875=CARTESIAN_POINT ( 'NONE',  ( 55.94051828345050836, 59.79948385550240175, -4.345558710429103577 ) ) ;
#4882=CARTESIAN_POINT ( 'NONE',  ( 53.54508667620424234, 62.70051614449766220, -4.840751629271188961 ) ) ;
#4883=CARTESIAN_POINT ( 'NONE',  ( 55.11794222512601493, 50.19948385550241454, 3.688883143319541702 ) ) ;
#4892=CARTESIAN_POINT ( 'NONE',  ( 55.94051828345053679, 61.20051614449766220, 4.345558710429044069 ) ) ;
#4894=CARTESIAN_POINT ( 'NONE',  ( 46.45491332379576477, 47.70051614449766220, 4.840751629271188961 ) ) ;
#4896=CARTESIAN_POINT ( 'NONE',  ( 45.86712807150323812, 61.29948385550240886, -5.649768623646098220 ) ) ;
#4897=CARTESIAN_POINT ( 'NONE',  ( 56.65037692655918988, 51.89948385550241028, -2.184720259617163762 ) ) ;
#4900=CARTESIAN_POINT ( 'NONE',  ( 56.65037692655918988, 47.89948385550240317, -2.184720259617163762 ) ) ;
#4911=CARTESIAN_POINT ( 'NONE',  ( 55.08986747509849380, 59.20051614449766220, 3.727524721679155384 ) ) ;
#4913=CARTESIAN_POINT ( 'NONE',  ( 47.42335538002188144, 60.59948385550240602, 8.007379884777233059 ) ) ;
#4915=CARTESIAN_POINT ( 'NONE',  ( 55.94051828345050836, 63.79948385550240886, -4.345558710429104465 ) ) ;
#4917=CARTESIAN_POINT ( 'NONE',  ( 52.62207051974839089, 50.39948385550241738, 7.992620115222770494 ) ) ;
#4929=CARTESIAN_POINT ( 'NONE',  ( 49.97728705011488870, 65.49948385550240459, -6.000000000000000888 ) ) ;
#4930=CARTESIAN_POINT ( 'NONE',  ( 43.34962307344078880, 54.10051614449766788, -2.184720259617096705 ) ) ;
#4931=CARTESIAN_POINT ( 'NONE',  ( 42.39856655714564226, 60.10051614449766788, -2.493737253992044156 ) ) ;
#4936=CARTESIAN_POINT ( 'NONE',  ( 43.18075615816994173, 51.80051614449766362, 4.924951120819380357 ) ) ;
#4947=CARTESIAN_POINT ( 'NONE',  ( 49.97728705011488870, 45.49948385550240459, -6.000000000000000888 ) ) ;
#4948=CARTESIAN_POINT ( 'NONE',  ( 55.96859303347805081, 62.19948385550241454, 4.306917132069425058 ) ) ;
#4953=CARTESIAN_POINT ( 'NONE',  ( 43.34962307344078880, 52.10051614449766078, -2.184720259617096705 ) ) ;
#4954=CARTESIAN_POINT ( 'NONE',  ( 49.97728705011488870, 53.49948385550240459, -6.000000000000000888 ) ) ;
#4964=CARTESIAN_POINT ( 'NONE',  ( 50.02271294988512551, 46.49948385550240459, 7.000000000000000888 ) ) ;
#4967=CARTESIAN_POINT ( 'NONE',  ( 53.50833635130544508, 45.30051614449766362, 4.867452303228181343 ) ) ;
#4970=CARTESIAN_POINT ( 'NONE',  ( 56.66441430157296821, 58.09948385550240602, 2.141517661632100111 ) ) ;
#4971=CARTESIAN_POINT ( 'NONE',  ( 50.02271294988512551, 50.49948385550240459, 7.000000000000000888 ) ) ;
#4974=CARTESIAN_POINT ( 'NONE',  ( 55.94051828345050836, 51.79948385550240175, -4.345558710429104465 ) ) ;
#4978=DIRECTION ( 'NONE',  ( -1.000000000000000000, 0.000000000000000000, 1.224646799147353207E-16 ) ) ;
#4984=CARTESIAN_POINT ( 'NONE',  ( 44.28664221472221385, 59.90051614449767214, 1.832500667257213722 ) ) ;
#4987=CARTESIAN_POINT ( 'NONE',  ( 56.81924384183011512, 58.19948385550240744, 4.924951120819313743 ) ) ;
#4988=CARTESIAN_POINT ( 'NONE',  ( 54.13287192849676188, 64.29948385550241596, 5.649768623646098220 ) ) ;
#4990=CARTESIAN_POINT ( 'NONE',  ( 52.57664461997811856, 49.59948385550241312, -8.007379884777229506 ) ) ;
#4999=CARTESIAN_POINT ( 'NONE',  ( 56.30877334542961421, 59.99948385550241170, -0.02388180880520959434 ) ) ;
#5000=CARTESIAN_POINT ( 'NONE',  ( 44.03140696652198471, 53.80051614449766362, 4.306917132069485454 ) ) ;
#5002=CARTESIAN_POINT ( 'NONE',  ( 50.02271294988505446, 58.50051614449765225, -8.000000000000001776 ) ) ;
#5004=CARTESIAN_POINT ( 'NONE',  ( 42.38452918213190657, 47.90051614449765793, 2.450534656007115508 ) ) ;
#5019=CARTESIAN_POINT ( 'NONE',  ( 44.30067958973596376, 46.89948385550240317, 1.875703265242204099 ) ) ;
#5020=CARTESIAN_POINT ( 'NONE',  ( 49.97728705011488159, 61.49948385550240459, -7.000000000000000888 ) ) ;
#5025=CARTESIAN_POINT ( 'NONE',  ( 45.86712807150329496, 53.70051614449766220, 5.649768623646139964 ) ) ;
#5026=CARTESIAN_POINT ( 'NONE',  ( 44.88205777487398507, 55.19948385550240744, -3.688883143319540814 ) ) ;
#5038=CARTESIAN_POINT ( 'NONE',  ( 46.49166364869456913, 46.30051614449766362, -4.867452303228181343 ) ) ;
#5040=CARTESIAN_POINT ( 'NONE',  ( 57.36023556966787851, 57.99948385550239038, -0.02388180880522424582 ) ) ;
#5041=CARTESIAN_POINT ( 'NONE',  ( 47.70284917648453415, 55.39948385550238896, -6.992620115222774047 ) ) ;
#5043=CARTESIAN_POINT ( 'NONE',  ( 47.74827507625478518, 46.59948385550239891, 7.007379884777227730 ) ) ;
#5052=CARTESIAN_POINT ( 'NONE',  ( 44.91013252490150620, 62.20051614449766220, -3.727524721679154940 ) ) ;
#5055=CARTESIAN_POINT ( 'NONE',  ( 45.27934281921075410, 59.29948385550240886, -6.458785618021043895 ) ) ;
#5057=CARTESIAN_POINT ( 'NONE',  ( 42.38452918213188525, 51.09948385550240602, -2.450534656007040013 ) ) ;
#5062=( GEOMETRIC_REPRESENTATION_CONTEXT ( 3 ) GLOBAL_UNCERTAINTY_ASSIGNED_CONTEXT ( ( #506 ) ) GLOBAL_UNIT_ASSIGNED_CONTEXT ( ( #4482, #11107, #12150 ) ) REPRESENTATION_CONTEXT ( 'NONE', 'WORKASPACE' ) );
#5067=CARTESIAN_POINT ( 'NONE',  ( 44.88205777487398507, 65.19948385550240744, -3.688883143319540814 ) ) ;
#5068=CARTESIAN_POINT ( 'NONE',  ( 50.02271294988505446, 50.50051614449765935, -7.000000000000000888 ) ) ;
#5069=CARTESIAN_POINT ( 'NONE',  ( 49.97728705011495265, 61.50051614449766646, 8.000000000000001776 ) ) ;
#5073=CARTESIAN_POINT ( 'NONE',  ( 41.58830220609386430, 50.00051614449765935, -0.02388180880514929535 ) ) ;
#5087=CARTESIAN_POINT ( 'NONE',  ( 54.13287192849676188, 64.29948385550241596, 5.649768623646098220 ) ) ;
#5088=CARTESIAN_POINT ( 'NONE',  ( 52.29715082351547295, 60.39948385550240317, 6.992620115222774047 ) ) ;
#5093=CARTESIAN_POINT ( 'NONE',  ( 42.63976443033212860, 50.00051614449766646, -0.02388180880514948964 ) ) ;
#5094=CARTESIAN_POINT ( 'NONE',  ( 51.97223112728254790, 52.39948385550241028, 5.992620115222778487 ) ) ;
#5108=CARTESIAN_POINT ( 'NONE',  ( 56.30877334542961421, 45.00051614449765225, 0.02388180880515774693 ) ) ;
#5111=CARTESIAN_POINT ( 'NONE',  ( 54.13287192849676188, 56.29948385550240175, 5.649768623646098220 ) ) ;
#5114=CARTESIAN_POINT ( 'NONE',  ( 52.29715082351547295, 48.39948385550240317, 6.992620115222774047 ) ) ;
#5123=CARTESIAN_POINT ( 'NONE',  ( 50.02271294988512551, 48.49948385550240459, 7.000000000000000888 ) ) ;
#5125=CARTESIAN_POINT ( 'NONE',  ( 49.97728705011495265, 49.50051614449765935, 7.000000000000000888 ) ) ;
#5127=CARTESIAN_POINT ( 'NONE',  ( 43.18075615816989199, 57.19948385550241454, -4.924951120819313743 ) ) ;
#5129=CARTESIAN_POINT ( 'NONE',  ( 58.41169779390614281, 49.99948385550240459, -0.02388180880523160798 ) ) ;
#5142=CARTESIAN_POINT ( 'NONE',  ( 46.49166364869460466, 60.69948385550240033, 4.867452303228209765 ) ) ;
#5143=CARTESIAN_POINT ( 'NONE',  ( 50.02271294988505446, 62.50051614449766646, -7.000000000000000888 ) ) ;
#5144=CARTESIAN_POINT ( 'NONE',  ( 42.38452918213190657, 59.90051614449767214, 2.450534656007115508 ) ) ;
#5148=CARTESIAN_POINT ( 'NONE',  ( 47.42335538002180328, 52.40051614449767214, -8.007379884777206414 ) ) ;
#5154=EDGE_LOOP ( 'NONE', ( #13463, #2133 ) ) ;
#5160=CARTESIAN_POINT ( 'NONE',  ( 45.90387839640214196, 64.69948385550240744, 5.676469297603166098 ) ) ;
#5161=CARTESIAN_POINT ( 'NONE',  ( 54.13287192849676188, 58.29948385550240175, 5.649768623646098220 ) ) ;
#5162=CARTESIAN_POINT ( 'NONE',  ( 45.86712807150329496, 61.70051614449766220, 5.649768623646139964 ) ) ;
#5166=CARTESIAN_POINT ( 'NONE',  ( 49.99999999999997158, 45.00000000000001421, -7.499999999999998224 ) ) ;
#5167=CARTESIAN_POINT ( 'NONE',  ( 43.33558569842706021, 49.90051614449766504, 2.141517661632167169 ) ) ;
#5168=CARTESIAN_POINT ( 'NONE',  ( 55.69932041026404335, 49.89948385550241028, -1.875703265242203432 ) ) ;
#5177=CARTESIAN_POINT ( 'NONE',  ( 54.13287192849676188, 46.29948385550240886, 5.649768623646098220 ) ) ;
#5179=CARTESIAN_POINT ( 'NONE',  ( 46.49166364869456913, 48.30051614449765651, -4.867452303228181343 ) ) ;
#5182=CARTESIAN_POINT ( 'NONE',  ( 44.05948171654949874, 50.79948385550238754, 4.345558710429105354 ) ) ;
#5184=CARTESIAN_POINT ( 'NONE',  ( 52.25172492374522903, 53.59948385550241312, -7.007379884777225953 ) ) ;
#5187=ORIENTED_EDGE ( 'NONE', *, *, #9129, .T. ) ;
#5196=CARTESIAN_POINT ( 'NONE',  ( 49.97728705011495265, 47.50051614449766646, 7.000000000000000888 ) ) ;
#5200=CARTESIAN_POINT ( 'NONE',  ( 43.20883090819745576, 62.79948385550240175, 4.963592699179006473 ) ) ;
#5204=CARTESIAN_POINT ( 'NONE',  ( 57.61547081786812896, 54.09948385550241312, 2.450534656007040901 ) ) ;
#5205=ORIENTED_EDGE ( 'NONE', *, *, #1266, .F. ) ;
#5214=CARTESIAN_POINT ( 'NONE',  ( 55.71335778527780036, 46.90051614449766504, -1.832500667257213056 ) ) ;
#5216=CARTESIAN_POINT ( 'NONE',  ( 54.13287192849671214, 62.70051614449766220, -5.649768623646139964 ) ) ;
#5217=CARTESIAN_POINT ( 'NONE',  ( 57.60143344285433642, 45.89948385550240317, -2.493737253992118319 ) ) ;
#5219=CARTESIAN_POINT ( 'NONE',  ( 45.31609314410960820, 48.30051614449765651, -6.485486291978072693 ) ) ;
#5227=CARTESIAN_POINT ( 'NONE',  ( 49.97728705011488870, 49.49948385550241170, -6.000000000000000888 ) ) ;
#5230=CARTESIAN_POINT ( 'NONE',  ( 57.36023556966787851, 59.00051614449765935, 0.02388180880515038476 ) ) ;
#5234=CARTESIAN_POINT ( 'NONE',  ( 54.09612160359792199, 49.30051614449765651, 5.676469297603124353 ) ) ;
#5235=CARTESIAN_POINT ( 'NONE',  ( 44.28664221472220675, 57.09948385550240602, -1.832500667257165317 ) ) ;
#5240=ORIENTED_EDGE ( 'NONE', *, *, #9129, .F. ) ;
#5247=CARTESIAN_POINT ( 'NONE',  ( 44.28664221472221385, 53.90051614449765793, 1.832500667257213722 ) ) ;
#5249=CARTESIAN_POINT ( 'NONE',  ( 56.65037692655918988, 61.89948385550241028, -2.184720259617163762 ) ) ;
#5250=CARTESIAN_POINT ( 'NONE',  ( 42.63976443033212860, 62.99948385550241170, 0.02388180880522514787 ) ) ;
#5251=CARTESIAN_POINT ( 'NONE',  ( 56.65037692655918988, 61.89948385550241028, -2.184720259617163762 ) ) ;
#5261=CARTESIAN_POINT ( 'NONE',  ( 55.94051828345050836, 47.79948385550240886, -4.345558710429103577 ) ) ;
#5262=CARTESIAN_POINT ( 'NONE',  ( 43.33558569842706021, 47.90051614449765793, 2.141517661632167169 ) ) ;
#5264=CARTESIAN_POINT ( 'NONE',  ( 47.70284917648453415, 47.39948385550238896, -6.992620115222774047 ) ) ;
#5266=CARTESIAN_POINT ( 'NONE',  ( 54.68390685589033495, 55.69948385550240744, -6.485486291978119766 ) ) ;
#5275=CARTESIAN_POINT ( 'NONE',  ( 46.49166364869456913, 50.30051614449766362, -4.867452303228181343 ) ) ;
#5276=CARTESIAN_POINT ( 'NONE',  ( 49.97728705011495265, 59.50051614449765935, 7.000000000000000888 ) ) ;
#5277=CARTESIAN_POINT ( 'NONE',  ( 50.02271294988505446, 64.50051614449766646, -8.000000000000001776 ) ) ;
#5279=CARTESIAN_POINT ( 'NONE',  ( 56.79116909180259398, 59.20051614449766220, 4.963592699178938972 ) ) ;
#5290=CARTESIAN_POINT ( 'NONE',  ( 44.91013252490152752, 52.79948385550240175, 3.727524721679198461 ) ) ;
#5292=CARTESIAN_POINT ( 'NONE',  ( 45.86712807150323812, 63.29948385550240886, -5.649768623646098220 ) ) ;
#5293=CARTESIAN_POINT ( 'NONE',  ( 45.31609314410960820, 48.30051614449765651, -6.485486291978072693 ) ) ;
#5298=CARTESIAN_POINT ( 'NONE',  ( 44.03140696652198471, 55.80051614449766362, 4.306917132069485454 ) ) ;
#5299=CARTESIAN_POINT ( 'NONE',  ( 49.97728705011488870, 61.49948385550241170, -6.000000000000000888 ) ) ;
#5302=( GEOMETRIC_REPRESENTATION_CONTEXT ( 3 ) GLOBAL_UNCERTAINTY_ASSIGNED_CONTEXT ( ( #11728 ) ) GLOBAL_UNIT_ASSIGNED_CONTEXT ( ( #5726, #2594, #5929 ) ) REPRESENTATION_CONTEXT ( 'NONE', 'WORKASPACE' ) );
#5308=CARTESIAN_POINT ( 'NONE',  ( 47.70284917648453415, 51.39948385550238896, -6.992620115222774047 ) ) ;
#5312=CARTESIAN_POINT ( 'NONE',  ( 50.02271294988506156, 52.50051614449766646, -6.000000000000000888 ) ) ;
#5315=CARTESIAN_POINT ( 'NONE',  ( 54.13287192849676188, 62.29948385550240886, 5.649768623646098220 ) ) ;
#5316=CARTESIAN_POINT ( 'NONE',  ( 44.05948171654949874, 62.79948385550241596, 4.345558710429105354 ) ) ;
#5324=CARTESIAN_POINT ( 'NONE',  ( 54.09612160359786515, 47.69948385550240744, -5.676469297603166098 ) ) ;
#5325=CARTESIAN_POINT ( 'NONE',  ( 48.07319477248762496, 64.40051614449764372, -6.007379884777208190 ) ) ;
#5329=CARTESIAN_POINT ( 'NONE',  ( 57.36023556966787851, 47.99948385550239038, -0.02388180880522424582 ) ) ;
#5333=CARTESIAN_POINT ( 'NONE',  ( 52.57664461997811856, 59.59948385550240602, -8.007379884777229506 ) ) ;
#5341=CARTESIAN_POINT ( 'NONE',  ( 49.97728705011494554, 45.50051614449766646, 6.000000000000000888 ) ) ;
#5342=CARTESIAN_POINT ( 'NONE',  ( 54.09612160359792199, 57.30051614449765651, 5.676469297603124353 ) ) ;
#5343=CARTESIAN_POINT ( 'NONE',  ( 45.31609314410967926, 46.69948385550240744, 6.485486291978119766 ) ) ;
#5345=CARTESIAN_POINT ( 'NONE',  ( 56.81924384183006538, 58.80051614449766362, -4.924951120819380357 ) ) ;
#5358=CARTESIAN_POINT ( 'NONE',  ( 50.02271294988511841, 48.49948385550241170, 6.000000000000000888 ) ) ;
#5360=CARTESIAN_POINT ( 'NONE',  ( 57.36023556966787851, 63.99948385550241170, -0.02388180880522424582 ) ) ;
#5362=CARTESIAN_POINT ( 'NONE',  ( 47.42335538002180328, 48.40051614449766504, -8.007379884777206414 ) ) ;
#5366=CARTESIAN_POINT ( 'NONE',  ( 45.86712807150329496, 55.70051614449766220, 5.649768623646139964 ) ) ;
#5367=CARTESIAN_POINT ( 'NONE',  ( 53.50833635130540955, 61.69948385550240744, -4.867452303228209765 ) ) ;
#5377=CARTESIAN_POINT ( 'NONE',  ( 52.25172492374522903, 49.59948385550240602, -7.007379884777225953 ) ) ;
#5378=ADVANCED_FACE ( 'NONE', ( #10997 ), #1016, .T. ) ;
#5380=CARTESIAN_POINT ( 'NONE',  ( 44.30067958973594955, 50.10051614449766078, -1.875703265242155693 ) ) ;
#5384=CARTESIAN_POINT ( 'NONE',  ( 44.05948171654949874, 56.79948385550240886, 4.345558710429105354 ) ) ;
#5397=CARTESIAN_POINT ( 'NONE',  ( 57.36023556966787851, 53.99948385550239749, -0.02388180880522424582 ) ) ;
#5398=CARTESIAN_POINT ( 'NONE',  ( 57.36023556966787851, 47.00051614449764514, 0.02388180880515038476 ) ) ;
#5400=CARTESIAN_POINT ( 'NONE',  ( 52.29715082351547295, 48.39948385550240317, 6.992620115222774047 ) ) ;
#5402=CARTESIAN_POINT ( 'NONE',  ( 50.02271294988513972, 54.49948385550240459, 8.000000000000001776 ) ) ;
#5403=B_SPLINE_CURVE_WITH_KNOTS ( 'NONE', 3,
 ( #2941, #839, #6281, #9437, #2162, #9233 ),
 .UNSPECIFIED., .F., .F.,
 ( 4, 2, 4 ),
 ( 0.0007315534878134838555, 0.001060812114463466869, 0.001390070741113449884 ),
 .UNSPECIFIED. ) ;
#5410=CARTESIAN_POINT ( 'NONE',  ( 56.30877334542961421, 49.00051614449765935, 0.02388180880515774693 ) ) ;
#5411=CARTESIAN_POINT ( 'NONE',  ( 44.03140696652198471, 61.80051614449766362, 4.306917132069485454 ) ) ;
#5413=CARTESIAN_POINT ( 'NONE',  ( 54.68390685589039890, 63.30051614449767072, 6.485486291978072693 ) ) ;
#5416=CARTESIAN_POINT ( 'NONE',  ( 52.62207051974829852, 58.60051614449766788, -7.992620115222797139 ) ) ;
#5430=CARTESIAN_POINT ( 'NONE',  ( 55.08986747509847248, 51.79948385550240175, -3.727524721679197572 ) ) ;
#5432=CARTESIAN_POINT ( 'NONE',  ( 43.20883090819742023, 46.20051614449766220, -4.963592699178938972 ) ) ;
#5435=CARTESIAN_POINT ( 'NONE',  ( 43.33558569842706021, 59.90051614449766504, 2.141517661632167169 ) ) ;
#5436=CARTESIAN_POINT ( 'NONE',  ( 51.92680522751233951, 61.59948385550240602, -6.007379884777223289 ) ) ;
#5447=CARTESIAN_POINT ( 'NONE',  ( 44.03140696652192787, 53.19948385550238612, -4.306917132069425058 ) ) ;
#5449=CARTESIAN_POINT ( 'NONE',  ( 55.08986747509849380, 51.20051614449766220, 3.727524721679155384 ) ) ;
#5453=CARTESIAN_POINT ( 'NONE',  ( 49.97728705011488159, 59.49948385550240459, -7.000000000000000888 ) ) ;
#5463=CARTESIAN_POINT ( 'NONE',  ( 54.13287192849676188, 54.29948385550240886, 5.649768623646098220 ) ) ;
#5464=CARTESIAN_POINT ( 'NONE',  ( 47.74827507625469281, 52.40051614449763662, -7.007379884777203749 ) ) ;
#5466=CARTESIAN_POINT ( 'NONE',  ( 42.39856655714566358, 62.89948385550240317, 2.493737253992119207 ) ) ;
#5468=CARTESIAN_POINT ( 'NONE',  ( 58.41169779390614281, 55.99948385550241170, -0.02388180880523160798 ) ) ;
#5474=CARTESIAN_POINT ( 'NONE',  ( 55.69932041026405045, 45.10051614449766788, 1.875703265242156359 ) ) ;
#5476=CARTESIAN_POINT ( 'NONE',  ( 45.31609314410967926, 48.69948385550241454, 6.485486291978119766 ) ) ;
#5478=CARTESIAN_POINT ( 'NONE',  ( 57.61547081786810764, 56.90051614449767214, -2.450534656007114176 ) ) ;
#5488=CARTESIAN_POINT ( 'NONE',  ( 53.54508667620428497, 52.29948385550240886, 4.840751629271157874 ) ) ;
#5490=CARTESIAN_POINT ( 'NONE',  ( 52.62207051974829852, 44.60051614449766078, -7.992620115222797139 ) ) ;
#5495=CARTESIAN_POINT ( 'NONE',  ( 49.97728705011495265, 59.50051614449765935, 7.000000000000000888 ) ) ;
#5496=CARTESIAN_POINT ( 'NONE',  ( 51.97223112728254790, 56.39948385550241028, 5.992620115222778487 ) ) ;
#5507=CARTESIAN_POINT ( 'NONE',  ( 54.13287192849676188, 48.29948385550240175, 5.649768623646098220 ) ) ;
#5509=CARTESIAN_POINT ( 'NONE',  ( 48.07319477248762496, 50.40051614449766504, -6.007379884777208190 ) ) ;
#5512=CARTESIAN_POINT ( 'NONE',  ( 47.70284917648453415, 61.39948385550241738, -6.992620115222774047 ) ) ;
#5522=CARTESIAN_POINT ( 'NONE',  ( 43.33558569842703179, 51.09948385550240602, -2.141517661632099223 ) ) ;
#5523=CARTESIAN_POINT ( 'NONE',  ( 47.70284917648459100, 51.60051614449765367, 6.992620115222796251 ) ) ;
#5525=CARTESIAN_POINT ( 'NONE',  ( 50.02271294988512551, 54.49948385550240459, 7.000000000000000888 ) ) ;
#5530=CARTESIAN_POINT ( 'NONE',  ( 41.58830220609386430, 64.99948385550240459, 0.02388180880523263147 ) ) ;
#5537=CARTESIAN_POINT ( 'NONE',  ( 44.88205777487401349, 51.80051614449766362, 3.688883143319584779 ) ) ;
#5540=CARTESIAN_POINT ( 'NONE',  ( 56.81924384183011512, 50.19948385550241454, 4.924951120819313743 ) ) ;
#5541=CARTESIAN_POINT ( 'NONE',  ( 55.94051828345050836, 53.79948385550238754, -4.345558710429104465 ) ) ;
#5543=CARTESIAN_POINT ( 'NONE',  ( 42.38452918213190657, 57.90051614449765793, 2.450534656007115508 ) ) ;
#5554=CARTESIAN_POINT ( 'NONE',  ( 48.02776887271745210, 59.39948385550240317, -5.992620115222778487 ) ) ;
#5555=CARTESIAN_POINT ( 'NONE',  ( 57.36023556966787851, 45.00051614449765225, 0.02388180880515038476 ) ) ;
#5556=CARTESIAN_POINT ( 'NONE',  ( 47.37792948025170858, 49.60051614449766788, 7.992620115222797139 ) ) ;
#5561=CARTESIAN_POINT ( 'NONE',  ( 54.13287192849671214, 54.70051614449766220, -5.649768623646139964 ) ) ;
#5562=CARTESIAN_POINT ( 'NONE',  ( 46.49166364869460466, 62.69948385550240744, 4.867452303228209765 ) ) ;
#5567=CIRCLE ( 'NONE', #6020, 0.4999999999999972244 ) ;
#5572=CARTESIAN_POINT ( 'NONE',  ( 56.66441430157296821, 52.09948385550240602, 2.141517661632100111 ) ) ;
#5575=CARTESIAN_POINT ( 'NONE',  ( 46.49166364869456913, 60.30051614449767072, -4.867452303228181343 ) ) ;
#5577=FACE_OUTER_BOUND ( 'NONE', #3870, .T. ) ;
#5579=CARTESIAN_POINT ( 'NONE',  ( 55.08986747509847248, 47.79948385550240886, -3.727524721679197572 ) ) ;
#5592=CARTESIAN_POINT ( 'NONE',  ( 50.02271294988512551, 52.49948385550240459, 7.000000000000000888 ) ) ;
#5594=CARTESIAN_POINT ( 'NONE',  ( 45.86712807150329496, 51.70051614449766220, 5.649768623646139964 ) ) ;
#5596=CARTESIAN_POINT ( 'NONE',  ( 52.29715082351547295, 54.39948385550239607, 6.992620115222774047 ) ) ;
#5598=CARTESIAN_POINT ( 'NONE',  ( 45.31609314410967926, 62.69948385550240744, 6.485486291978119766 ) ) ;
#5607=CARTESIAN_POINT ( 'NONE',  ( 43.69122665457040000, 54.00051614449765935, -0.02388180880515696977 ) ) ;
#5609=CARTESIAN_POINT ( 'NONE',  ( 49.97728705011486738, 55.49948385550241170, -8.000000000000001776 ) ) ;
#5610=CARTESIAN_POINT ( 'NONE',  ( 52.25172492374522903, 57.59948385550241312, -7.007379884777225953 ) ) ;
#5612=CARTESIAN_POINT ( 'NONE',  ( 41.58830220609386430, 60.00051614449765935, -0.02388180880514929535 ) ) ;
#5624=CARTESIAN_POINT ( 'NONE',  ( 53.54508667620428497, 56.29948385550240886, 4.840751629271157874 ) ) ;
#5625=CARTESIAN_POINT ( 'NONE',  ( 50.02271294988505446, 48.50051614449765935, -7.000000000000000888 ) ) ;
#5627=CARTESIAN_POINT ( 'NONE',  ( 57.61547081786810764, 50.90051614449765793, -2.450534656007114176 ) ) ;
#5631=CARTESIAN_POINT ( 'NONE',  ( 52.29715082351538769, 60.60051614449764656, -6.992620115222796251 ) ) ;
#5643=CARTESIAN_POINT ( 'NONE',  ( 45.90387839640214196, 58.69948385550240033, 5.676469297603166098 ) ) ;
#5645=CARTESIAN_POINT ( 'NONE',  ( 55.11794222512599362, 56.80051614449764941, -3.688883143319583446 ) ) ;
#5648=MANIFOLD_SOLID_BREP ( 'Cavity1', #3168 ) ;
#5650=CARTESIAN_POINT ( 'NONE',  ( 49.97728705011488870, 47.49948385550240459, -6.000000000000000888 ) ) ;
#5661=CARTESIAN_POINT ( 'NONE',  ( 43.33558569842706021, 51.90051614449765793, 2.141517661632167169 ) ) ;
#5664=CARTESIAN_POINT ( 'NONE',  ( 52.29715082351547295, 52.39948385550241738, 6.992620115222774047 ) ) ;
#5665=CARTESIAN_POINT ( 'NONE',  ( 42.63976443033212860, 46.99948385550240459, 0.02388180880522514787 ) ) ;
#5667=CARTESIAN_POINT ( 'NONE',  ( 49.97728705011486738, 65.49948385550240459, -8.000000000000001776 ) ) ;
#5676=CARTESIAN_POINT ( 'NONE',  ( 43.69122665457040000, 52.00051614449766646, -0.02388180880515696977 ) ) ;
#5678=CARTESIAN_POINT ( 'NONE',  ( 58.41169779390614281, 55.99948385550241170, -0.02388180880523160798 ) ) ;
#5679=CARTESIAN_POINT ( 'NONE',  ( 47.74827507625478518, 58.59948385550238470, 7.007379884777227730 ) ) ;
#5681=ADVANCED_FACE ( 'NONE', ( #12018 ), #12542, .T. ) ;
#5682=CARTESIAN_POINT ( 'NONE',  ( 45.27934281921082516, 63.70051614449766930, 6.458785618021089192 ) ) ;
#5693=CARTESIAN_POINT ( 'NONE',  ( 53.50833635130540955, 53.69948385550240744, -4.867452303228209765 ) ) ;
#5694=CARTESIAN_POINT ( 'NONE',  ( 55.94051828345054389, 47.20051614449766220, 4.345558710429044957 ) ) ;
#5695=CARTESIAN_POINT ( 'NONE',  ( 43.20883090819742023, 52.20051614449766220, -4.963592699178938972 ) ) ;
#5700=CARTESIAN_POINT ( 'NONE',  ( 52.62207051974829852, 44.60051614449766078, -7.992620115222797139 ) ) ;
#5709=CARTESIAN_POINT ( 'NONE',  ( 47.74827507625478518, 56.59948385550238470, 7.007379884777227730 ) ) ;
#5711=CARTESIAN_POINT ( 'NONE',  ( 48.02776887271750184, 55.60051614449765367, 5.992620115222795363 ) ) ;
#5715=CARTESIAN_POINT ( 'NONE',  ( 43.69122665457040000, 64.00051614449765225, -0.02388180880515696977 ) ) ;
#5716=CARTESIAN_POINT ( 'NONE',  ( 44.05948171654949874, 64.79948385550240175, 4.345558710429105354 ) ) ;
#5719=VECTOR ( 'NONE', #4978, 1000.000000000000000 ) ;
#5726=( LENGTH_UNIT ( ) NAMED_UNIT ( * ) SI_UNIT ( .MILLI., .METRE. ) );
#5729=CARTESIAN_POINT ( 'NONE',  ( 43.34962307344078880, 56.10051614449766078, -2.184720259617096705 ) ) ;
#5732=CARTESIAN_POINT ( 'NONE',  ( 44.05948171654949874, 50.79948385550238754, 4.345558710429105354 ) ) ;
#5734=CARTESIAN_POINT ( 'NONE',  ( 50.02271294988513972, 62.49948385550240459, 8.000000000000001776 ) ) ;
#5739=VERTEX_POINT ( 'NONE', #4534 ) ;
#5743=CARTESIAN_POINT ( 'NONE',  ( 51.97223112728249816, 54.60051614449766788, -5.992620115222793586 ) ) ;
#5746=CARTESIAN_POINT ( 'NONE',  ( 57.60143344285433642, 51.89948385550241028, -2.493737253992118319 ) ) ;
#5748=CARTESIAN_POINT ( 'NONE',  ( 49.97728705011488159, 57.49948385550241170, -7.000000000000000888 ) ) ;
#5750=CARTESIAN_POINT ( 'NONE',  ( 50.02271294988505446, 62.50051614449767357, -8.000000000000001776 ) ) ;
#5763=CARTESIAN_POINT ( 'NONE',  ( 46.49166364869460466, 54.69948385550240033, 4.867452303228209765 ) ) ;
#5764=CARTESIAN_POINT ( 'NONE',  ( 45.86712807150329496, 47.70051614449766220, 5.649768623646139964 ) ) ;
#5765=CARTESIAN_POINT ( 'NONE',  ( 47.37792948025170858, 51.60051614449766788, 7.992620115222797139 ) ) ;
#5769=CARTESIAN_POINT ( 'NONE',  ( 44.03140696652198471, 63.80051614449765651, 4.306917132069485454 ) ) ;
#5781=CARTESIAN_POINT ( 'NONE',  ( 45.90387839640214196, 54.69948385550240744, 5.676469297603166098 ) ) ;
#5782=CARTESIAN_POINT ( 'NONE',  ( 51.92680522751238925, 57.40051614449767214, 6.007379884777208190 ) ) ;
#5786=CARTESIAN_POINT ( 'NONE',  ( 49.97728705011494554, 61.50051614449766646, 6.000000000000000888 ) ) ;
#5787=CARTESIAN_POINT ( 'NONE',  ( 51.92680522751233951, 45.59948385550240602, -6.007379884777223289 ) ) ;
#5799=CARTESIAN_POINT ( 'NONE',  ( 56.66441430157294690, 62.90051614449765083, -2.141517661632166281 ) ) ;
#5803=CARTESIAN_POINT ( 'NONE',  ( 57.36023556966787851, 49.99948385550238328, -0.02388180880522424582 ) ) ;
#5804=CARTESIAN_POINT ( 'NONE',  ( 56.66441430157296821, 46.09948385550240602, 2.141517661632100111 ) ) ;
#5806=CARTESIAN_POINT ( 'NONE',  ( 42.39856655714566358, 62.89948385550240317, 2.493737253992119207 ) ) ;
#5814=CARTESIAN_POINT ( 'NONE',  ( 55.08986747509849380, 55.20051614449766220, 3.727524721679155384 ) ) ;
#5817=CARTESIAN_POINT ( 'NONE',  ( 56.81924384183011512, 54.19948385550241454, 4.924951120819313743 ) ) ;
#5818=CARTESIAN_POINT ( 'NONE',  ( 50.02271294988512551, 58.49948385550241170, 7.000000000000000888 ) ) ;
#5820=CARTESIAN_POINT ( 'NONE',  ( 45.31609314410967926, 46.69948385550240744, 6.485486291978119766 ) ) ;
#5828=CARTESIAN_POINT ( 'NONE',  ( 0.000000000000000000, 0.000000000000000000, 0.000000000000000000 ) ) ;
#5832=CARTESIAN_POINT ( 'NONE',  ( 55.08986747509847248, 55.79948385550239465, -3.727524721679197572 ) ) ;
#5834=CARTESIAN_POINT ( 'NONE',  ( 54.72065718078918906, 52.70051614449766220, -6.458785618021089192 ) ) ;
#5836=CARTESIAN_POINT ( 'NONE',  ( 45.86712807150329496, 63.70051614449766220, 5.649768623646139964 ) ) ;
#5845=CARTESIAN_POINT ( 'NONE',  ( 56.66441430157296821, 58.09948385550240602, 2.141517661632100111 ) ) ;
#5846=CARTESIAN_POINT ( 'NONE',  ( 43.33558569842703179, 53.09948385550240602, -2.141517661632099223 ) ) ;
#5854=CARTESIAN_POINT ( 'NONE',  ( 44.91013252490150620, 64.20051614449766930, -3.727524721679154940 ) ) ;
#5855=CARTESIAN_POINT ( 'NONE',  ( 44.28664221472220675, 47.09948385550240602, -1.832500667257165317 ) ) ;
#5869=CARTESIAN_POINT ( 'NONE',  ( 50.02271294988505446, 58.50051614449765935, -7.000000000000000888 ) ) ;
#5872=CARTESIAN_POINT ( 'NONE',  ( 56.65037692655918988, 59.89948385550241028, -2.184720259617163762 ) ) ;
#5873=CARTESIAN_POINT ( 'NONE',  ( 42.63976443033212860, 46.99948385550240459, 0.02388180880522514787 ) ) ;
#5880=CARTESIAN_POINT ( 'NONE',  ( 56.30877334542961421, 63.00051614449766646, 0.02388180880515774693 ) ) ;
#5883=CARTESIAN_POINT ( 'NONE',  ( 54.72065718078924590, 62.29948385550241596, 6.458785618021043895 ) ) ;
#5884=CARTESIAN_POINT ( 'NONE',  ( 42.63976443033212860, 60.99948385550238328, 0.02388180880522514787 ) ) ;
#5887=CARTESIAN_POINT ( 'NONE',  ( 49.97728705011486738, 45.49948385550240459, -8.000000000000001776 ) ) ;
#5899=CARTESIAN_POINT ( 'NONE',  ( 55.69932041026404335, 63.89948385550240317, -1.875703265242203432 ) ) ;
#5900=CARTESIAN_POINT ( 'NONE',  ( 55.94051828345054389, 53.20051614449766220, 4.345558710429044957 ) ) ;
#5901=CARTESIAN_POINT ( 'NONE',  ( 50.02271294988505446, 54.50051614449765935, -8.000000000000001776 ) ) ;
#5904=CARTESIAN_POINT ( 'NONE',  ( 54.72065718078918906, 46.70051614449766220, -6.458785618021089192 ) ) ;
#5912=CARTESIAN_POINT ( 'NONE',  ( 55.96859303347804371, 64.19948385550239323, 4.306917132069425946 ) ) ;
#5913=ADVANCED_FACE ( 'NONE', ( #12279 ), #9361, .T. ) ;
#5914=CARTESIAN_POINT ( 'NONE',  ( 42.63976443033212149, 60.99948385550239749, 0.02388180880522514787 ) ) ;
#5919=CARTESIAN_POINT ( 'NONE',  ( 51.97223112728249816, 62.60051614449765367, -5.992620115222793586 ) ) ;
#5920=CARTESIAN_POINT ( 'NONE',  ( 48.07319477248768180, 54.59948385550240602, 6.007379884777225953 ) ) ;
#5929=( NAMED_UNIT ( * ) SI_UNIT ( $, .STERADIAN. ) SOLID_ANGLE_UNIT ( ) );
#5932=CARTESIAN_POINT ( 'NONE',  ( 55.94051828345053679, 57.20051614449766930, 4.345558710429044069 ) ) ;
#5934=CARTESIAN_POINT ( 'NONE',  ( 50.02271294988506156, 48.50051614449765935, -6.000000000000000888 ) ) ;
#5936=CARTESIAN_POINT ( 'NONE',  ( 43.34962307344081012, 58.89948385550241028, 2.184720259617164650 ) ) ;
#5941=CARTESIAN_POINT ( 'NONE',  ( 42.63976443033212860, 48.99948385550240459, 0.02388180880522514787 ) ) ;
#5952=CARTESIAN_POINT ( 'NONE',  ( 51.92680522751238925, 61.40051614449765793, 6.007379884777208190 ) ) ;
#5955=CARTESIAN_POINT ( 'NONE',  ( 49.97728705011486738, 59.49948385550240459, -8.000000000000001776 ) ) ;
#5957=CARTESIAN_POINT ( 'NONE',  ( 43.33558569842703179, 61.09948385550240602, -2.141517661632099223 ) ) ;
#5960=CARTESIAN_POINT ( 'NONE',  ( 57.60143344285433642, 47.89948385550240317, -2.493737253992118319 ) ) ;
#5972=CARTESIAN_POINT ( 'NONE',  ( 44.91013252490152752, 62.79948385550240175, 3.727524721679198461 ) ) ;
#5973=CARTESIAN_POINT ( 'NONE',  ( 55.96859303347802239, 50.80051614449766362, -4.306917132069484566 ) ) ;
#5974=CARTESIAN_POINT ( 'NONE',  ( 42.39856655714564226, 58.10051614449765367, -2.493737253992044156 ) ) ;
#5978=CARTESIAN_POINT ( 'NONE',  ( 49.97728705011495265, 47.50051614449765935, 8.000000000000001776 ) ) ;
#5987=CARTESIAN_POINT ( 'NONE',  ( 45.90387839640214196, 60.69948385550240033, 5.676469297603166098 ) ) ;
#5988=CARTESIAN_POINT ( 'NONE',  ( 56.66441430157296821, 62.09948385550239891, 2.141517661632100111 ) ) ;
#5993=CARTESIAN_POINT ( 'NONE',  ( 47.70284917648459100, 45.60051614449765367, 6.992620115222796251 ) ) ;
#5994=CARTESIAN_POINT ( 'NONE',  ( 44.91013252490152752, 52.79948385550240175, 3.727524721679198461 ) ) ;
#6006=CARTESIAN_POINT ( 'NONE',  ( 44.91013252490152752, 64.79948385550240175, 3.727524721679198461 ) ) ;
#6008=CARTESIAN_POINT ( 'NONE',  ( 44.05948171654949874, 56.79948385550240886, 4.345558710429105354 ) ) ;
#6009=CARTESIAN_POINT ( 'NONE',  ( 44.05948171654949874, 52.79948385550240175, 4.345558710429105354 ) ) ;
#6013=CARTESIAN_POINT ( 'NONE',  ( 45.90387839640214196, 46.69948385550240744, 5.676469297603166098 ) ) ;
#6020=AXIS2_PLACEMENT_3D ( 'NONE', #12534, #3269, #903 ) ;
#6026=CARTESIAN_POINT ( 'NONE',  ( 49.97728705011494554, 59.50051614449765935, 6.000000000000000888 ) ) ;
#6028=CARTESIAN_POINT ( 'NONE',  ( 56.81924384183011512, 56.19948385550240744, 4.924951120819313743 ) ) ;
#6029=CARTESIAN_POINT ( 'NONE',  ( 57.36023556966787851, 61.99948385550241170, -0.02388180880522424582 ) ) ;
#6032=ADVANCED_FACE ( 'NONE', ( #5577 ), #3359, .F. ) ;
#6033=CARTESIAN_POINT ( 'NONE',  ( 49.97728705011486738, 47.49948385550240459, -8.000000000000001776 ) ) ;
#6045=CARTESIAN_POINT ( 'NONE',  ( 53.50833635130540955, 63.69948385550240033, -4.867452303228209765 ) ) ;
#6046=CARTESIAN_POINT ( 'NONE',  ( 56.65037692655921120, 51.10051614449766078, 2.184720259617097593 ) ) ;
#6047=CARTESIAN_POINT ( 'NONE',  ( 54.72065718078918906, 58.70051614449765509, -6.458785618021089192 ) ) ;
#6050=CARTESIAN_POINT ( 'NONE',  ( 54.68390685589039890, 51.30051614449765651, 6.485486291978072693 ) ) ;
#6062=CARTESIAN_POINT ( 'NONE',  ( 48.07319477248768180, 46.59948385550239891, 6.007379884777225953 ) ) ;
#6063=CARTESIAN_POINT ( 'NONE',  ( 54.13287192849676188, 56.29948385550240175, 5.649768623646098220 ) ) ;
#6067=CARTESIAN_POINT ( 'NONE',  ( 52.25172492374527877, 53.40051614449765793, 7.007379884777203749 ) ) ;
#6068=CARTESIAN_POINT ( 'NONE',  ( 50.02271294988511841, 54.49948385550240459, 6.000000000000000888 ) ) ;
#6080=CARTESIAN_POINT ( 'NONE',  ( 56.65037692655918988, 45.89948385550240317, -2.184720259617163762 ) ) ;
#6084=CARTESIAN_POINT ( 'NONE',  ( 46.49166364869460466, 64.69948385550240744, 4.867452303228209765 ) ) ;
#6087=CARTESIAN_POINT ( 'NONE',  ( 44.05948171654949874, 58.79948385550240886, 4.345558710429105354 ) ) ;
#6088=CARTESIAN_POINT ( 'NONE',  ( 45.90387839640214196, 54.69948385550240744, 5.676469297603166098 ) ) ;
#6091=CARTESIAN_POINT ( 'NONE',  ( 55.96859303347804371, 52.19948385550240033, 4.306917132069425946 ) ) ;
#6099=CARTESIAN_POINT ( 'NONE',  ( 47.70284917648453415, 49.39948385550239607, -6.992620115222774047 ) ) ;
#6100=CARTESIAN_POINT ( 'NONE',  ( 55.69932041026405045, 63.10051614449766078, 1.875703265242156359 ) ) ;
#6102=CARTESIAN_POINT ( 'NONE',  ( 56.79116909180255135, 57.79948385550240175, -4.963592699179005585 ) ) ;
#6103=CARTESIAN_POINT ( 'NONE',  ( 44.03140696652192787, 63.19948385550240744, -4.306917132069425058 ) ) ;
#6105=CARTESIAN_POINT ( 'NONE',  ( 57.61547081786812896, 48.09948385550240602, 2.450534656007040901 ) ) ;
#6114=CARTESIAN_POINT ( 'NONE',  ( 44.30067958973596376, 64.89948385550239607, 1.875703265242204099 ) ) ;
#6115=CARTESIAN_POINT ( 'NONE',  ( 42.63976443033212149, 52.00051614449765935, -0.02388180880514948964 ) ) ;
#6116=CARTESIAN_POINT ( 'NONE',  ( 52.62207051974829852, 56.60051614449765367, -7.992620115222797139 ) ) ;
#6118=CARTESIAN_POINT ( 'NONE',  ( 42.38452918213190657, 51.90051614449765793, 2.450534656007115508 ) ) ;
#6130=CARTESIAN_POINT ( 'NONE',  ( 55.96859303347804371, 62.19948385550240744, 4.306917132069425946 ) ) ;
#6131=CARTESIAN_POINT ( 'NONE',  ( 43.33558569842703179, 59.09948385550240602, -2.141517661632099223 ) ) ;
#6136=CARTESIAN_POINT ( 'NONE',  ( 54.56344682779376143, 44.99999999999996447, -5.899875555194201482 ) ) ;
#6137=CARTESIAN_POINT ( 'NONE',  ( 45.86712807150329496, 49.70051614449766220, 5.649768623646139964 ) ) ;
#6138=CARTESIAN_POINT ( 'NONE',  ( 46.49166364869460466, 52.69948385550240744, 4.867452303228209765 ) ) ;
#6151=CARTESIAN_POINT ( 'NONE',  ( 48.07319477248762496, 46.40051614449765793, -6.007379884777208190 ) ) ;
#6153=CARTESIAN_POINT ( 'NONE',  ( 55.94051828345050836, 55.79948385550238044, -4.345558710429104465 ) ) ;
#6154=CARTESIAN_POINT ( 'NONE',  ( 55.94051828345050836, 55.79948385550238044, -4.345558710429104465 ) ) ;
#6156=CARTESIAN_POINT ( 'NONE',  ( 49.97728705011488159, 47.49948385550240459, -7.000000000000000888 ) ) ;
#6163=CARTESIAN_POINT ( 'NONE',  ( 54.13287192849676188, 46.29948385550240886, 5.649768623646098220 ) ) ;
#6164=CARTESIAN_POINT ( 'NONE',  ( 47.74827507625469281, 48.40051614449764372, -7.007379884777203749 ) ) ;
#6167=CARTESIAN_POINT ( 'NONE',  ( 56.81924384183011512, 60.19948385550240744, 4.924951120819313743 ) ) ;
#6169=CARTESIAN_POINT ( 'NONE',  ( 43.18075615816989199, 47.19948385550240744, -4.924951120819313743 ) ) ;
#6182=CARTESIAN_POINT ( 'NONE',  ( 53.54508667620424234, 44.70051614449765509, -4.840751629271188961 ) ) ;
#6183=CARTESIAN_POINT ( 'NONE',  ( 55.94051828345054389, 51.20051614449765509, 4.345558710429044957 ) ) ;
#6184=CARTESIAN_POINT ( 'NONE',  ( 50.02271294988505446, 60.50051614449766646, -8.000000000000001776 ) ) ;
#6187=CARTESIAN_POINT ( 'NONE',  ( 56.79116909180259398, 51.20051614449766220, 4.963592699178938972 ) ) ;
#6198=CARTESIAN_POINT ( 'NONE',  ( 50.02271294988512551, 62.49948385550240459, 7.000000000000000888 ) ) ;
#6199=CARTESIAN_POINT ( 'NONE',  ( 56.65037692655918988, 57.89948385550240317, -2.184720259617163762 ) ) ;
#6201=CARTESIAN_POINT ( 'NONE',  ( 50.02271294988505446, 60.50051614449765935, -7.000000000000000888 ) ) ;
#6206=CARTESIAN_POINT ( 'NONE',  ( 47.74827507625469281, 52.40051614449763662, -7.007379884777203749 ) ) ;
#6207=CARTESIAN_POINT ( 'NONE',  ( 43.69122665457040000, 54.99948385550239749, 0.02388180880521036456 ) ) ;
#6223=CARTESIAN_POINT ( 'NONE',  ( 55.96859303347804371, 46.19948385550238612, 4.306917132069425946 ) ) ;
#6227=CARTESIAN_POINT ( 'NONE',  ( 44.30067958973596376, 64.89948385550239607, 1.875703265242204099 ) ) ;
#6228=CARTESIAN_POINT ( 'NONE',  ( 56.66441430157296821, 64.09948385550239891, 2.141517661632100111 ) ) ;
#6229=CARTESIAN_POINT ( 'NONE',  ( 50.02271294988512551, 54.49948385550240459, 7.000000000000000888 ) ) ;
#6231=CARTESIAN_POINT ( 'NONE',  ( 45.90387839640214196, 52.69948385550240033, 5.676469297603166098 ) ) ;
#6239=CARTESIAN_POINT ( 'NONE',  ( 55.94051828345050836, 45.79948385550240886, -4.345558710429103577 ) ) ;
#6241=CARTESIAN_POINT ( 'NONE',  ( 50.02271294988506156, 64.50051614449766646, -6.000000000000000888 ) ) ;
#6243=CARTESIAN_POINT ( 'NONE',  ( 55.96859303347804371, 48.19948385550240033, 4.306917132069425946 ) ) ;
#6244=PLANE ( 'NONE',  #6698 ) ;
#6245=CARTESIAN_POINT ( 'NONE',  ( 54.68390685589033495, 49.69948385550240744, -6.485486291978119766 ) ) ;
#6257=CARTESIAN_POINT ( 'NONE',  ( 46.45491332379576477, 45.70051614449766220, 4.840751629271188961 ) ) ;
#6258=CARTESIAN_POINT ( 'NONE',  ( 56.66441430157294690, 58.90051614449766504, -2.141517661632166281 ) ) ;
#6259=CARTESIAN_POINT ( 'NONE',  ( 54.68390685589039890, 61.30051614449766362, 6.485486291978072693 ) ) ;
#6262=CARTESIAN_POINT ( 'NONE',  ( 43.20883090819742023, 52.20051614449766220, -4.963592699178938972 ) ) ;
#6271=CARTESIAN_POINT ( 'NONE',  ( 50.02271294988511841, 50.49948385550239749, 6.000000000000000888 ) ) ;
#6274=CARTESIAN_POINT ( 'NONE',  ( 57.36023556966787851, 61.00051614449766646, 0.02388180880515038476 ) ) ;
#6279=CARTESIAN_POINT ( 'NONE',  ( 44.03140696652198471, 49.80051614449766362, 4.306917132069485454 ) ) ;
#6280=CARTESIAN_POINT ( 'NONE',  ( 55.11794222512601493, 58.19948385550240744, 3.688883143319541702 ) ) ;
#6281=CARTESIAN_POINT ( 'NONE',  ( 55.11928596558036020, 44.77036257738321012, -5.000000000000000888 ) ) ;
#6292=CARTESIAN_POINT ( 'NONE',  ( 51.92680522751238925, 51.40051614449767214, 6.007379884777208190 ) ) ;
#6295=CARTESIAN_POINT ( 'NONE',  ( 47.70284917648453415, 65.39948385550239607, -6.992620115222774047 ) ) ;
#6296=CARTESIAN_POINT ( 'NONE',  ( 44.03140696652192787, 61.19948385550239323, -4.306917132069425058 ) ) ;
#6306=CARTESIAN_POINT ( 'NONE',  ( 43.34962307344078880, 50.10051614449766078, -2.184720259617096705 ) ) ;
#6310=CARTESIAN_POINT ( 'NONE',  ( 56.79116909180255135, 63.79948385550241596, -4.963592699179005585 ) ) ;
#6311=CARTESIAN_POINT ( 'NONE',  ( 50.02271294988505446, 44.50051614449765935, -7.000000000000000888 ) ) ;
#6313=CARTESIAN_POINT ( 'NONE',  ( 58.41169779390614281, 57.99948385550241170, -0.02388180880523160798 ) ) ;
#6322=CARTESIAN_POINT ( 'NONE',  ( 56.30877334542961421, 51.00051614449765935, 0.02388180880515774693 ) ) ;
#6323=CARTESIAN_POINT ( 'NONE',  ( 54.13287192849671214, 58.70051614449765509, -5.649768623646139964 ) ) ;
#6324=CARTESIAN_POINT ( 'NONE',  ( 54.68390685589033495, 47.69948385550240744, -6.485486291978119766 ) ) ;
#6327=CARTESIAN_POINT ( 'NONE',  ( 41.58830220609386430, 54.00051614449765935, -0.02388180880514929535 ) ) ;
#6335=CARTESIAN_POINT ( 'NONE',  ( 46.45491332379572924, 51.29948385550240175, -4.840751629271157874 ) ) ;
#6337=CARTESIAN_POINT ( 'NONE',  ( 56.79116909180259398, 49.20051614449766220, 4.963592699178938972 ) ) ;
#6342=CARTESIAN_POINT ( 'NONE',  ( 44.05948171654945611, 56.20051614449764799, -4.345558710429044069 ) ) ;
#6343=CARTESIAN_POINT ( 'NONE',  ( 51.92680522751233951, 59.59948385550240602, -6.007379884777223289 ) ) ;
#6355=CARTESIAN_POINT ( 'NONE',  ( 50.02271294988512551, 48.49948385550240459, 7.000000000000000888 ) ) ;
#6357=CARTESIAN_POINT ( 'NONE',  ( 48.07319477248762496, 54.40051614449765793, -6.007379884777208190 ) ) ;
#6359=CARTESIAN_POINT ( 'NONE',  ( 55.96859303347804371, 64.19948385550239323, 4.306917132069425946 ) ) ;
#6360=CARTESIAN_POINT ( 'NONE',  ( 45.90387839640214196, 64.69948385550240744, 5.676469297603166098 ) ) ;
#6361=CARTESIAN_POINT ( 'NONE',  ( 52.29715082351547295, 62.39948385550239607, 6.992620115222774047 ) ) ;
#6368=CARTESIAN_POINT ( 'NONE',  ( 47.70284917648453415, 47.39948385550239607, -6.992620115222774047 ) ) ;
#6369=CARTESIAN_POINT ( 'NONE',  ( 44.05948171654945611, 48.20051614449764799, -4.345558710429044069 ) ) ;
#6372=CARTESIAN_POINT ( 'NONE',  ( 56.65037692655918988, 45.89948385550240317, -2.184720259617163762 ) ) ;
#6374=CARTESIAN_POINT ( 'NONE',  ( 52.62207051974839089, 58.39948385550241028, 7.992620115222770494 ) ) ;
#6384=CARTESIAN_POINT ( 'NONE',  ( 55.08986747509849380, 45.20051614449766220, 3.727524721679155384 ) ) ;
#6385=CARTESIAN_POINT ( 'NONE',  ( 45.90387839640208512, 60.30051614449766362, -5.676469297603124353 ) ) ;
#6386=CARTESIAN_POINT ( 'NONE',  ( 43.18075615816994173, 63.80051614449766362, 4.924951120819380357 ) ) ;
#6388=CARTESIAN_POINT ( 'NONE',  ( 52.57664461997821093, 57.40051614449767214, 8.007379884777206414 ) ) ;
#6400=CARTESIAN_POINT ( 'NONE',  ( 55.08986747509847248, 47.79948385550240886, -3.727524721679197572 ) ) ;
#6403=CARTESIAN_POINT ( 'NONE',  ( 52.57664461997821093, 47.40051614449765793, 8.007379884777206414 ) ) ;
#6408=CARTESIAN_POINT ( 'NONE',  ( 52.25172492374527877, 59.40051614449765083, 7.007379884777203749 ) ) ;
#6409=CARTESIAN_POINT ( 'NONE',  ( 55.69932041026404335, 59.89948385550240317, -1.875703265242203432 ) ) ;
#6417=CARTESIAN_POINT ( 'NONE',  ( 56.66441430157296821, 54.09948385550240602, 2.141517661632100111 ) ) ;
#6418=CARTESIAN_POINT ( 'NONE',  ( 43.20883090819745576, 58.79948385550240175, 4.963592699179006473 ) ) ;
#6422=CARTESIAN_POINT ( 'NONE',  ( 44.88205777487401349, 51.80051614449766362, 3.688883143319584779 ) ) ;
#6424=CARTESIAN_POINT ( 'NONE',  ( 54.13287192849676188, 64.29948385550241596, 5.649768623646098220 ) ) ;
#6426=CARTESIAN_POINT ( 'NONE',  ( 43.34962307344081012, 60.89948385550241028, 2.184720259617164650 ) ) ;
#6434=CARTESIAN_POINT ( 'NONE',  ( 47.74827507625477807, 50.59948385550239891, 7.007379884777229506 ) ) ;
#6435=CARTESIAN_POINT ( 'NONE',  ( 47.70284917648459100, 45.60051614449765367, 6.992620115222796251 ) ) ;
#6437=CARTESIAN_POINT ( 'NONE',  ( 54.68390685589033495, 63.69948385550240033, -6.485486291978119766 ) ) ;
#6439=CARTESIAN_POINT ( 'NONE',  ( 42.39856655714566358, 54.89948385550240317, 2.493737253992119207 ) ) ;
#6447=CARTESIAN_POINT ( 'NONE',  ( 44.88205777487401349, 45.80051614449766362, 3.688883143319584779 ) ) ;
#6448=CARTESIAN_POINT ( 'NONE',  ( 52.29715082351539479, 60.60051614449764656, -6.992620115222796251 ) ) ;
#6450=CARTESIAN_POINT ( 'NONE',  ( 49.97728705011486738, 45.49948385550240459, -8.000000000000001776 ) ) ;
#6451=EDGE_CURVE ( 'NONE', #9726, #9705, #2637, .T. ) ;
#6454=CARTESIAN_POINT ( 'NONE',  ( 42.38452918213190657, 53.90051614449765793, 2.450534656007115508 ) ) ;
#6465=CARTESIAN_POINT ( 'NONE',  ( 48.02776887271745210, 51.39948385550241028, -5.992620115222778487 ) ) ;
#6467=CARTESIAN_POINT ( 'NONE',  ( 49.97728705011488159, 65.49948385550240459, -7.000000000000000888 ) ) ;
#6468=CARTESIAN_POINT ( 'NONE',  ( 47.74827507625469281, 64.40051614449765793, -7.007379884777203749 ) ) ;
#6471=CARTESIAN_POINT ( 'NONE',  ( 55.94051828345053679, 55.20051614449766930, 4.345558710429044069 ) ) ;
#6472=CARTESIAN_POINT ( 'NONE',  ( 44.91013252490152752, 60.79948385550241596, 3.727524721679198461 ) ) ;
#6484=CARTESIAN_POINT ( 'NONE',  ( 44.05948171654949874, 52.79948385550240175, 4.345558710429105354 ) ) ;
#6486=CARTESIAN_POINT ( 'NONE',  ( 55.08986747509849380, 49.20051614449766220, 3.727524721679155384 ) ) ;
#6491=CARTESIAN_POINT ( 'NONE',  ( 45.90387839640214196, 58.69948385550240033, 5.676469297603166098 ) ) ;
#6503=CARTESIAN_POINT ( 'NONE',  ( 44.03140696652193498, 55.19948385550240744, -4.306917132069424170 ) ) ;
#6504=CARTESIAN_POINT ( 'NONE',  ( 55.94051828345053679, 55.20051614449766930, 4.345558710429044069 ) ) ;
#6506=CARTESIAN_POINT ( 'NONE',  ( 45.90387839640214196, 48.69948385550240744, 5.676469297603166098 ) ) ;
#6508=CARTESIAN_POINT ( 'NONE',  ( 57.60143344285433642, 55.89948385550241028, -2.493737253992118319 ) ) ;
#6515=CARTESIAN_POINT ( 'NONE',  ( 48.02776887271750184, 47.60051614449766078, 5.992620115222795363 ) ) ;
#6518=CARTESIAN_POINT ( 'NONE',  ( 47.42335538002188144, 48.59948385550239891, 8.007379884777233059 ) ) ;
#6521=CARTESIAN_POINT ( 'NONE',  ( 42.38452918213190657, 55.90051614449766504, 2.450534656007115508 ) ) ;
#6531=CARTESIAN_POINT ( 'NONE',  ( 55.69932041026404335, 49.89948385550241028, -1.875703265242203432 ) ) ;
#6533=CARTESIAN_POINT ( 'NONE',  ( 47.37792948025170858, 45.60051614449765367, 7.992620115222797139 ) ) ;
#6536=CARTESIAN_POINT ( 'NONE',  ( 55.96859303347802239, 56.80051614449764230, -4.306917132069484566 ) ) ;
#6537=CARTESIAN_POINT ( 'NONE',  ( 44.30067958973596376, 58.89948385550241028, 1.875703265242204099 ) ) ;
#6547=CARTESIAN_POINT ( 'NONE',  ( 47.74827507625478518, 48.59948385550239180, 7.007379884777227730 ) ) ;
#6550=CARTESIAN_POINT ( 'NONE',  ( 44.91013252490150620, 50.20051614449766220, -3.727524721679154940 ) ) ;
#6553=CARTESIAN_POINT ( 'NONE',  ( 57.36023556966787851, 61.99948385550241170, -0.02388180880522424582 ) ) ;
#6563=CARTESIAN_POINT ( 'NONE',  ( 54.09612160359786515, 49.69948385550240744, -5.676469297603166098 ) ) ;
#6564=CARTESIAN_POINT ( 'NONE',  ( 52.29715082351538769, 56.60051614449766788, -6.992620115222796251 ) ) ;
#6567=CARTESIAN_POINT ( 'NONE',  ( 47.70284917648453415, 53.39948385550238186, -6.992620115222774047 ) ) ;
#6570=CARTESIAN_POINT ( 'NONE',  ( 58.41169779390614281, 63.99948385550241170, -0.02388180880523160798 ) ) ;
#6576=CARTESIAN_POINT ( 'NONE',  ( 48.02776887271750184, 51.60051614449766788, 5.992620115222795363 ) ) ;
#6577=CARTESIAN_POINT ( 'NONE',  ( 56.65037692655921120, 63.10051614449766078, 2.184720259617097593 ) ) ;
#6578=CARTESIAN_POINT ( 'NONE',  ( 42.39856655714566358, 54.89948385550240317, 2.493737253992119207 ) ) ;
#6579=CARTESIAN_POINT ( 'NONE',  ( 44.03140696652192787, 55.19948385550238612, -4.306917132069425058 ) ) ;
#6581=CARTESIAN_POINT ( 'NONE',  ( 47.37792948025170858, 57.60051614449765367, 7.992620115222797139 ) ) ;
#6592=CARTESIAN_POINT ( 'NONE',  ( 55.08986747509847248, 53.79948385550241596, -3.727524721679197572 ) ) ;
#6593=CARTESIAN_POINT ( 'NONE',  ( 49.97728705011495265, 49.50051614449765935, 7.000000000000000888 ) ) ;
#6594=CARTESIAN_POINT ( 'NONE',  ( 52.57664461997821093, 49.40051614449766504, 8.007379884777206414 ) ) ;
#6597=CARTESIAN_POINT ( 'NONE',  ( 47.74827507625469281, 56.40051614449766504, -7.007379884777203749 ) ) ;
#6598=CARTESIAN_POINT ( 'NONE',  ( 51.97223112728254790, 62.39948385550240317, 5.992620115222778487 ) ) ;
#6607=CARTESIAN_POINT ( 'NONE',  ( 56.66441430157296821, 50.09948385550240602, 2.141517661632100111 ) ) ;
#6609=CARTESIAN_POINT ( 'NONE',  ( 55.11794222512599362, 58.80051614449766362, -3.688883143319583446 ) ) ;
#6612=COLOUR_RGB ( '',0.8941176470588234615, 0.8941176470588234615, 0.8941176470588234615 ) ;
#6615=CARTESIAN_POINT ( 'NONE',  ( 48.07319477248768180, 46.59948385550239891, 6.007379884777225953 ) ) ;
#6631=CARTESIAN_POINT ( 'NONE',  ( 54.09612160359786515, 51.69948385550240744, -5.676469297603166098 ) ) ;
#6632=CARTESIAN_POINT ( 'NONE',  ( 45.86712807150329496, 53.70051614449766220, 5.649768623646139964 ) ) ;
#6635=CARTESIAN_POINT ( 'NONE',  ( 55.96859303347804371, 50.19948385550240744, 4.306917132069425946 ) ) ;
#6638=CARTESIAN_POINT ( 'NONE',  ( 54.72065718078924590, 62.29948385550241596, 6.458785618021043895 ) ) ;
#6647=CARTESIAN_POINT ( 'NONE',  ( 44.30067958973594955, 56.10051614449766078, -1.875703265242155693 ) ) ;
#6650=CARTESIAN_POINT ( 'NONE',  ( 58.41169779390614281, 51.99948385550239749, -0.02388180880523160798 ) ) ;
#6651=CARTESIAN_POINT ( 'NONE',  ( 57.36023556966787851, 59.99948385550240459, -0.02388180880522424582 ) ) ;
#6653=CARTESIAN_POINT ( 'NONE',  ( 54.72065718078918906, 60.70051614449766930, -6.458785618021089192 ) ) ;
#6662=CARTESIAN_POINT ( 'NONE',  ( 51.92680522751233951, 55.59948385550240602, -6.007379884777223289 ) ) ;
#6664=CARTESIAN_POINT ( 'NONE',  ( 43.20883090819742023, 54.20051614449766220, -4.963592699178938972 ) ) ;
#6668=CARTESIAN_POINT ( 'NONE',  ( 52.25172492374527877, 63.40051614449765793, 7.007379884777203749 ) ) ;
#6679=CARTESIAN_POINT ( 'NONE',  ( 52.25172492374522903, 57.59948385550241312, -7.007379884777225953 ) ) ;
#6681=CARTESIAN_POINT ( 'NONE',  ( 55.08986747509849380, 59.20051614449766220, 3.727524721679155384 ) ) ;
#6685=CARTESIAN_POINT ( 'NONE',  ( 42.63976443033212860, 64.99948385550240459, 0.02388180880522514787 ) ) ;
#6698=AXIS2_PLACEMENT_3D ( 'NONE', #13392, #2903, #11190 ) ;
#6699=CARTESIAN_POINT ( 'NONE',  ( 56.65037692655921120, 51.10051614449766078, 2.184720259617097593 ) ) ;
#6702=CARTESIAN_POINT ( 'NONE',  ( 56.65037692655918988, 49.89948385550240317, -2.184720259617163762 ) ) ;
#6703=CARTESIAN_POINT ( 'NONE',  ( 56.65037692655918988, 45.89948385550240317, -2.184720259617163762 ) ) ;
#6704=CIRCLE ( 'NONE', #334, 0.4999999999999972244 ) ;
#6705=CARTESIAN_POINT ( 'NONE',  ( 54.72065718078924590, 64.29948385550240175, 6.458785618021043895 ) ) ;
#6712=CARTESIAN_POINT ( 'NONE',  ( 51.97223112728249816, 56.60051614449765367, -5.992620115222793586 ) ) ;
#6715=CARTESIAN_POINT ( 'NONE',  ( 54.68390685589033495, 55.69948385550240744, -6.485486291978119766 ) ) ;
#6717=CARTESIAN_POINT ( 'NONE',  ( 57.36023556966787851, 55.99948385550239038, -0.02388180880522424582 ) ) ;
#6720=CARTESIAN_POINT ( 'NONE',  ( 45.31609314410960820, 60.30051614449767072, -6.485486291978072693 ) ) ;
#6729=CARTESIAN_POINT ( 'NONE',  ( 53.54508667620428497, 58.29948385550240886, 4.840751629271157874 ) ) ;
#6731=CARTESIAN_POINT ( 'NONE',  ( 45.27934281921082516, 51.70051614449765509, 6.458785618021089192 ) ) ;
#6735=CARTESIAN_POINT ( 'NONE',  ( 49.97728705011495265, 45.50051614449766646, 8.000000000000001776 ) ) ;
#6744=CARTESIAN_POINT ( 'NONE',  ( 42.63976443033212860, 58.99948385550239038, 0.02388180880522514787 ) ) ;
#6746=CARTESIAN_POINT ( 'NONE',  ( 44.30067958973594955, 60.10051614449766788, -1.875703265242155693 ) ) ;
#6749=CARTESIAN_POINT ( 'NONE',  ( 44.88205777487401349, 63.80051614449766362, 3.688883143319584779 ) ) ;
#6750=CARTESIAN_POINT ( 'NONE',  ( 46.49166364869460466, 46.69948385550240744, 4.867452303228209765 ) ) ;
#6762=CARTESIAN_POINT ( 'NONE',  ( 44.03140696652198471, 55.80051614449766362, 4.306917132069485454 ) ) ;
#6764=CARTESIAN_POINT ( 'NONE',  ( 55.94051828345050836, 51.79948385550240175, -4.345558710429104465 ) ) ;
#6765=CARTESIAN_POINT ( 'NONE',  ( 55.94051828345050836, 47.79948385550240886, -4.345558710429104465 ) ) ;
#6767=CARTESIAN_POINT ( 'NONE',  ( 45.31609314410967926, 64.69948385550240744, 6.485486291978119766 ) ) ;
#6776=CARTESIAN_POINT ( 'NONE',  ( 44.28664221472221385, 53.90051614449765793, 1.832500667257213722 ) ) ;
#6778=CARTESIAN_POINT ( 'NONE',  ( 50.02271294988513972, 52.49948385550241170, 8.000000000000001776 ) ) ;
#6779=CARTESIAN_POINT ( 'NONE',  ( 45.90387839640214196, 56.69948385550240744, 5.676469297603166098 ) ) ;
#6782=CARTESIAN_POINT ( 'NONE',  ( 42.38452918213190657, 59.90051614449767214, 2.450534656007115508 ) ) ;
#6794=CARTESIAN_POINT ( 'NONE',  ( 51.97223112728254790, 54.39948385550241028, 5.992620115222778487 ) ) ;
#6796=CARTESIAN_POINT ( 'NONE',  ( 49.97728705011495265, 53.50051614449767357, 8.000000000000001776 ) ) ;
#6798=CARTESIAN_POINT ( 'NONE',  ( 51.51576781266200555, 45.00000000000000711, -6.337576802645323859 ) ) ;
#6799=CARTESIAN_POINT ( 'NONE',  ( 47.74827507625469281, 62.40051614449766504, -7.007379884777203749 ) ) ;
#6806=CARTESIAN_POINT ( 'NONE',  ( 49.97728705011488159, 55.49948385550240459, -7.000000000000000888 ) ) ;
#6809=CARTESIAN_POINT ( 'NONE',  ( 55.08986747509849380, 61.20051614449766220, 3.727524721679155384 ) ) ;
#6812=CARTESIAN_POINT ( 'NONE',  ( 50.02271294988505446, 44.50051614449765935, -7.000000000000000888 ) ) ;
#6813=CARTESIAN_POINT ( 'NONE',  ( 44.30067958973596376, 48.89948385550241028, 1.875703265242204099 ) ) ;
#6815=ORIENTED_EDGE ( 'NONE', *, *, #8305, .F. ) ;
#6824=CARTESIAN_POINT ( 'NONE',  ( 43.34962307344078880, 62.10051614449766078, -2.184720259617096705 ) ) ;
#6828=CARTESIAN_POINT ( 'NONE',  ( 55.94051828345050836, 53.79948385550238754, -4.345558710429104465 ) ) ;
#6829=CARTESIAN_POINT ( 'NONE',  ( 47.74827507625478518, 48.59948385550239180, 7.007379884777227730 ) ) ;
#6831=CARTESIAN_POINT ( 'NONE',  ( 45.31609314410967926, 60.69948385550240033, 6.485486291978119766 ) ) ;
#6839=CARTESIAN_POINT ( 'NONE',  ( 44.28664221472221385, 51.90051614449765793, 1.832500667257213722 ) ) ;
#6842=CARTESIAN_POINT ( 'NONE',  ( 47.37792948025162332, 53.39948385550241028, -7.992620115222770494 ) ) ;
#6844=CARTESIAN_POINT ( 'NONE',  ( 42.63976443033212860, 58.99948385550239038, 0.02388180880522514787 ) ) ;
#6847=CARTESIAN_POINT ( 'NONE',  ( 58.41169779390614281, 61.00051614449765935, 0.02388180880515032231 ) ) ;
#6857=LINE ( 'NONE', #11061, #10303 ) ;
#6858=CARTESIAN_POINT ( 'NONE',  ( 50.02271294988511841, 58.49948385550241170, 6.000000000000000888 ) ) ;
#6859=CARTESIAN_POINT ( 'NONE',  ( 55.96859303347802239, 48.80051614449765651, -4.306917132069484566 ) ) ;
#6861=CARTESIAN_POINT ( 'NONE',  ( 56.81924384183006538, 52.80051614449766362, -4.924951120819380357 ) ) ;
#6865=CARTESIAN_POINT ( 'NONE',  ( 45.90387839640208512, 62.30051614449766362, -5.676469297603124353 ) ) ;
#6874=CARTESIAN_POINT ( 'NONE',  ( 56.66441430157296821, 56.09948385550240602, 2.141517661632100111 ) ) ;
#6875=CARTESIAN_POINT ( 'NONE',  ( 56.66441430157296821, 50.09948385550240602, 2.141517661632100111 ) ) ;
#6876=CARTESIAN_POINT ( 'NONE',  ( 48.02776887271750184, 59.60051614449765367, 5.992620115222795363 ) ) ;
#6879=CARTESIAN_POINT ( 'NONE',  ( 52.29715082351538769, 46.60051614449766078, -6.992620115222796251 ) ) ;
#6880=CARTESIAN_POINT ( 'NONE',  ( 44.03140696652192787, 65.19948385550240744, -4.306917132069425058 ) ) ;
#6897=CARTESIAN_POINT ( 'NONE',  ( 49.97728705011495265, 57.50051614449766646, 7.000000000000000888 ) ) ;
#6901=CARTESIAN_POINT ( 'NONE',  ( 49.97728705011488159, 57.49948385550241170, -7.000000000000000888 ) ) ;
#6902=CARTESIAN_POINT ( 'NONE',  ( 42.63976443033212860, 48.99948385550240459, 0.02388180880522514787 ) ) ;
#6903=CARTESIAN_POINT ( 'NONE',  ( 56.66441430157296821, 46.09948385550240602, 2.141517661632100111 ) ) ;
#6911=CARTESIAN_POINT ( 'NONE',  ( 48.07319477248762496, 62.40051614449765793, -6.007379884777208190 ) ) ;
#6914=CARTESIAN_POINT ( 'NONE',  ( 52.57664461997811856, 57.59948385550240602, -8.007379884777229506 ) ) ;
#6915=CARTESIAN_POINT ( 'NONE',  ( 43.33558569842703179, 65.09948385550239891, -2.141517661632099223 ) ) ;
#6917=CARTESIAN_POINT ( 'NONE',  ( 56.81924384183006538, 62.80051614449766362, -4.924951120819380357 ) ) ;
#6928=CARTESIAN_POINT ( 'NONE',  ( 56.30877334542961421, 63.99948385550241170, -0.02388180880520959434 ) ) ;
#6929=CARTESIAN_POINT ( 'NONE',  ( 44.05948171654945611, 52.20051614449765509, -4.345558710429044069 ) ) ;
#6930=CARTESIAN_POINT ( 'NONE',  ( 52.62207051974829852, 52.60051614449765367, -7.992620115222797139 ) ) ;
#6934=CARTESIAN_POINT ( 'NONE',  ( 55.96859303347802239, 62.80051614449766362, -4.306917132069484566 ) ) ;
#6944=CARTESIAN_POINT ( 'NONE',  ( 47.70284917648453415, 59.39948385550241028, -6.992620115222774047 ) ) ;
#6945=CARTESIAN_POINT ( 'NONE',  ( 47.74827507625477807, 58.59948385550239180, 7.007379884777229506 ) ) ;
#6952=CARTESIAN_POINT ( 'NONE',  ( 55.69932041026405045, 63.10051614449766078, 1.875703265242156359 ) ) ;
#6953=CARTESIAN_POINT ( 'NONE',  ( 53.50833635130540955, 53.69948385550240744, -4.867452303228209765 ) ) ;
#6968=CARTESIAN_POINT ( 'NONE',  ( 44.05948171654945611, 60.20051614449764799, -4.345558710429044069 ) ) ;
#6970=CARTESIAN_POINT ( 'NONE',  ( 51.97223112728249816, 46.60051614449764656, -5.992620115222793586 ) ) ;
#6972=CARTESIAN_POINT ( 'NONE',  ( 52.25172492374522903, 55.59948385550241312, -7.007379884777225953 ) ) ;
#6973=CARTESIAN_POINT ( 'NONE',  ( 57.36023556966787851, 45.99948385550238328, -0.02388180880522424582 ) ) ;
#6974=CARTESIAN_POINT ( 'NONE',  ( 47.74827507625478518, 48.59948385550239180, 7.007379884777227730 ) ) ;
#6981=CARTESIAN_POINT ( 'NONE',  ( 49.97728705011494554, 63.50051614449765935, 6.000000000000000888 ) ) ;
#6983=CARTESIAN_POINT ( 'NONE',  ( 45.27934281921075410, 61.29948385550240886, -6.458785618021043895 ) ) ;
#6986=CARTESIAN_POINT ( 'NONE',  ( 54.68390685589033495, 47.69948385550240744, -6.485486291978119766 ) ) ;
#6999=CARTESIAN_POINT ( 'NONE',  ( 49.97728705011488870, 61.49948385550241170, -6.000000000000000888 ) ) ;
#7000=CARTESIAN_POINT ( 'NONE',  ( 45.86712807150329496, 55.70051614449766220, 5.649768623646139964 ) ) ;
#7001=CARTESIAN_POINT ( 'NONE',  ( 58.41169779390614281, 61.00051614449765935, 0.02388180880515032231 ) ) ;
#7004=CARTESIAN_POINT ( 'NONE',  ( 57.61547081786810764, 48.90051614449766504, -2.450534656007114176 ) ) ;
#7011=CARTESIAN_POINT ( 'NONE',  ( 44.05948171654949874, 64.79948385550240175, 4.345558710429105354 ) ) ;
#7012=CARTESIAN_POINT ( 'NONE',  ( 47.74827507625477807, 56.59948385550240602, 7.007379884777229506 ) ) ;
#7016=CARTESIAN_POINT ( 'NONE',  ( 49.97728705011494554, 63.50051614449765935, 6.000000000000000888 ) ) ;
#7017=CARTESIAN_POINT ( 'NONE',  ( 51.92680522751233951, 53.59948385550240602, -6.007379884777223289 ) ) ;
#7027=FILL_AREA_STYLE ('',( #7999 ) ) ;
#7032=CARTESIAN_POINT ( 'NONE',  ( 44.30067958973594955, 46.10051614449766078, -1.875703265242155693 ) ) ;
#7035=CARTESIAN_POINT ( 'NONE',  ( 54.09612160359786515, 57.69948385550240744, -5.676469297603166098 ) ) ;
#7036=CARTESIAN_POINT ( 'NONE',  ( 52.25172492374522903, 51.59948385550240602, -7.007379884777225953 ) ) ;
#7040=CARTESIAN_POINT ( 'NONE',  ( 55.94051828345050836, 49.79948385550240175, -4.345558710429104465 ) ) ;
#7049=CARTESIAN_POINT ( 'NONE',  ( 46.49166364869456913, 60.30051614449767072, -4.867452303228181343 ) ) ;
#7052=CARTESIAN_POINT ( 'NONE',  ( 45.31609314410967926, 58.69948385550240033, 6.485486291978119766 ) ) ;
#7056=CARTESIAN_POINT ( 'NONE',  ( 52.57664461997811856, 51.59948385550240602, -8.007379884777229506 ) ) ;
#7067=CARTESIAN_POINT ( 'NONE',  ( 55.69932041026404335, 61.89948385550241738, -1.875703265242203432 ) ) ;
#7068=CARTESIAN_POINT ( 'NONE',  ( 50.02271294988505446, 54.50051614449765935, -7.000000000000000888 ) ) ;
#7069=CARTESIAN_POINT ( 'NONE',  ( 57.60143344285435774, 57.10051614449766788, 2.493737253992045044 ) ) ;
#7073=CARTESIAN_POINT ( 'NONE',  ( 56.79116909180259398, 53.20051614449766220, 4.963592699178938972 ) ) ;
#7084=CARTESIAN_POINT ( 'NONE',  ( 42.63976443033212860, 62.99948385550241170, 0.02388180880522514787 ) ) ;
#7085=CARTESIAN_POINT ( 'NONE',  ( 56.66441430157296821, 60.09948385550240602, 2.141517661632100111 ) ) ;
#7090=CARTESIAN_POINT ( 'NONE',  ( 52.25172492374527877, 49.40051614449766504, 7.007379884777203749 ) ) ;
#7091=CARTESIAN_POINT ( 'NONE',  ( 51.97223112728254790, 54.39948385550241028, 5.992620115222778487 ) ) ;
#7100=CARTESIAN_POINT ( 'NONE',  ( 44.03140696652192787, 47.19948385550240744, -4.306917132069425058 ) ) ;
#7104=CARTESIAN_POINT ( 'NONE',  ( 48.02776887271750184, 47.60051614449766078, 5.992620115222795363 ) ) ;
#7106=CARTESIAN_POINT ( 'NONE',  ( 55.94051828345050836, 57.79948385550238754, -4.345558710429104465 ) ) ;
#7107=CARTESIAN_POINT ( 'NONE',  ( 54.09612160359786515, 53.69948385550240744, -5.676469297603166098 ) ) ;
#7111=CARTESIAN_POINT ( 'NONE',  ( 49.97728705011488159, 51.49948385550240459, -7.000000000000000888 ) ) ;
#7123=CARTESIAN_POINT ( 'NONE',  ( 53.54508667620424234, 58.70051614449765509, -4.840751629271188961 ) ) ;
#7125=CARTESIAN_POINT ( 'NONE',  ( 54.68390685589033495, 61.69948385550240744, -6.485486291978119766 ) ) ;
#7126=CARTESIAN_POINT ( 'NONE',  ( 44.03140696652192787, 61.19948385550239323, -4.306917132069425058 ) ) ;
#7128=CARTESIAN_POINT ( 'NONE',  ( 41.58830220609386430, 52.99948385550241170, 0.02388180880523263147 ) ) ;
#7140=CARTESIAN_POINT ( 'NONE',  ( 44.30067958973596376, 62.89948385550240317, 1.875703265242204099 ) ) ;
#7142=CARTESIAN_POINT ( 'NONE',  ( 44.03140696652198471, 51.80051614449766362, 4.306917132069485454 ) ) ;
#7143=CARTESIAN_POINT ( 'NONE',  ( 58.41169779390614281, 59.00051614449766646, 0.02388180880515032231 ) ) ;
#7146=CARTESIAN_POINT ( 'NONE',  ( 45.27934281921082516, 49.70051614449766220, 6.458785618021089192 ) ) ;
#7157=CARTESIAN_POINT ( 'NONE',  ( 43.34962307344081012, 60.89948385550241028, 2.184720259617164650 ) ) ;
#7158=CARTESIAN_POINT ( 'NONE',  ( 43.34962307344081012, 56.89948385550240317, 2.184720259617164650 ) ) ;
#7163=CARTESIAN_POINT ( 'NONE',  ( 42.63976443033212860, 48.00051614449766646, -0.02388180880514948964 ) ) ;
#7164=CARTESIAN_POINT ( 'NONE',  ( 46.45491332379572924, 55.29948385550240175, -4.840751629271157874 ) ) ;
#7179=CARTESIAN_POINT ( 'NONE',  ( 44.28664221472221385, 47.90051614449765793, 1.832500667257213722 ) ) ;
#7182=CARTESIAN_POINT ( 'NONE',  ( 45.90387839640214196, 56.69948385550240744, 5.676469297603166098 ) ) ;
#7183=CARTESIAN_POINT ( 'NONE',  ( 57.36023556966787851, 53.99948385550239038, -0.02388180880522424582 ) ) ;
#7187=CARTESIAN_POINT ( 'NONE',  ( 47.70284917648453415, 47.39948385550238896, -6.992620115222774047 ) ) ;
#7195=CARTESIAN_POINT ( 'NONE',  ( 55.96859303347805081, 48.19948385550240744, 4.306917132069425058 ) ) ;
#7196=CARTESIAN_POINT ( 'NONE',  ( 44.28664221472221385, 63.90051614449765793, 1.832500667257213722 ) ) ;
#7199=CARTESIAN_POINT ( 'NONE',  ( 57.61547081786812896, 60.09948385550240602, 2.450534656007040901 ) ) ;
#7201=CARTESIAN_POINT ( 'NONE',  ( 57.60143344285433642, 49.89948385550241028, -2.493737253992118319 ) ) ;
#7204=VERTEX_POINT ( 'NONE', #1476 ) ;
#7210=CARTESIAN_POINT ( 'NONE',  ( 43.69122665457040000, 60.99948385550241170, 0.02388180880521036456 ) ) ;
#7211=CARTESIAN_POINT ( 'NONE',  ( 50.02271294988505446, 56.50051614449766646, -7.000000000000000888 ) ) ;
#7213=CARTESIAN_POINT ( 'NONE',  ( 45.31609314410960820, 60.30051614449767072, -6.485486291978072693 ) ) ;
#7216=CARTESIAN_POINT ( 'NONE',  ( 47.42335538002180328, 50.40051614449766504, -8.007379884777206414 ) ) ;
#7229=CARTESIAN_POINT ( 'NONE',  ( 45.86712807150323812, 63.29948385550240886, -5.649768623646098220 ) ) ;
#7230=CARTESIAN_POINT ( 'NONE',  ( 50.02271294988512551, 60.49948385550240459, 7.000000000000000888 ) ) ;
#7231=CARTESIAN_POINT ( 'NONE',  ( 44.03140696652198471, 57.80051614449766362, 4.306917132069485454 ) ) ;
#7235=CARTESIAN_POINT ( 'NONE',  ( 44.03140696652198471, 53.80051614449766362, 4.306917132069485454 ) ) ;
#7236=CARTESIAN_POINT ( 'NONE',  ( 44.30067958973596376, 50.89948385550240317, 1.875703265242204099 ) ) ;
#7247=CARTESIAN_POINT ( 'NONE',  ( 56.30877334542961421, 47.00051614449766646, 0.02388180880515774693 ) ) ;
#7249=CARTESIAN_POINT ( 'NONE',  ( 54.09612160359786515, 61.69948385550240744, -5.676469297603166098 ) ) ;
#7250=CARTESIAN_POINT ( 'NONE',  ( 56.66441430157296821, 52.09948385550240602, 2.141517661632100111 ) ) ;
#7253=CARTESIAN_POINT ( 'NONE',  ( 43.34962307344081012, 52.89948385550240317, 2.184720259617164650 ) ) ;
#7261=CARTESIAN_POINT ( 'NONE',  ( 52.25172492374527877, 47.40051614449766504, 7.007379884777203749 ) ) ;
#7265=CARTESIAN_POINT ( 'NONE',  ( 54.09612160359786515, 47.69948385550240744, -5.676469297603166098 ) ) ;
#7268=CARTESIAN_POINT ( 'NONE',  ( 47.37792948025162332, 47.39948385550241028, -7.992620115222770494 ) ) ;
#7279=CARTESIAN_POINT ( 'NONE',  ( 55.69932041026405045, 51.10051614449766078, 1.875703265242156359 ) ) ;
#7280=CARTESIAN_POINT ( 'NONE',  ( 56.65037692655921120, 57.10051614449766078, 2.184720259617097593 ) ) ;
#7282=CARTESIAN_POINT ( 'NONE',  ( 43.18075615816994173, 59.80051614449766362, 4.924951120819380357 ) ) ;
#7285=CARTESIAN_POINT ( 'NONE',  ( 52.57664461997821093, 51.40051614449767214, 8.007379884777206414 ) ) ;
#7300=CARTESIAN_POINT ( 'NONE',  ( 56.65037692655918988, 63.89948385550239607, -2.184720259617163762 ) ) ;
#7303=CARTESIAN_POINT ( 'NONE',  ( 49.97728705011495265, 59.50051614449765935, 7.000000000000000888 ) ) ;
#7307=CARTESIAN_POINT ( 'NONE',  ( 43.34962307344078880, 48.10051614449766078, -2.184720259617096705 ) ) ;
#7308=CARTESIAN_POINT ( 'NONE',  ( 55.08986747509847248, 61.79948385550240175, -3.727524721679197572 ) ) ;
#7320=CARTESIAN_POINT ( 'NONE',  ( 44.05948171654949874, 46.79948385550238754, 4.345558710429105354 ) ) ;
#7323=CARTESIAN_POINT ( 'NONE',  ( 49.97728705011494554, 49.50051614449766646, 6.000000000000000888 ) ) ;
#7325=CARTESIAN_POINT ( 'NONE',  ( 57.36023556966787851, 61.99948385550241170, -0.02388180880522424582 ) ) ;
#7326=CARTESIAN_POINT ( 'NONE',  ( 44.03140696652192787, 55.19948385550238612, -4.306917132069425058 ) ) ;
#7334=CARTESIAN_POINT ( 'NONE',  ( 56.66441430157296821, 46.09948385550240602, 2.141517661632100111 ) ) ;
#7336=CARTESIAN_POINT ( 'NONE',  ( 55.94051828345053679, 47.20051614449766220, 4.345558710429044069 ) ) ;
#7338=CARTESIAN_POINT ( 'NONE',  ( 47.74827507625478518, 46.59948385550239891, 7.007379884777227730 ) ) ;
#7340=CARTESIAN_POINT ( 'NONE',  ( 43.20883090819745576, 56.79948385550240175, 4.963592699179006473 ) ) ;
#7351=CARTESIAN_POINT ( 'NONE',  ( 44.28664221472221385, 49.90051614449766504, 1.832500667257213722 ) ) ;
#7352=CARTESIAN_POINT ( 'NONE',  ( 47.70284917648459810, 59.60051614449765367, 6.992620115222797139 ) ) ;
#7353=CARTESIAN_POINT ( 'NONE',  ( 58.41169779390614281, 47.99948385550239038, -0.02388180880523160798 ) ) ;
#7356=CARTESIAN_POINT ( 'NONE',  ( 57.60143344285435774, 59.10051614449766078, 2.493737253992045044 ) ) ;
#7367=CARTESIAN_POINT ( 'NONE',  ( 53.54508667620428497, 50.29948385550240886, 4.840751629271157874 ) ) ;
#7369=CARTESIAN_POINT ( 'NONE',  ( 52.62207051974829852, 48.60051614449766788, -7.992620115222797139 ) ) ;
#7373=CARTESIAN_POINT ( 'NONE',  ( 57.36023556966787851, 49.00051614449763804, 0.02388180880515038476 ) ) ;
#7374=CARTESIAN_POINT ( 'NONE',  ( 44.88205777487398507, 57.19948385550241454, -3.688883143319540814 ) ) ;
#7383=CARTESIAN_POINT ( 'NONE',  ( 55.96859303347804371, 52.19948385550240033, 4.306917132069425946 ) ) ;
#7385=CARTESIAN_POINT ( 'NONE',  ( 46.49166364869456913, 54.30051614449765651, -4.867452303228181343 ) ) ;
#7387=CARTESIAN_POINT ( 'NONE',  ( 56.66441430157296821, 62.09948385550239891, 2.141517661632100111 ) ) ;
#7388=CARTESIAN_POINT ( 'NONE',  ( 56.66441430157296821, 64.09948385550239891, 2.141517661632100111 ) ) ;
#7389=CARTESIAN_POINT ( 'NONE',  ( 57.36023556966787851, 57.99948385550239038, -0.02388180880522424582 ) ) ;
#7399=CARTESIAN_POINT ( 'NONE',  ( 57.36023556966787851, 45.99948385550239749, -0.02388180880522424582 ) ) ;
#7401=CARTESIAN_POINT ( 'NONE',  ( 44.03140696652198471, 47.80051614449764230, 4.306917132069485454 ) ) ;
#7404=CARTESIAN_POINT ( 'NONE',  ( 49.97728705011486738, 65.49948385550240459, -8.000000000000001776 ) ) ;
#7408=CARTESIAN_POINT ( 'NONE',  ( 57.60143344285433642, 57.89948385550241028, -2.493737253992118319 ) ) ;
#7418=CARTESIAN_POINT ( 'NONE',  ( 44.88205777487401349, 49.80051614449765651, 3.688883143319584779 ) ) ;
#7419=CARTESIAN_POINT ( 'NONE',  ( 57.36023556966787851, 59.00051614449765935, 0.02388180880515038476 ) ) ;
#7420=CARTESIAN_POINT ( 'NONE',  ( 49.97728705011486738, 49.49948385550241170, -8.000000000000001776 ) ) ;
#7422=CARTESIAN_POINT ( 'NONE',  ( 49.97728705011495265, 59.50051614449765935, 8.000000000000001776 ) ) ;
#7431=CARTESIAN_POINT ( 'NONE',  ( 56.30877334542961421, 47.99948385550239038, -0.02388180880520959434 ) ) ;
#7433=CARTESIAN_POINT ( 'NONE',  ( 44.05948171654945611, 64.20051614449765509, -4.345558710429044069 ) ) ;
#7437=CARTESIAN_POINT ( 'NONE',  ( 55.96859303347802239, 58.80051614449764941, -4.306917132069484566 ) ) ;
#7438=CARTESIAN_POINT ( 'NONE',  ( 51.92680522751233951, 57.59948385550240602, -6.007379884777223289 ) ) ;
#7447=CARTESIAN_POINT ( 'NONE',  ( 50.02271294988512551, 52.49948385550240459, 7.000000000000000888 ) ) ;
#7449=CARTESIAN_POINT ( 'NONE',  ( 53.50833635130544508, 49.30051614449766362, 4.867452303228181343 ) ) ;
#7452=CARTESIAN_POINT ( 'NONE',  ( 42.63976443033212860, 62.99948385550241170, 0.02388180880522514787 ) ) ;
#7454=CARTESIAN_POINT ( 'NONE',  ( 45.86712807150323812, 59.29948385550240175, -5.649768623646098220 ) ) ;
#7465=CARTESIAN_POINT ( 'NONE',  ( 52.29715082351538769, 48.60051614449766788, -6.992620115222796251 ) ) ;
#7468=CARTESIAN_POINT ( 'NONE',  ( 52.62207051974839089, 64.39948385550239607, 7.992620115222770494 ) ) ;
#7470=CARTESIAN_POINT ( 'NONE',  ( 49.97728705011486738, 57.49948385550241170, -8.000000000000001776 ) ) ;
#7477=CARTESIAN_POINT ( 'NONE',  ( 53.50833635130544508, 45.30051614449766362, 4.867452303228181343 ) ) ;
#7479=CARTESIAN_POINT ( 'NONE',  ( 44.05948171654945611, 58.20051614449764799, -4.345558710429044069 ) ) ;
#7480=CARTESIAN_POINT ( 'NONE',  ( 56.79116909180255135, 47.79948385550240886, -4.963592699179005585 ) ) ;
#7482=CARTESIAN_POINT ( 'NONE',  ( 47.37792948025170858, 59.60051614449765367, 7.992620115222797139 ) ) ;
#7492=CARTESIAN_POINT ( 'NONE',  ( 51.92680522751233951, 47.59948385550239891, -6.007379884777223289 ) ) ;
#7494=CARTESIAN_POINT ( 'NONE',  ( 43.34962307344081012, 62.89948385550241028, 2.184720259617164650 ) ) ;
#7495=CARTESIAN_POINT ( 'NONE',  ( 57.60143344285435774, 47.10051614449766078, 2.493737253992045044 ) ) ;
#7499=CARTESIAN_POINT ( 'NONE',  ( 57.36023556966787851, 59.00051614449765935, 0.02388180880515038476 ) ) ;
#7500=CARTESIAN_POINT ( 'NONE',  ( 53.54508667620428497, 60.29948385550240175, 4.840751629271157874 ) ) ;
#7509=CARTESIAN_POINT ( 'NONE',  ( 57.36023556966787851, 47.99948385550239038, -0.02388180880522424582 ) ) ;
#7513=CARTESIAN_POINT ( 'NONE',  ( 55.69932041026405045, 49.10051614449766788, 1.875703265242156359 ) ) ;
#7517=CARTESIAN_POINT ( 'NONE',  ( 45.90387839640214196, 56.69948385550240744, 5.676469297603166098 ) ) ;
#7529=CARTESIAN_POINT ( 'NONE',  ( 56.65037692655918988, 51.89948385550241028, -2.184720259617163762 ) ) ;
#7530=CARTESIAN_POINT ( 'NONE',  ( 54.13287192849671214, 46.70051614449766220, -5.649768623646139964 ) ) ;
#7532=CARTESIAN_POINT ( 'NONE',  ( 43.20883090819745576, 64.79948385550240175, 4.963592699179006473 ) ) ;
#7535=CARTESIAN_POINT ( 'NONE',  ( 43.18075615816989199, 55.19948385550240744, -4.924951120819313743 ) ) ;
#7541=CARTESIAN_POINT ( 'NONE',  ( 51.97223112728249816, 50.60051614449765367, -5.992620115222793586 ) ) ;
#7542=CARTESIAN_POINT ( 'NONE',  ( 42.63976443033212149, 62.00051614449765225, -0.02388180880514948964 ) ) ;
#7543=CARTESIAN_POINT ( 'NONE',  ( 56.81924384183011512, 46.19948385550240744, 4.924951120819313743 ) ) ;
#7545=CARTESIAN_POINT ( 'NONE',  ( 54.72065718078918906, 54.70051614449765509, -6.458785618021089192 ) ) ;
#7562=CARTESIAN_POINT ( 'NONE',  ( 53.50833635130540955, 51.69948385550241454, -4.867452303228209765 ) ) ;
#7563=CARTESIAN_POINT ( 'NONE',  ( 49.97728705011488159, 63.49948385550241170, -7.000000000000000888 ) ) ;
#7564=CARTESIAN_POINT ( 'NONE',  ( 45.27934281921082516, 47.70051614449766220, 6.458785618021089192 ) ) ;
#7567=CARTESIAN_POINT ( 'NONE',  ( 52.25172492374527877, 57.40051614449765083, 7.007379884777203749 ) ) ;
#7568=CARTESIAN_POINT ( 'NONE',  ( 46.49166364869460466, 56.69948385550240744, 4.867452303228209765 ) ) ;
#7577=CARTESIAN_POINT ( 'NONE',  ( 55.96859303347804371, 54.19948385550240033, 4.306917132069425946 ) ) ;
#7581=CARTESIAN_POINT ( 'NONE',  ( 55.69932041026405045, 51.10051614449766078, 1.875703265242156359 ) ) ;
#7585=CARTESIAN_POINT ( 'NONE',  ( 55.94051828345050836, 59.79948385550238754, -4.345558710429104465 ) ) ;
#7598=CARTESIAN_POINT ( 'NONE',  ( 44.05948171654949874, 52.79948385550240175, 4.345558710429104465 ) ) ;
#7599=CARTESIAN_POINT ( 'NONE',  ( 43.34962307344078880, 54.10051614449766788, -2.184720259617096705 ) ) ;
#7601=CARTESIAN_POINT ( 'NONE',  ( 43.33558569842703179, 51.09948385550240602, -2.141517661632099223 ) ) ;
#7602=CARTESIAN_POINT ( 'NONE',  ( 43.18075615816989199, 59.19948385550240744, -4.924951120819313743 ) ) ;
#7611=CARTESIAN_POINT ( 'NONE',  ( 56.30877334542961421, 57.00051614449766646, 0.02388180880515774693 ) ) ;
#7614=CARTESIAN_POINT ( 'NONE',  ( 58.41169779390614281, 63.00051614449766646, 0.02388180880515032231 ) ) ;
#7617=CARTESIAN_POINT ( 'NONE',  ( 54.68390685589039890, 57.30051614449767072, 6.485486291978072693 ) ) ;
#7628=CARTESIAN_POINT ( 'NONE',  ( 46.49166364869460466, 52.69948385550240744, 4.867452303228209765 ) ) ;
#7629=CARTESIAN_POINT ( 'NONE',  ( 55.94051828345054389, 49.20051614449766220, 4.345558710429044957 ) ) ;
#7632=CARTESIAN_POINT ( 'NONE',  ( 57.60143344285435774, 49.10051614449766788, 2.493737253992045044 ) ) ;
#7636=CARTESIAN_POINT ( 'NONE',  ( 43.34962307344078880, 56.10051614449766078, -2.184720259617096705 ) ) ;
#7637=CARTESIAN_POINT ( 'NONE',  ( 46.45491332379572924, 63.29948385550240175, -4.840751629271157874 ) ) ;
#7646=CARTESIAN_POINT ( 'NONE',  ( 55.96859303347804371, 48.19948385550240033, 4.306917132069425946 ) ) ;
#7650=CARTESIAN_POINT ( 'NONE',  ( 53.54508667620424234, 56.70051614449766930, -4.840751629271188961 ) ) ;
#7654=CARTESIAN_POINT ( 'NONE',  ( 52.29715082351547295, 58.39948385550238896, 6.992620115222774047 ) ) ;
#7664=DIRECTION ( 'NONE',  ( -0.04542589977017699732, 0.9989677110047501252, 0.000000000000000000 ) ) ;
#7665=CARTESIAN_POINT ( 'NONE',  ( 52.25172492374522903, 49.59948385550240602, -7.007379884777227730 ) ) ;
#7666=CARTESIAN_POINT ( 'NONE',  ( 54.09612160359792199, 51.30051614449766362, 5.676469297603124353 ) ) ;
#7669=CARTESIAN_POINT ( 'NONE',  ( 54.09612160359786515, 49.69948385550240744, -5.676469297603166098 ) ) ;
#7671=CARTESIAN_POINT ( 'NONE',  ( 56.81924384183011512, 64.19948385550240744, 4.924951120819313743 ) ) ;
#7677=CARTESIAN_POINT ( 'NONE',  ( 44.30067958973594955, 54.10051614449766078, -1.875703265242155693 ) ) ;
#7678=CARTESIAN_POINT ( 'NONE',  ( 49.97728705011495265, 63.50051614449765935, 7.000000000000000888 ) ) ;
#7679=CARTESIAN_POINT ( 'NONE',  ( 58.41169779390614281, 49.99948385550240459, -0.02388180880523160798 ) ) ;
#7680=CARTESIAN_POINT ( 'NONE',  ( 49.97728705011488159, 59.49948385550240459, -7.000000000000000888 ) ) ;
#7682=CARTESIAN_POINT ( 'NONE',  ( 52.57664461997821093, 61.40051614449765793, 8.007379884777206414 ) ) ;
#7693=CARTESIAN_POINT ( 'NONE',  ( 49.97728705011488870, 57.49948385550241170, -6.000000000000000888 ) ) ;
#7694=CARTESIAN_POINT ( 'NONE',  ( 56.66441430157294690, 46.90051614449765793, -2.141517661632166281 ) ) ;
#7695=CARTESIAN_POINT ( 'NONE',  ( 41.58830220609386430, 50.00051614449765935, -0.02388180880514929535 ) ) ;
#7699=CARTESIAN_POINT ( 'NONE',  ( 49.97728705011495265, 55.50051614449766646, 7.000000000000000888 ) ) ;
#7713=CARTESIAN_POINT ( 'NONE',  ( 56.65037692655918988, 59.89948385550241028, -2.184720259617163762 ) ) ;
#7715=CARTESIAN_POINT ( 'NONE',  ( 55.71335778527780036, 60.90051614449766504, -1.832500667257213056 ) ) ;
#7721=CARTESIAN_POINT ( 'NONE',  ( 43.33558569842703179, 65.09948385550239891, -2.141517661632099223 ) ) ;
#7734=CARTESIAN_POINT ( 'NONE',  ( 52.25172492374522903, 51.59948385550240602, -7.007379884777227730 ) ) ;
#7735=CARTESIAN_POINT ( 'NONE',  ( 47.70284917648459100, 53.60051614449765367, 6.992620115222796251 ) ) ;
#7738=CARTESIAN_POINT ( 'NONE',  ( 52.29715082351547295, 50.39948385550240317, 6.992620115222774047 ) ) ;
#7739=CARTESIAN_POINT ( 'NONE',  ( 57.36023556966787851, 49.99948385550238328, -0.02388180880522424582 ) ) ;
#7740=CARTESIAN_POINT ( 'NONE',  ( 43.18075615816989199, 61.19948385550241454, -4.924951120819313743 ) ) ;
#7749=CARTESIAN_POINT ( 'NONE',  ( 46.45491332379576477, 53.70051614449766220, 4.840751629271188961 ) ) ;
#7752=CARTESIAN_POINT ( 'NONE',  ( 57.61547081786812896, 50.09948385550240602, 2.450534656007040901 ) ) ;
#7753=CARTESIAN_POINT ( 'NONE',  ( 55.96859303347804371, 58.19948385550241454, 4.306917132069425946 ) ) ;
#7755=CARTESIAN_POINT ( 'NONE',  ( 49.97728705011495265, 61.50051614449766646, 8.000000000000001776 ) ) ;
#7765=CARTESIAN_POINT ( 'NONE',  ( 44.30067958973596376, 54.89948385550240317, 1.875703265242204099 ) ) ;
#7766=CARTESIAN_POINT ( 'NONE',  ( 44.03140696652198471, 49.80051614449765651, 4.306917132069485454 ) ) ;
#7767=CARTESIAN_POINT ( 'NONE',  ( 52.57664461997821093, 53.40051614449765793, 8.007379884777206414 ) ) ;
#7772=CARTESIAN_POINT ( 'NONE',  ( 53.93078149122418807, 45.00000000000000000, -5.235029531081472953 ) ) ;
#7773=CARTESIAN_POINT ( 'NONE',  ( 44.05948171654945611, 64.20051614449765509, -4.345558710429044069 ) ) ;
#7783=CARTESIAN_POINT ( 'NONE',  ( 45.90387839640214196, 56.69948385550240744, 5.676469297603166098 ) ) ;
#7784=CARTESIAN_POINT ( 'NONE',  ( 56.30877334542961421, 59.00051614449766646, 0.02388180880515774693 ) ) ;
#7787=CARTESIAN_POINT ( 'NONE',  ( 56.65037692655921120, 45.10051614449766078, 2.184720259617097593 ) ) ;
#7788=CARTESIAN_POINT ( 'NONE',  ( 45.86712807150323812, 65.29948385550241596, -5.649768623646098220 ) ) ;
#7803=CARTESIAN_POINT ( 'NONE',  ( 57.36023556966787851, 53.00051614449765225, 0.02388180880515038476 ) ) ;
#7805=CARTESIAN_POINT ( 'NONE',  ( 56.66441430157296821, 54.09948385550240602, 2.141517661632100111 ) ) ;
#7808=CARTESIAN_POINT ( 'NONE',  ( 43.18075615816989199, 65.19948385550240744, -4.924951120819313743 ) ) ;
#7816=CARTESIAN_POINT ( 'NONE',  ( 55.08986747509849380, 57.20051614449766220, 3.727524721679155384 ) ) ;
#7818=CARTESIAN_POINT ( 'NONE',  ( 56.81924384183011512, 52.19948385550240744, 4.924951120819313743 ) ) ;
#7820=CARTESIAN_POINT ( 'NONE',  ( 54.13287192849676188, 54.29948385550240886, 5.649768623646098220 ) ) ;
#7823=CARTESIAN_POINT ( 'NONE',  ( 57.60143344285435774, 61.10051614449766788, 2.493737253992045044 ) ) ;
#7832=AXIS2_PLACEMENT_3D ( 'NONE', #4525, #12192, #3554 ) ;
#7835=CARTESIAN_POINT ( 'NONE',  ( 56.30877334542961421, 55.99948385550241170, -0.02388180880520959434 ) ) ;
#7836=CARTESIAN_POINT ( 'NONE',  ( 44.05948171654945611, 46.20051614449766220, -4.345558710429044069 ) ) ;
#7838=CARTESIAN_POINT ( 'NONE',  ( 49.97728705011495265, 51.50051614449765935, 8.000000000000001776 ) ) ;
#7842=CARTESIAN_POINT ( 'NONE',  ( 50.02271294988505446, 44.50051614449765935, -8.000000000000001776 ) ) ;
#7850=CARTESIAN_POINT ( 'NONE',  ( 57.36023556966787851, 57.99948385550239038, -0.02388180880522424582 ) ) ;
#7852=CARTESIAN_POINT ( 'NONE',  ( 55.71335778527780036, 56.90051614449767214, -1.832500667257213056 ) ) ;
#7855=CARTESIAN_POINT ( 'NONE',  ( 49.97728705011495265, 45.50051614449765935, 7.000000000000000888 ) ) ;
#7856=CARTESIAN_POINT ( 'NONE',  ( 48.07319477248768180, 48.59948385550239891, 6.007379884777225953 ) ) ;
#7869=CARTESIAN_POINT ( 'NONE',  ( 43.33558569842706021, 53.90051614449765793, 2.141517661632167169 ) ) ;
#7872=CARTESIAN_POINT ( 'NONE',  ( 43.33558569842703179, 55.09948385550241312, -2.141517661632099223 ) ) ;
#7873=CARTESIAN_POINT ( 'NONE',  ( 52.25172492374522903, 47.59948385550239891, -7.007379884777225953 ) ) ;
#7875=CARTESIAN_POINT ( 'NONE',  ( 49.97728705011486738, 61.49948385550241170, -8.000000000000001776 ) ) ;
#7886=CARTESIAN_POINT ( 'NONE',  ( 49.97728705011494554, 57.50051614449766646, 6.000000000000000888 ) ) ;
#7887=CARTESIAN_POINT ( 'NONE',  ( 47.70284917648459810, 63.60051614449766078, 6.992620115222797139 ) ) ;
#7888=CARTESIAN_POINT ( 'NONE',  ( 57.60143344285433642, 53.89948385550240317, -2.493737253992118319 ) ) ;
#7889=CARTESIAN_POINT ( 'NONE',  ( 54.09612160359786515, 57.69948385550240744, -5.676469297603166098 ) ) ;
#7891=CARTESIAN_POINT ( 'NONE',  ( 52.62207051974839089, 46.39948385550240317, 7.992620115222770494 ) ) ;
#7901=CARTESIAN_POINT ( 'NONE',  ( 55.08986747509847248, 57.79948385550240175, -3.727524721679197572 ) ) ;
#7902=CARTESIAN_POINT ( 'NONE',  ( 54.13287192849671214, 48.70051614449766220, -5.649768623646139964 ) ) ;
#7903=CARTESIAN_POINT ( 'NONE',  ( 47.42335538002180328, 52.40051614449767214, -8.007379884777206414 ) ) ;
#7906=CARTESIAN_POINT ( 'NONE',  ( 55.94051828345053679, 61.20051614449766220, 4.345558710429044069 ) ) ;
#7914=CARTESIAN_POINT ( 'NONE',  ( 56.65037692655918988, 55.89948385550240317, -2.184720259617163762 ) ) ;
#7916=CARTESIAN_POINT ( 'NONE',  ( 46.49166364869456913, 58.30051614449765651, -4.867452303228181343 ) ) ;
#7919=CARTESIAN_POINT ( 'NONE',  ( 44.88205777487401349, 61.80051614449766362, 3.688883143319584779 ) ) ;
#7920=CARTESIAN_POINT ( 'NONE',  ( 49.97728705011488159, 63.49948385550241170, -7.000000000000000888 ) ) ;
#7928=SURFACE_STYLE_USAGE ( .BOTH. , #8834 ) ;
#7931=CARTESIAN_POINT ( 'NONE',  ( 47.70284917648459100, 57.60051614449764656, 6.992620115222796251 ) ) ;
#7935=CARTESIAN_POINT ( 'NONE',  ( 47.70284917648453415, 55.39948385550238896, -6.992620115222774047 ) ) ;
#7936=CARTESIAN_POINT ( 'NONE',  ( 44.05948171654949874, 46.79948385550238754, 4.345558710429105354 ) ) ;
#7938=CARTESIAN_POINT ( 'NONE',  ( 43.18075615816989199, 63.19948385550240744, -4.924951120819313743 ) ) ;
#7948=CARTESIAN_POINT ( 'NONE',  ( 53.54508667620424234, 62.70051614449766220, -4.840751629271188961 ) ) ;
#7950=CARTESIAN_POINT ( 'NONE',  ( 43.18075615816989199, 65.19948385550240744, -4.924951120819313743 ) ) ;
#7951=CARTESIAN_POINT ( 'NONE',  ( 43.18075615816989199, 51.19948385550240744, -4.924951120819313743 ) ) ;
#7953=CARTESIAN_POINT ( 'NONE',  ( 50.02271294988512551, 64.49948385550240459, 7.000000000000000888 ) ) ;
#7955=CARTESIAN_POINT ( 'NONE',  ( 42.38452918213190657, 61.90051614449766504, 2.450534656007115508 ) ) ;
#7966=CARTESIAN_POINT ( 'NONE',  ( 44.28664221472220675, 63.09948385550240602, -1.832500667257165317 ) ) ;
#7967=CARTESIAN_POINT ( 'NONE',  ( 57.36023556966787851, 55.00051614449765935, 0.02388180880515038476 ) ) ;
#7968=CARTESIAN_POINT ( 'NONE',  ( 57.61547081786810764, 54.90051614449765793, -2.450534656007114176 ) ) ;
#7971=CARTESIAN_POINT ( 'NONE',  ( 57.60143344285435774, 45.10051614449766788, 2.493737253992045044 ) ) ;
#7982=CARTESIAN_POINT ( 'NONE',  ( 52.29715082351547295, 58.39948385550238896, 6.992620115222774047 ) ) ;
#7983=CARTESIAN_POINT ( 'NONE',  ( 47.74827507625477807, 52.59948385550239891, 7.007379884777229506 ) ) ;
#7987=CARTESIAN_POINT ( 'NONE',  ( 55.96859303347802239, 44.80051614449767072, -4.306917132069484566 ) ) ;
#7988=CARTESIAN_POINT ( 'NONE',  ( 44.28664221472220675, 49.09948385550241312, -1.832500667257165317 ) ) ;
#7999=FILL_AREA_STYLE_COLOUR ( '', #6612 ) ;
#8002=CARTESIAN_POINT ( 'NONE',  ( 56.65037692655921120, 57.10051614449766078, 2.184720259617097593 ) ) ;
#8004=CARTESIAN_POINT ( 'NONE',  ( 46.45491332379572924, 65.29948385550241596, -4.840751629271157874 ) ) ;
#8006=CARTESIAN_POINT ( 'NONE',  ( 42.63976443033212860, 58.99948385550239038, 0.02388180880522514787 ) ) ;
#8007=CARTESIAN_POINT ( 'NONE',  ( 52.25172492374522903, 49.59948385550240602, -7.007379884777225953 ) ) ;
#8009=CARTESIAN_POINT ( 'NONE',  ( 45.90387839640214196, 48.69948385550240744, 5.676469297603166098 ) ) ;
#8017=CARTESIAN_POINT ( 'NONE',  ( 49.97728705011494554, 61.50051614449766646, 6.000000000000000888 ) ) ;
#8020=CARTESIAN_POINT ( 'NONE',  ( 54.72065718078924590, 58.29948385550240886, 6.458785618021043895 ) ) ;
#8021=CARTESIAN_POINT ( 'NONE',  ( 45.86712807150323812, 61.29948385550240886, -5.649768623646098220 ) ) ;
#8023=CARTESIAN_POINT ( 'NONE',  ( 45.27934281921075410, 53.29948385550240886, -6.458785618021043895 ) ) ;
#8034=CARTESIAN_POINT ( 'NONE',  ( 50.02271294988511841, 60.49948385550240459, 6.000000000000000888 ) ) ;
#8035=CARTESIAN_POINT ( 'NONE',  ( 54.13287192849671214, 54.70051614449766220, -5.649768623646139964 ) ) ;
#8037=CARTESIAN_POINT ( 'NONE',  ( 45.31609314410960820, 62.30051614449766362, -6.485486291978072693 ) ) ;
#8038=DIRECTION ( 'NONE',  ( -0.9989677110047504582, -0.04542589977017007230, 1.386346192018204258E-14 ) ) ;
#8039=CARTESIAN_POINT ( 'NONE',  ( 49.99999999999997158, 45.00000000000001421, -6.500000000000004441 ) ) ;
#8040=CARTESIAN_POINT ( 'NONE',  ( 49.97728705011495265, 61.50051614449765935, 7.000000000000000888 ) ) ;
#8044=EDGE_CURVE ( 'NONE', #5739, #3958, #5567, .T. ) ;
#8051=APPLICATION_CONTEXT ( 'automotive_design' ) ;
#8054=CARTESIAN_POINT ( 'NONE',  ( 52.29715082351547295, 64.39948385550239607, 6.992620115222774047 ) ) ;
#8055=CARTESIAN_POINT ( 'NONE',  ( 45.90387839640214196, 56.69948385550240744, 5.676469297603166098 ) ) ;
#8061=CARTESIAN_POINT ( 'NONE',  ( 52.29715082351538769, 44.60051614449766788, -6.992620115222796251 ) ) ;
#8062=CARTESIAN_POINT ( 'NONE',  ( 48.07319477248768180, 52.59948385550240602, 6.007379884777225953 ) ) ;
#8076=CARTESIAN_POINT ( 'NONE',  ( 44.88205777487401349, 47.80051614449764941, 3.688883143319584779 ) ) ;
#8078=CARTESIAN_POINT ( 'NONE',  ( 44.05948171654949874, 60.79948385550240886, 4.345558710429105354 ) ) ;
#8079=CARTESIAN_POINT ( 'NONE',  ( 57.36023556966787851, 51.99948385550238328, -0.02388180880522424582 ) ) ;
#8081=CARTESIAN_POINT ( 'NONE',  ( 55.96859303347804371, 46.19948385550238612, 4.306917132069425946 ) ) ;
#8090=CARTESIAN_POINT ( 'NONE',  ( 51.97223112728249816, 58.60051614449766788, -5.992620115222793586 ) ) ;
#8093=CARTESIAN_POINT ( 'NONE',  ( 42.39856655714566358, 58.89948385550241028, 2.493737253992119207 ) ) ;
#8096=CARTESIAN_POINT ( 'NONE',  ( 54.72065718078924590, 50.29948385550240886, 6.458785618021043895 ) ) ;
#8107=CARTESIAN_POINT ( 'NONE',  ( 46.45491332379572924, 65.29948385550241596, -4.840751629271157874 ) ) ;
#8108=CARTESIAN_POINT ( 'NONE',  ( 54.09612160359792199, 51.30051614449766362, 5.676469297603124353 ) ) ;
#8109=CARTESIAN_POINT ( 'NONE',  ( 57.61547081786810764, 56.90051614449767214, -2.450534656007114176 ) ) ;
#8112=CARTESIAN_POINT ( 'NONE',  ( 57.61547081786810764, 52.90051614449766504, -2.450534656007114176 ) ) ;
#8121=SHAPE_DEFINITION_REPRESENTATION ( #3124, #4503 ) ;
#8122=CARTESIAN_POINT ( 'NONE',  ( 55.11794222512601493, 46.19948385550240744, 3.688883143319541702 ) ) ;
#8123=CARTESIAN_POINT ( 'NONE',  ( 55.96859303347805081, 56.19948385550240744, 4.306917132069425058 ) ) ;
#8127=CARTESIAN_POINT ( 'NONE',  ( 55.96859303347802239, 48.80051614449766362, -4.306917132069484566 ) ) ;
#8128=CARTESIAN_POINT ( 'NONE',  ( 49.97728705011488870, 51.49948385550240459, -6.000000000000000888 ) ) ;
#8139=CARTESIAN_POINT ( 'NONE',  ( 43.34962307344081012, 46.89948385550240317, 2.184720259617164650 ) ) ;
#8142=CARTESIAN_POINT ( 'NONE',  ( 48.02776887271745210, 65.39948385550239607, -5.992620115222778487 ) ) ;
#8144=CARTESIAN_POINT ( 'NONE',  ( 55.96859303347804371, 60.19948385550240744, 4.306917132069425946 ) ) ;
#8145=CARTESIAN_POINT ( 'NONE',  ( 44.03140696652192787, 51.19948385550238612, -4.306917132069425058 ) ) ;
#8149=CARTESIAN_POINT ( 'NONE',  ( 43.34962307344081012, 48.89948385550240317, 2.184720259617164650 ) ) ;
#8160=CARTESIAN_POINT ( 'NONE',  ( 55.69932041026405045, 61.10051614449766788, 1.875703265242156359 ) ) ;
#8162=CARTESIAN_POINT ( 'NONE',  ( 43.20883090819745576, 56.79948385550240175, 4.963592699179006473 ) ) ;
#8163=CARTESIAN_POINT ( 'NONE',  ( 44.05948171654949874, 62.79948385550241596, 4.345558710429105354 ) ) ;
#8166=CARTESIAN_POINT ( 'NONE',  ( 47.42335538002188144, 52.59948385550240602, 8.007379884777233059 ) ) ;
#8177=CARTESIAN_POINT ( 'NONE',  ( 44.88205777487398507, 63.19948385550240744, -3.688883143319540814 ) ) ;
#8178=CARTESIAN_POINT ( 'NONE',  ( 49.97728705011495265, 53.50051614449765935, 7.000000000000000888 ) ) ;
#8179=CARTESIAN_POINT ( 'NONE',  ( 56.81924384183006538, 56.80051614449764941, -4.924951120819380357 ) ) ;
#8181=CARTESIAN_POINT ( 'NONE',  ( 45.27934281921082516, 47.70051614449766220, 6.458785618021089192 ) ) ;
#8186=PRODUCT_DEFINITION_CONTEXT ( 'detailed design', #8051, 'design' ) ;
#8192=CARTESIAN_POINT ( 'NONE',  ( 45.90387839640214196, 62.69948385550240744, 5.676469297603166098 ) ) ;
#8194=CARTESIAN_POINT ( 'NONE',  ( 55.94051828345050836, 57.79948385550240175, -4.345558710429103577 ) ) ;
#8199=CARTESIAN_POINT ( 'NONE',  ( 55.94051828345053679, 49.20051614449766930, 4.345558710429044069 ) ) ;
#8200=CARTESIAN_POINT ( 'NONE',  ( 56.30877334542961421, 51.99948385550239749, -0.02388180880520959434 ) ) ;
#8210=CARTESIAN_POINT ( 'NONE',  ( 54.09612160359786515, 47.69948385550240744, -5.676469297603166098 ) ) ;
#8213=CARTESIAN_POINT ( 'NONE',  ( 53.50833635130544508, 47.30051614449766362, 4.867452303228181343 ) ) ;
#8215=CARTESIAN_POINT ( 'NONE',  ( 47.70284917648453415, 59.39948385550241028, -6.992620115222774047 ) ) ;
#8216=CARTESIAN_POINT ( 'NONE',  ( 42.63976443033212860, 50.99948385550240459, 0.02388180880522514787 ) ) ;
#8220=CARTESIAN_POINT ( 'NONE',  ( 45.86712807150323812, 47.29948385550240886, -5.649768623646098220 ) ) ;
#8231=CARTESIAN_POINT ( 'NONE',  ( 48.02776887271750184, 63.60051614449764656, 5.992620115222795363 ) ) ;
#8234=( BOUNDED_CURVE ( )  B_SPLINE_CURVE ( 2, ( #4511, #413, #3407, #5555, #12112, #3475, #9894, #1379, #2633, #10933, #9767, #10864, #3679, #1310, #12864, #7836, #12048, #4581, #2566, #4721, #1448, #12999, #7694, #8738, #4651, #5694, #10994, #4442, #8869, #8939, #5764, #288, #1518, #480, #11063, #10791, #12928, #8797, #5625, #13138, #7902, #6859, #1585, #9835, #10030, #7629, #11833, #2356, #6593, #11903, #3542, #7766, #11979, #2425, #354, #2498, #12179, #2916, #5068, #11136, #11205, #5973, #2779, #9282, #6046, #6183, #8108, #13472, #3746, #2989, #12312, #7142, #8248, #6115, #10238, #6929, #2704, #751, #11349, #1726, #4022, #3816, #606, #1656, #545, #5900, #10175, #1936, #8178, #3882, #677, #5000, #10097, #11279, #4930, #2845, #9000, #4789, #7068, #10309, #8035, #13197, #1871, #7967, #4859, #9074, #9142, #12247, #9213, #13268, #7000, #12448, #3949, #13335, #1799, #816, #13403, #12382, #7211, #11416, #3189, #2010, #3119, #9616, #7280, #891, #5342, #73, #10515, #9548, #10651, #12652, #11492, #9351, #2140, #7479, #1027, #9477, #2074, #12518, #6323, #11684, #6258, #7419, #10582, #3324, #3050, #10449, #5276, #7352, #11625, #4293, #2, #13546, #4225, #8381, #6385, #139, #4097, #6448, #8517, #8446, #1090, #12717, #2205, #4359, #12588, #3258, #12780, #9418, #1165, #5411, #8578, #7542, #11752, #957, #2270, #10379, #5143, #8318, #5216, #11564, #13615, #4157, #6577, #12846, #12092, #11816, #7678, #7887, #399, #9817, #11886, #2479, #2339, #3525, #2407, #337, #1229 ),
 .UNSPECIFIED., .F., .F. ) 
 B_SPLINE_CURVE_WITH_KNOTS ( ( 3, 2, 2, 2, 2, 2, 2, 2, 2, 2, 2, 2, 2, 2, 2, 2, 2, 2, 2, 2, 2, 2, 2, 2, 2, 2, 2, 2, 2, 2, 2, 2, 2, 2, 2, 2, 2, 2, 2, 2, 2, 2, 2, 2, 2, 2, 2, 2, 2, 2, 2, 2, 2, 2, 2, 2, 2, 2, 2, 2, 2, 2, 2, 2, 2, 2, 2, 2, 2, 2, 2, 2, 2, 2, 2, 2, 2, 2, 2, 2, 2, 2, 2, 2, 2, 2, 2, 2, 2, 2, 2, 2, 2, 2, 2, 2, 2, 2, 2, 3 ),
 ( 0.01230184727895902198, 0.02000000000000000042, 0.02999999999999999889, 0.04000000000000000083, 0.05000000000000000278, 0.05999999999999999778, 0.07000000000000000666, 0.08000000000000000167, 0.08999999999999999667, 0.1000000000000000056, 0.1100000000000000006, 0.1199999999999999956, 0.1300000000000000044, 0.1400000000000000133, 0.1499999999999999944, 0.1600000000000000033, 0.1700000000000000122, 0.1799999999999999933, 0.1900000000000000022, 0.2000000000000000111, 0.2099999999999999922, 0.2200000000000000011, 0.2300000000000000100, 0.2399999999999999911, 0.2500000000000000000, 0.2600000000000000089, 0.2700000000000000178, 0.2800000000000000266, 0.2899999999999999800, 0.2999999999999999889, 0.3099999999999999978, 0.3200000000000000067, 0.3300000000000000155, 0.3400000000000000244, 0.3499999999999999778, 0.3599999999999999867, 0.3699999999999999956, 0.3800000000000000044, 0.3900000000000000133, 0.4000000000000000222, 0.4099999999999999756, 0.4199999999999999845, 0.4299999999999999933, 0.4400000000000000022, 0.4500000000000000111, 0.4600000000000000200, 0.4699999999999999734, 0.4799999999999999822, 0.4899999999999999911, 0.5000000000000000000, 0.5100000000000000089, 0.5200000000000000178, 0.5300000000000000266, 0.5400000000000000355, 0.5500000000000000444, 0.5600000000000000533, 0.5699999999999999512, 0.5799999999999999600, 0.5899999999999999689, 0.5999999999999999778, 0.6099999999999999867, 0.6199999999999999956, 0.6300000000000000044, 0.6400000000000000133, 0.6500000000000000222, 0.6600000000000000311, 0.6700000000000000400, 0.6800000000000000488, 0.6899999999999999467, 0.6999999999999999556, 0.7099999999999999645, 0.7199999999999999734, 0.7299999999999999822, 0.7399999999999999911, 0.7500000000000000000, 0.7600000000000000089, 0.7700000000000000178, 0.7800000000000000266, 0.7900000000000000355, 0.8000000000000000444, 0.8100000000000000533, 0.8199999999999999512, 0.8299999999999999600, 0.8399999999999999689, 0.8499999999999999778, 0.8599999999999999867, 0.8699999999999999956, 0.8800000000000000044, 0.8900000000000000133, 0.9000000000000000222, 0.9100000000000000311, 0.9200000000000000400, 0.9300000000000000488, 0.9399999999999999467, 0.9499999999999999556, 0.9599999999999999645, 0.9699999999999999734, 0.9799999999999999822, 0.9899999999999999911, 1.000000000000000000 ),
 .UNSPECIFIED. ) 
 CURVE ( )  GEOMETRIC_REPRESENTATION_ITEM ( )  RATIONAL_B_SPLINE_CURVE ( ( 0.9826544568871729002, 0.9623225587740311671, 1.000000000000000000, 0.9510565162951535312, 1.000000000000000000, 0.9510565162951535312, 1.000000000000000000, 0.9510565162951535312, 1.000000000000000000, 0.9510565162951535312, 1.000000000000000000, 0.9510565162951535312, 1.000000000000000000, 0.9510565162951535312, 1.000000000000000000, 0.9510565162951535312, 1.000000000000000000, 0.9510565162951535312, 1.000000000000000000, 0.9510565162951535312, 1.000000000000000000, 0.9510565162951535312, 1.000000000000000000, 0.9510565162951535312, 1.000000000000000000, 0.9510565162951535312, 1.000000000000000000, 0.9510565162951535312, 1.000000000000000000, 0.9510565162951535312, 1.000000000000000000, 0.9510565162951535312, 1.000000000000000000, 0.9510565162951535312, 1.000000000000000000, 0.9510565162951535312, 1.000000000000000000, 0.9510565162951535312, 1.000000000000000000, 0.9510565162951535312, 1.000000000000000000, 0.9510565162951535312, 1.000000000000000000, 0.9510565162951535312, 1.000000000000000000, 0.9510565162951535312, 1.000000000000000000, 0.9510565162951535312, 1.000000000000000000, 0.9510565162951535312, 1.000000000000000000, 0.9510565162951535312, 1.000000000000000000, 0.9510565162951535312, 1.000000000000000000, 0.9510565162951535312, 1.000000000000000000, 0.9510565162951535312, 1.000000000000000000, 0.9510565162951535312, 1.000000000000000000, 0.9510565162951535312, 1.000000000000000000, 0.9510565162951535312, 1.000000000000000000, 0.9510565162951535312, 1.000000000000000000, 0.9510565162951535312, 1.000000000000000000, 0.9510565162951535312, 1.000000000000000000, 0.9510565162951535312, 1.000000000000000000, 0.9510565162951535312, 1.000000000000000000, 0.9510565162951535312, 1.000000000000000000, 0.9510565162951535312, 1.000000000000000000, 0.9510565162951535312, 1.000000000000000000, 0.9510565162951535312, 1.000000000000000000, 0.9510565162951535312, 1.000000000000000000, 0.9510565162951535312, 1.000000000000000000, 0.9510565162951535312, 1.000000000000000000, 0.9510565162951535312, 1.000000000000000000, 0.9510565162951535312, 1.000000000000000000, 0.9510565162951535312, 1.000000000000000000, 0.9510565162951535312, 1.000000000000000000, 0.9510565162951535312, 1.000000000000000000, 0.9510565162951535312, 1.000000000000000000, 0.9510565162951535312, 1.000000000000000000, 0.9510565162951535312, 1.000000000000000000, 0.9510565162951535312, 1.000000000000000000, 0.9510565162951535312, 1.000000000000000000, 0.9510565162951535312, 1.000000000000000000, 0.9510565162951535312, 1.000000000000000000, 0.9510565162951535312, 1.000000000000000000, 0.9510565162951535312, 1.000000000000000000, 0.9510565162951535312, 1.000000000000000000, 0.9510565162951535312, 1.000000000000000000, 0.9510565162951535312, 1.000000000000000000, 0.9510565162951535312, 1.000000000000000000, 0.9510565162951535312, 1.000000000000000000, 0.9510565162951535312, 1.000000000000000000, 0.9510565162951535312, 1.000000000000000000, 0.9510565162951535312, 1.000000000000000000, 0.9510565162951535312, 1.000000000000000000, 0.9510565162951535312, 1.000000000000000000, 0.9510565162951535312, 1.000000000000000000, 0.9510565162951535312, 1.000000000000000000, 0.9510565162951535312, 1.000000000000000000, 0.9510565162951535312, 1.000000000000000000, 0.9510565162951535312, 1.000000000000000000, 0.9510565162951535312, 1.000000000000000000, 0.9510565162951535312, 1.000000000000000000, 0.9510565162951535312, 1.000000000000000000, 0.9510565162951535312, 1.000000000000000000, 0.9510565162951535312, 1.000000000000000000, 0.9510565162951535312, 1.000000000000000000, 0.9510565162951535312, 1.000000000000000000, 0.9510565162951535312, 1.000000000000000000, 0.9510565162951535312, 1.000000000000000000, 0.9510565162951535312, 1.000000000000000000, 0.9510565162951535312, 1.000000000000000000, 0.9510565162951535312, 1.000000000000000000, 0.9510565162951535312, 1.000000000000000000, 0.9510565162951535312, 1.000000000000000000, 0.9510565162951535312, 1.000000000000000000, 0.9510565162951535312, 1.000000000000000000, 0.9510565162951535312, 1.000000000000000000, 0.9510565162951535312, 1.000000000000000000, 0.9510565162951535312, 1.000000000000000000, 0.9510565162951535312, 1.000000000000000000, 0.9510565162951535312, 1.000000000000000000, 0.9510565162951535312, 1.000000000000000000, 0.9510565162951535312, 1.000000000000000000, 0.9510565162951535312, 1.000000000000000000, 0.9510565162951535312, 1.000000000000000000, 0.9510565162951535312, 1.000000000000000000 ) ) 
 REPRESENTATION_ITEM ( '' )  );
#8235=CARTESIAN_POINT ( 'NONE',  ( 45.31609314410967926, 60.69948385550240033, 6.485486291978119766 ) ) ;
#8237=CARTESIAN_POINT ( 'NONE',  ( 56.81924384183011512, 50.19948385550241454, 4.924951120819313743 ) ) ;
#8247=CARTESIAN_POINT ( 'NONE',  ( 46.45491332379572924, 61.29948385550240886, -4.840751629271157874 ) ) ;
#8248=CARTESIAN_POINT ( 'NONE',  ( 43.33558569842706021, 51.90051614449765793, 2.141517661632167169 ) ) ;
#8249=CARTESIAN_POINT ( 'NONE',  ( 47.37792948025170858, 59.60051614449765367, 7.992620115222797139 ) ) ;
#8252=CARTESIAN_POINT ( 'NONE',  ( 41.58830220609386430, 48.00051614449766646, -0.02388180880514929535 ) ) ;
#8262=CARTESIAN_POINT ( 'NONE',  ( 56.65037692655918988, 61.89948385550241028, -2.184720259617163762 ) ) ;
#8263=CARTESIAN_POINT ( 'NONE',  ( 49.97728705011488159, 57.49948385550241170, -7.000000000000000888 ) ) ;
#8265=CARTESIAN_POINT ( 'NONE',  ( 42.63976443033212860, 62.00051614449764514, -0.02388180880514948964 ) ) ;
#8269=CARTESIAN_POINT ( 'NONE',  ( 49.97728705011495265, 49.50051614449765935, 7.000000000000000888 ) ) ;
#8270=CARTESIAN_POINT ( 'NONE',  ( 48.02776887271745210, 49.39948385550241028, -5.992620115222778487 ) ) ;
#8285=CARTESIAN_POINT ( 'NONE',  ( 55.08986747509849380, 45.20051614449766220, 3.727524721679155384 ) ) ;
#8288=CARTESIAN_POINT ( 'NONE',  ( 52.29715082351547295, 64.39948385550239607, 6.992620115222774047 ) ) ;
#8289=CARTESIAN_POINT ( 'NONE',  ( 50.02271294988512551, 56.49948385550240459, 7.000000000000000888 ) ) ;
#8291=CARTESIAN_POINT ( 'NONE',  ( 50.02271294988512551, 50.49948385550240459, 7.000000000000000888 ) ) ;
#8299=CARTESIAN_POINT ( 'NONE',  ( 45.86712807150323812, 47.29948385550240886, -5.649768623646098220 ) ) ;
#8300=CARTESIAN_POINT ( 'NONE',  ( 47.70284917648459100, 47.60051614449763946, 6.992620115222796251 ) ) ;
#8302=CARTESIAN_POINT ( 'NONE',  ( 42.38452918213188525, 61.09948385550241312, -2.450534656007040013 ) ) ;
#8305=EDGE_CURVE ( 'NONE', #725, #9956, #13241, .T. ) ;
#8306=CARTESIAN_POINT ( 'NONE',  ( 43.20883090819745576, 52.79948385550240175, 4.963592699179006473 ) ) ;
#8317=CARTESIAN_POINT ( 'NONE',  ( 43.69122665457040000, 48.00051614449766646, -0.02388180880515696977 ) ) ;
#8318=CARTESIAN_POINT ( 'NONE',  ( 52.29715082351539479, 62.60051614449766078, -6.992620115222796251 ) ) ;
#8319=CARTESIAN_POINT ( 'NONE',  ( 47.42335538002180328, 56.40051614449765793, -8.007379884777206414 ) ) ;
#8321=CARTESIAN_POINT ( 'NONE',  ( 56.79116909180259398, 47.20051614449766220, 4.963592699178938972 ) ) ;
#8334=CARTESIAN_POINT ( 'NONE',  ( 44.05948171654949874, 60.79948385550240886, 4.345558710429105354 ) ) ;
#8335=CARTESIAN_POINT ( 'NONE',  ( 52.29715082351547295, 64.39948385550239607, 6.992620115222774047 ) ) ;
#8336=CARTESIAN_POINT ( 'NONE',  ( 47.74827507625469281, 58.40051614449766504, -7.007379884777203749 ) ) ;
#8340=CARTESIAN_POINT ( 'NONE',  ( 45.90387839640208512, 48.30051614449765651, -5.676469297603124353 ) ) ;
#8341=CARTESIAN_POINT ( 'NONE',  ( 44.88205777487398507, 59.19948385550240744, -3.688883143319540814 ) ) ;
#8353=CARTESIAN_POINT ( 'NONE',  ( 53.54508667620424234, 48.70051614449766930, -4.840751629271188961 ) ) ;
#8355=CARTESIAN_POINT ( 'NONE',  ( 47.70284917648453415, 63.39948385550240317, -6.992620115222774047 ) ) ;
#8356=CARTESIAN_POINT ( 'NONE',  ( 56.65037692655918988, 55.89948385550240317, -2.184720259617163762 ) ) ;
#8364=CARTESIAN_POINT ( 'NONE',  ( 44.03140696652198471, 45.80051614449764230, 4.306917132069485454 ) ) ;
#8368=CARTESIAN_POINT ( 'NONE',  ( 57.36023556966787851, 45.99948385550238328, -0.02388180880522424582 ) ) ;
#8371=CARTESIAN_POINT ( 'NONE',  ( 45.27934281921075410, 55.29948385550240175, -6.458785618021043895 ) ) ;
#8380=CARTESIAN_POINT ( 'NONE',  ( 43.69122665457040000, 50.00051614449765935, -0.02388180880515696977 ) ) ;
#8381=CARTESIAN_POINT ( 'NONE',  ( 44.05948171654945611, 60.20051614449765509, -4.345558710429044069 ) ) ;
#8382=CARTESIAN_POINT ( 'NONE',  ( 57.60143344285435774, 63.10051614449766078, 2.493737253992045044 ) ) ;
#8385=CARTESIAN_POINT ( 'NONE',  ( 54.72065718078918906, 58.70051614449765509, -6.458785618021089192 ) ) ;
#8396=CARTESIAN_POINT ( 'NONE',  ( 44.91013252490152752, 48.79948385550240175, 3.727524721679198461 ) ) ;
#8398=CARTESIAN_POINT ( 'NONE',  ( 42.63976443033212149, 64.99948385550240459, 0.02388180880522514787 ) ) ;
#8400=CARTESIAN_POINT ( 'NONE',  ( 49.97728705011495265, 63.50051614449765935, 7.000000000000000888 ) ) ;
#8405=CARTESIAN_POINT ( 'NONE',  ( 56.66441430157294690, 52.90051614449765793, -2.141517661632166281 ) ) ;
#8406=CARTESIAN_POINT ( 'NONE',  ( 55.11794222512601493, 56.19948385550240744, 3.688883143319541702 ) ) ;
#8417=CARTESIAN_POINT ( 'NONE',  ( 47.70284917648453415, 53.39948385550238186, -6.992620115222774047 ) ) ;
#8421=CARTESIAN_POINT ( 'NONE',  ( 44.91013252490150620, 54.20051614449766220, -3.727524721679154940 ) ) ;
#8423=CARTESIAN_POINT ( 'NONE',  ( 43.34962307344081012, 62.89948385550241028, 2.184720259617164650 ) ) ;
#8424=CARTESIAN_POINT ( 'NONE',  ( 43.33558569842703179, 63.09948385550240602, -2.141517661632099223 ) ) ;
#8425=CARTESIAN_POINT ( 'NONE',  ( 44.03140696652192787, 59.19948385550238612, -4.306917132069425058 ) ) ;
#8433=CARTESIAN_POINT ( 'NONE',  ( 44.05948171654945611, 50.20051614449764088, -4.345558710429044069 ) ) ;
#8436=CARTESIAN_POINT ( 'NONE',  ( 52.25172492374522903, 47.59948385550239891, -7.007379884777225953 ) ) ;
#8437=CARTESIAN_POINT ( 'NONE',  ( 56.79116909180255135, 55.79948385550239465, -4.963592699179005585 ) ) ;
#8445=CARTESIAN_POINT ( 'NONE',  ( 55.69932041026405045, 49.10051614449766788, 1.875703265242156359 ) ) ;
#8446=CARTESIAN_POINT ( 'NONE',  ( 55.96859303347802239, 60.80051614449765651, -4.306917132069484566 ) ) ;
#8447=CARTESIAN_POINT ( 'NONE',  ( 41.58830220609386430, 48.99948385550241170, 0.02388180880523263147 ) ) ;
#8450=CARTESIAN_POINT ( 'NONE',  ( 41.58830220609386430, 58.00051614449765935, -0.02388180880514929535 ) ) ;
#8461=CARTESIAN_POINT ( 'NONE',  ( 44.28664221472220675, 49.09948385550241312, -1.832500667257165317 ) ) ;
#8462=CARTESIAN_POINT ( 'NONE',  ( 56.66441430157296821, 64.09948385550239891, 2.141517661632100111 ) ) ;
#8463=CARTESIAN_POINT ( 'NONE',  ( 44.03140696652198471, 63.80051614449765651, 4.306917132069485454 ) ) ;
#8468=CARTESIAN_POINT ( 'NONE',  ( 56.65037692655921120, 59.10051614449766078, 2.184720259617097593 ) ) ;
#8469=CARTESIAN_POINT ( 'NONE',  ( 55.71335778527780747, 60.09948385550240602, 1.832500667257165983 ) ) ;
#8482=CARTESIAN_POINT ( 'NONE',  ( 56.65037692655918988, 51.89948385550241028, -2.184720259617163762 ) ) ;
#8484=CARTESIAN_POINT ( 'NONE',  ( 55.71335778527780036, 54.90051614449765793, -1.832500667257213056 ) ) ;
#8487=CARTESIAN_POINT ( 'NONE',  ( 55.96859303347804371, 62.19948385550240744, 4.306917132069425946 ) ) ;
#8489=CARTESIAN_POINT ( 'NONE',  ( 45.90387839640214196, 60.69948385550240033, 5.676469297603166098 ) ) ;
#8499=CARTESIAN_POINT ( 'NONE',  ( 45.90387839640214196, 46.69948385550240744, 5.676469297603166098 ) ) ;
#8501=CARTESIAN_POINT ( 'NONE',  ( 57.36023556966787851, 45.00051614449763804, 0.02388180880515038476 ) ) ;
#8504=CARTESIAN_POINT ( 'NONE',  ( 56.81924384183011512, 64.19948385550240744, 4.924951120819313743 ) ) ;
#8507=CARTESIAN_POINT ( 'NONE',  ( 56.81924384183011512, 56.19948385550240744, 4.924951120819313743 ) ) ;
#8516=CARTESIAN_POINT ( 'NONE',  ( 55.08986747509849380, 51.20051614449766220, 3.727524721679155384 ) ) ;
#8517=CARTESIAN_POINT ( 'NONE',  ( 54.13287192849671214, 60.70051614449766220, -5.649768623646139964 ) ) ;
#8518=CARTESIAN_POINT ( 'NONE',  ( 57.61547081786812896, 46.09948385550240602, 2.450534656007040901 ) ) ;
#8520=CARTESIAN_POINT ( 'NONE',  ( 45.27934281921082516, 55.70051614449766220, 6.458785618021089192 ) ) ;
#8529=CARTESIAN_POINT ( 'NONE',  ( 44.88205777487398507, 49.19948385550240744, -3.688883143319540814 ) ) ;
#8530=CARTESIAN_POINT ( 'NONE',  ( 52.29715082351547295, 62.39948385550240317, 6.992620115222774047 ) ) ;
#8532=CARTESIAN_POINT ( 'NONE',  ( 54.72065718078918906, 44.70051614449765509, -6.458785618021089192 ) ) ;
#8536=CARTESIAN_POINT ( 'NONE',  ( 54.13287192849671214, 58.70051614449765509, -5.649768623646139964 ) ) ;
#8537=CARTESIAN_POINT ( 'NONE',  ( 44.28664221472220675, 59.09948385550240602, -1.832500667257165317 ) ) ;
#8548=CARTESIAN_POINT ( 'NONE',  ( 57.36023556966787851, 53.99948385550239038, -0.02388180880522424582 ) ) ;
#8550=CARTESIAN_POINT ( 'NONE',  ( 53.54508667620424234, 54.70051614449765509, -4.840751629271188961 ) ) ;
#8554=CARTESIAN_POINT ( 'NONE',  ( 45.86712807150323812, 61.29948385550240886, -5.649768623646098220 ) ) ;
#8562=CARTESIAN_POINT ( 'NONE',  ( 55.94051828345050836, 51.79948385550240175, -4.345558710429103577 ) ) ;
#8563=CARTESIAN_POINT ( 'NONE',  ( 55.96859303347802239, 44.80051614449767072, -4.306917132069484566 ) ) ;
#8565=CARTESIAN_POINT ( 'NONE',  ( 55.94051828345050836, 45.79948385550240886, -4.345558710429104465 ) ) ;
#8569=CARTESIAN_POINT ( 'NONE',  ( 49.97728705011486738, 53.49948385550240459, -8.000000000000001776 ) ) ;
#8577=CARTESIAN_POINT ( 'NONE',  ( 44.91013252490150620, 50.20051614449766220, -3.727524721679154940 ) ) ;
#8578=CARTESIAN_POINT ( 'NONE',  ( 43.33558569842706021, 61.90051614449766504, 2.141517661632167169 ) ) ;
#8579=CARTESIAN_POINT ( 'NONE',  ( 43.18075615816989199, 47.19948385550240744, -4.924951120819313743 ) ) ;
#8581=CARTESIAN_POINT ( 'NONE',  ( 57.61547081786810764, 54.90051614449765793, -2.450534656007114176 ) ) ;
#8593=CARTESIAN_POINT ( 'NONE',  ( 55.08986747509847248, 49.79948385550240175, -3.727524721679197572 ) ) ;
#8595=CARTESIAN_POINT ( 'NONE',  ( 45.31609314410960820, 46.30051614449766362, -6.485486291978072693 ) ) ;
#8601=CARTESIAN_POINT ( 'NONE',  ( 57.36023556966787851, 55.00051614449765225, 0.02388180880515038476 ) ) ;
#8602=CARTESIAN_POINT ( 'NONE',  ( 43.69122665457040000, 56.99948385550241170, 0.02388180880521036456 ) ) ;
#8613=CARTESIAN_POINT ( 'NONE',  ( 43.33558569842703179, 53.09948385550240602, -2.141517661632099223 ) ) ;
#8617=CARTESIAN_POINT ( 'NONE',  ( 51.97223112728249816, 50.60051614449765367, -5.992620115222793586 ) ) ;
#8621=CARTESIAN_POINT ( 'NONE',  ( 49.97728705011488159, 57.49948385550241170, -7.000000000000000888 ) ) ;
#8630=CARTESIAN_POINT ( 'NONE',  ( 55.94051828345050836, 55.79948385550239465, -4.345558710429103577 ) ) ;
#8631=CARTESIAN_POINT ( 'NONE',  ( 50.02271294988505446, 56.50051614449766646, -7.000000000000000888 ) ) ;
#8634=CARTESIAN_POINT ( 'NONE',  ( 42.63976443033212860, 48.99948385550240459, 0.02388180880522514787 ) ) ;
#8637=CARTESIAN_POINT ( 'NONE',  ( 47.42335538002188144, 58.59948385550239891, 8.007379884777233059 ) ) ;
#8647=CARTESIAN_POINT ( 'NONE',  ( 48.02776887271750184, 57.60051614449765367, 5.992620115222795363 ) ) ;
#8649=CARTESIAN_POINT ( 'NONE',  ( 43.18075615816989199, 49.19948385550240744, -4.924951120819313743 ) ) ;
#8652=CARTESIAN_POINT ( 'NONE',  ( 54.72065718078918906, 56.70051614449766930, -6.458785618021089192 ) ) ;
#8667=CARTESIAN_POINT ( 'NONE',  ( 46.49166364869460466, 50.69948385550240744, 4.867452303228209765 ) ) ;
#8670=CARTESIAN_POINT ( 'NONE',  ( 42.38452918213190657, 45.90051614449766504, 2.450534656007115508 ) ) ;
#8673=CARTESIAN_POINT ( 'NONE',  ( 50.02271294988505446, 58.50051614449765935, -7.000000000000000888 ) ) ;
#8674=CARTESIAN_POINT ( 'NONE',  ( 44.28664221472220675, 63.09948385550240602, -1.832500667257165317 ) ) ;
#8684=CARTESIAN_POINT ( 'NONE',  ( 43.34962307344081012, 50.89948385550241028, 2.184720259617164650 ) ) ;
#8686=CARTESIAN_POINT ( 'NONE',  ( 44.91013252490150620, 60.20051614449766220, -3.727524721679154940 ) ) ;
#8690=CARTESIAN_POINT ( 'NONE',  ( 54.09612160359786515, 59.69948385550240033, -5.676469297603166098 ) ) ;
#8700=CARTESIAN_POINT ( 'NONE',  ( 56.66441430157296821, 54.09948385550240602, 2.141517661632100111 ) ) ;
#8701=CARTESIAN_POINT ( 'NONE',  ( 54.09612160359792199, 55.30051614449765651, 5.676469297603124353 ) ) ;
#8704=CARTESIAN_POINT ( 'NONE',  ( 45.86712807150323812, 49.29948385550240175, -5.649768623646098220 ) ) ;
#8706=CARTESIAN_POINT ( 'NONE',  ( 41.58830220609386430, 62.99948385550241170, 0.02388180880523263147 ) ) ;
#8715=CARTESIAN_POINT ( 'NONE',  ( 51.92680522751238925, 55.40051614449767214, 6.007379884777208190 ) ) ;
#8719=CARTESIAN_POINT ( 'NONE',  ( 42.39856655714566358, 52.89948385550241028, 2.493737253992119207 ) ) ;
#8720=CARTESIAN_POINT ( 'NONE',  ( 44.03140696652192787, 59.19948385550238612, -4.306917132069425058 ) ) ;
#8725=CARTESIAN_POINT ( 'NONE',  ( 50.02271294988505446, 60.50051614449766646, -8.000000000000001776 ) ) ;
#8737=CARTESIAN_POINT ( 'NONE',  ( 46.49166364869460466, 56.69948385550240744, 4.867452303228209765 ) ) ;
#8738=CARTESIAN_POINT ( 'NONE',  ( 57.36023556966787851, 47.00051614449765935, 0.02388180880515038476 ) ) ;
#8739=CARTESIAN_POINT ( 'NONE',  ( 57.60143344285435774, 51.10051614449766078, 2.493737253992045044 ) ) ;
#8742=CARTESIAN_POINT ( 'NONE',  ( 50.02271294988505446, 54.50051614449765935, -7.000000000000000888 ) ) ;
#8749=CARTESIAN_POINT ( 'NONE',  ( 43.34962307344081012, 58.89948385550241028, 2.184720259617164650 ) ) ;
#8751=CARTESIAN_POINT ( 'NONE',  ( 51.92680522751238925, 55.40051614449767214, 6.007379884777208190 ) ) ;
#8756=CARTESIAN_POINT ( 'NONE',  ( 54.09612160359786515, 63.69948385550240744, -5.676469297603166098 ) ) ;
#8768=CARTESIAN_POINT ( 'NONE',  ( 56.66441430157296821, 52.09948385550240602, 2.141517661632100111 ) ) ;
#8769=CARTESIAN_POINT ( 'NONE',  ( 55.96859303347802239, 52.80051614449764941, -4.306917132069484566 ) ) ;
#8771=CARTESIAN_POINT ( 'NONE',  ( 43.34962307344081012, 50.89948385550241028, 2.184720259617164650 ) ) ;
#8773=CARTESIAN_POINT ( 'NONE',  ( 54.09612160359786515, 45.69948385550240744, -5.676469297603166098 ) ) ;
#8781=CARTESIAN_POINT ( 'NONE',  ( 44.91013252490150620, 56.20051614449766220, -3.727524721679154940 ) ) ;
#8783=CARTESIAN_POINT ( 'NONE',  ( 54.72065718078924590, 50.29948385550240886, 6.458785618021043895 ) ) ;
#8784=CARTESIAN_POINT ( 'NONE',  ( 52.29715082351547295, 56.39948385550238896, 6.992620115222774047 ) ) ;
#8786=CARTESIAN_POINT ( 'NONE',  ( 41.58830220609386430, 62.00051614449766646, -0.02388180880514929535 ) ) ;
#8789=ORIENTED_EDGE ( 'NONE', *, *, #22, .F. ) ;
#8796=CARTESIAN_POINT ( 'NONE',  ( 44.30067958973596376, 58.89948385550241028, 1.875703265242204099 ) ) ;
#8797=CARTESIAN_POINT ( 'NONE',  ( 47.74827507625470702, 48.40051614449765793, -7.007379884777204637 ) ) ;
#8798=CARTESIAN_POINT ( 'NONE',  ( 47.37792948025170858, 55.60051614449765367, 7.992620115222797139 ) ) ;
#8803=CARTESIAN_POINT ( 'NONE',  ( 43.34962307344078880, 62.10051614449766078, -2.184720259617096705 ) ) ;
#8804=MECHANICAL_DESIGN_GEOMETRIC_PRESENTATION_REPRESENTATION('',(#397),#5062);
#8816=CARTESIAN_POINT ( 'NONE',  ( 50.02271294988512551, 54.49948385550240459, 7.000000000000000888 ) ) ;
#8817=CARTESIAN_POINT ( 'NONE',  ( 48.07319477248762496, 56.40051614449765793, -6.007379884777208190 ) ) ;
#8819=STYLED_ITEM ( 'NONE', ( #2811 ), #383 ) ;
#8821=CARTESIAN_POINT ( 'NONE',  ( 50.02271294988505446, 46.50051614449765935, -7.000000000000000888 ) ) ;
#8822=CARTESIAN_POINT ( 'NONE',  ( 53.54508667620428497, 46.29948385550240886, 4.840751629271157874 ) ) ;
#8834=SURFACE_SIDE_STYLE ('',( #1616 ) ) ;
#8837=CARTESIAN_POINT ( 'NONE',  ( 52.25172492374527877, 53.40051614449765793, 7.007379884777203749 ) ) ;
#8839=CARTESIAN_POINT ( 'NONE',  ( 50.02271294988512551, 52.49948385550240459, 7.000000000000000888 ) ) ;
#8840=CARTESIAN_POINT ( 'NONE',  ( 47.70284917648453415, 49.39948385550238896, -6.992620115222774047 ) ) ;
#8842=CARTESIAN_POINT ( 'NONE',  ( 57.60143344285433642, 61.89948385550241738, -2.493737253992118319 ) ) ;
#8851=CARTESIAN_POINT ( 'NONE',  ( 55.11794222512599362, 56.80051614449764941, -3.688883143319583446 ) ) ;
#8854=CARTESIAN_POINT ( 'NONE',  ( 42.38452918213188525, 53.09948385550240602, -2.450534656007040013 ) ) ;
#8855=CARTESIAN_POINT ( 'NONE',  ( 43.33558569842703179, 57.09948385550240602, -2.141517661632099223 ) ) ;
#8857=CARTESIAN_POINT ( 'NONE',  ( 42.39856655714564226, 64.10051614449766078, -2.493737253992044156 ) ) ;
#8868=CARTESIAN_POINT ( 'NONE',  ( 55.11794222512601493, 56.19948385550240744, 3.688883143319541702 ) ) ;
#8869=CARTESIAN_POINT ( 'NONE',  ( 49.97728705011495265, 47.50051614449766646, 7.000000000000000888 ) ) ;
#8871=CARTESIAN_POINT ( 'NONE',  ( 49.97728705011495265, 55.50051614449766646, 8.000000000000001776 ) ) ;
#8876=CARTESIAN_POINT ( 'NONE',  ( 41.58830220609386430, 46.00051614449764514, -0.02388180880514929535 ) ) ;
#8887=CARTESIAN_POINT ( 'NONE',  ( 50.02271294988512551, 60.49948385550240459, 7.000000000000000888 ) ) ;
#8888=CARTESIAN_POINT ( 'NONE',  ( 55.69932041026405045, 57.10051614449766788, 1.875703265242156359 ) ) ;
#8893=CARTESIAN_POINT ( 'NONE',  ( 44.30067958973594955, 62.10051614449765367, -1.875703265242155693 ) ) ;
#8894=CARTESIAN_POINT ( 'NONE',  ( 56.30877334542961421, 45.99948385550240459, -0.02388180880520959434 ) ) ;
#8901=ORIENTED_EDGE ( 'NONE', *, *, #4185, .T. ) ;
#8908=CARTESIAN_POINT ( 'NONE',  ( 43.34962307344078880, 52.10051614449766078, -2.184720259617096705 ) ) ;
#8911=CARTESIAN_POINT ( 'NONE',  ( 47.74827507625478518, 50.59948385550238470, 7.007379884777227730 ) ) ;
#8912=CARTESIAN_POINT ( 'NONE',  ( 57.61547081786812896, 60.09948385550240602, 2.450534656007040901 ) ) ;
#8922=CARTESIAN_POINT ( 'NONE',  ( 46.49166364869456913, 52.30051614449766362, -4.867452303228181343 ) ) ;
#8924=CARTESIAN_POINT ( 'NONE',  ( 43.18075615816989199, 53.19948385550240744, -4.924951120819313743 ) ) ;
#8925=CARTESIAN_POINT ( 'NONE',  ( 49.97728705011488159, 55.49948385550240459, -7.000000000000000888 ) ) ;
#8929=CARTESIAN_POINT ( 'NONE',  ( 57.60143344285433642, 45.89948385550240317, -2.493737253992118319 ) ) ;
#8938=CARTESIAN_POINT ( 'NONE',  ( 43.69122665457040000, 56.99948385550241170, 0.02388180880521036456 ) ) ;
#8939=CARTESIAN_POINT ( 'NONE',  ( 47.70284917648459810, 47.60051614449766078, 6.992620115222797139 ) ) ;
#8941=CARTESIAN_POINT ( 'NONE',  ( 57.61547081786810764, 52.90051614449766504, -2.450534656007114176 ) ) ;
#8944=CARTESIAN_POINT ( 'NONE',  ( 47.42335538002180328, 46.40051614449765793, -8.007379884777206414 ) ) ;
#8951=CARTESIAN_POINT ( 'NONE',  ( 44.03140696652192787, 57.19948385550238612, -4.306917132069425058 ) ) ;
#8953=CARTESIAN_POINT ( 'NONE',  ( 50.02271294988506156, 58.50051614449765225, -6.000000000000000888 ) ) ;
#8956=CARTESIAN_POINT ( 'NONE',  ( 47.70284917648459100, 47.60051614449763946, 6.992620115222796251 ) ) ;
#8957=CARTESIAN_POINT ( 'NONE',  ( 49.97728705011488159, 65.49948385550240459, -7.000000000000000888 ) ) ;
#8968=CARTESIAN_POINT ( 'NONE',  ( 52.29715082351538769, 58.60051614449766078, -6.992620115222796251 ) ) ;
#8971=CARTESIAN_POINT ( 'NONE',  ( 56.66441430157296821, 60.09948385550240602, 2.141517661632100111 ) ) ;
#8972=CARTESIAN_POINT ( 'NONE',  ( 49.97728705011488159, 47.49948385550240459, -7.000000000000000888 ) ) ;
#8974=CARTESIAN_POINT ( 'NONE',  ( 57.60143344285433642, 59.89948385550240317, -2.493737253992118319 ) ) ;
#8982=CARTESIAN_POINT ( 'NONE',  ( 56.30877334542961421, 59.00051614449766646, 0.02388180880515774693 ) ) ;
#8985=CARTESIAN_POINT ( 'NONE',  ( 57.61547081786812896, 52.09948385550241312, 2.450534656007040901 ) ) ;
#8987=CARTESIAN_POINT ( 'NONE',  ( 45.86712807150323812, 57.29948385550240175, -5.649768623646098220 ) ) ;
#8989=CARTESIAN_POINT ( 'NONE',  ( 43.18075615816994173, 61.80051614449766362, 4.924951120819380357 ) ) ;
#8999=CARTESIAN_POINT ( 'NONE',  ( 43.69122665457040000, 54.99948385550239749, 0.02388180880521036456 ) ) ;
#9000=CARTESIAN_POINT ( 'NONE',  ( 45.90387839640208512, 54.30051614449765651, -5.676469297603124353 ) ) ;
#9001=CARTESIAN_POINT ( 'NONE',  ( 50.02271294988505446, 50.50051614449765935, -8.000000000000001776 ) ) ;
#9004=CARTESIAN_POINT ( 'NONE',  ( 58.41169779390614281, 45.00051614449765225, 0.02388180880515032231 ) ) ;
#9013=CARTESIAN_POINT ( 'NONE',  ( 54.13287192849676188, 58.29948385550240175, 5.649768623646098220 ) ) ;
#9015=CARTESIAN_POINT ( 'NONE',  ( 55.94051828345050836, 49.79948385550240175, -4.345558710429103577 ) ) ;
#9017=EDGE_CURVE ( 'NONE', #725, #5739, #9554, .T. ) ;
#9021=CARTESIAN_POINT ( 'NONE',  ( 57.36023556966787851, 47.00051614449764514, 0.02388180880515038476 ) ) ;
#9022=CARTESIAN_POINT ( 'NONE',  ( 55.11794222512601493, 46.19948385550240744, 3.688883143319541702 ) ) ;
#9034=CARTESIAN_POINT ( 'NONE',  ( 45.86712807150329496, 57.70051614449765509, 5.649768623646139964 ) ) ;
#9038=CARTESIAN_POINT ( 'NONE',  ( 57.36023556966787851, 59.99948385550240459, -0.02388180880522424582 ) ) ;
#9039=CARTESIAN_POINT ( 'NONE',  ( 56.65037692655918988, 47.89948385550240317, -2.184720259617163762 ) ) ;
#9041=CARTESIAN_POINT ( 'NONE',  ( 50.02271294988512551, 48.49948385550240459, 7.000000000000000888 ) ) ;
#9051=CARTESIAN_POINT ( 'NONE',  ( 53.50833635130544508, 59.30051614449766362, 4.867452303228181343 ) ) ;
#9053=CARTESIAN_POINT ( 'NONE',  ( 43.18075615816989199, 61.19948385550241454, -4.924951120819313743 ) ) ;
#9055=CARTESIAN_POINT ( 'NONE',  ( 47.74827507625478518, 64.59948385550239891, 7.007379884777227730 ) ) ;
#9058=CARTESIAN_POINT ( 'NONE',  ( 57.61547081786812896, 52.09948385550241312, 2.450534656007040901 ) ) ;
#9073=CARTESIAN_POINT ( 'NONE',  ( 56.30877334542961421, 61.99948385550241170, -0.02388180880520959434 ) ) ;
#9074=CARTESIAN_POINT ( 'NONE',  ( 55.94051828345054389, 55.20051614449766220, 4.345558710429044957 ) ) ;
#9075=CARTESIAN_POINT ( 'NONE',  ( 42.39856655714564226, 62.10051614449765367, -2.493737253992044156 ) ) ;
#9078=CARTESIAN_POINT ( 'NONE',  ( 54.09612160359792199, 61.30051614449766362, 5.676469297603124353 ) ) ;
#9087=CARTESIAN_POINT ( 'NONE',  ( 52.25172492374522903, 61.59948385550239891, -7.007379884777225953 ) ) ;
#9088=CARTESIAN_POINT ( 'NONE',  ( 47.74827507625477807, 60.59948385550239891, 7.007379884777229506 ) ) ;
#9092=CARTESIAN_POINT ( 'NONE',  ( 50.02271294988506156, 64.50051614449766646, -6.000000000000000888 ) ) ;
#9093=CARTESIAN_POINT ( 'NONE',  ( 44.88205777487398507, 51.19948385550240744, -3.688883143319540814 ) ) ;
#9108=CARTESIAN_POINT ( 'NONE',  ( 44.03140696652198471, 61.80051614449767072, 4.306917132069485454 ) ) ;
#9110=CARTESIAN_POINT ( 'NONE',  ( 55.08986747509847248, 63.79948385550241596, -3.727524721679197572 ) ) ;
#9112=CARTESIAN_POINT ( 'NONE',  ( 47.70284917648453415, 61.39948385550241738, -6.992620115222774047 ) ) ;
#9113=CARTESIAN_POINT ( 'NONE',  ( 50.02271294988512551, 52.49948385550240459, 7.000000000000000888 ) ) ;
#9115=CARTESIAN_POINT ( 'NONE',  ( 43.34962307344081012, 50.89948385550241028, 2.184720259617164650 ) ) ;
#9124=CARTESIAN_POINT ( 'NONE',  ( 46.49166364869456913, 58.30051614449765651, -4.867452303228181343 ) ) ;
#9126=CARTESIAN_POINT ( 'NONE',  ( 45.27934281921075410, 57.29948385550240175, -6.458785618021043895 ) ) ;
#9127=CARTESIAN_POINT ( 'NONE',  ( 52.25172492374522903, 63.59948385550237759, -7.007379884777225953 ) ) ;
#9129=EDGE_CURVE ( 'NONE', #7204, #3958, #8234, .T. ) ;
#9130=CARTESIAN_POINT ( 'NONE',  ( 47.37792948025162332, 51.39948385550241028, -7.992620115222770494 ) ) ;
#9141=CARTESIAN_POINT ( 'NONE',  ( 44.88205777487398507, 61.19948385550241454, -3.688883143319540814 ) ) ;
#9142=CARTESIAN_POINT ( 'NONE',  ( 54.09612160359792199, 55.30051614449765651, 5.676469297603124353 ) ) ;
#9144=CARTESIAN_POINT ( 'NONE',  ( 43.20883090819742023, 56.20051614449766220, -4.963592699178938972 ) ) ;
#9148=CARTESIAN_POINT ( 'NONE',  ( 52.62207051974829852, 52.60051614449765367, -7.992620115222797139 ) ) ;
#9158=CARTESIAN_POINT ( 'NONE',  ( 43.33558569842703179, 63.09948385550240602, -2.141517661632099223 ) ) ;
#9159=CARTESIAN_POINT ( 'NONE',  ( 44.05948171654949874, 56.79948385550239465, 4.345558710429104465 ) ) ;
#9166=CARTESIAN_POINT ( 'NONE',  ( 43.33558569842706021, 53.90051614449765793, 2.141517661632167169 ) ) ;
#9167=CARTESIAN_POINT ( 'NONE',  ( 56.30877334542961421, 53.99948385550241170, -0.02388180880520959434 ) ) ;
#9179=CARTESIAN_POINT ( 'NONE',  ( 55.11794222512599362, 46.80051614449766362, -3.688883143319583446 ) ) ;
#9181=CARTESIAN_POINT ( 'NONE',  ( 45.90387839640214196, 58.69948385550240033, 5.676469297603166098 ) ) ;
#9182=CARTESIAN_POINT ( 'NONE',  ( 47.74827507625478518, 52.59948385550239180, 7.007379884777227730 ) ) ;
#9184=CARTESIAN_POINT ( 'NONE',  ( 56.65037692655918988, 51.89948385550241028, -2.184720259617163762 ) ) ;
#9193=CARTESIAN_POINT ( 'NONE',  ( 48.02776887271750184, 61.60051614449765367, 5.992620115222795363 ) ) ;
#9197=CARTESIAN_POINT ( 'NONE',  ( 43.18075615816989199, 59.19948385550240744, -4.924951120819313743 ) ) ;
#9198=CARTESIAN_POINT ( 'NONE',  ( 49.97728705011488159, 61.49948385550240459, -7.000000000000000888 ) ) ;
#9200=CARTESIAN_POINT ( 'NONE',  ( 58.41169779390614281, 51.99948385550239749, -0.02388180880523160798 ) ) ;
#9212=CARTESIAN_POINT ( 'NONE',  ( 55.08986747509847248, 61.79948385550240175, -3.727524721679197572 ) ) ;
#9213=CARTESIAN_POINT ( 'NONE',  ( 49.97728705011495265, 55.50051614449766646, 7.000000000000000888 ) ) ;
#9214=CARTESIAN_POINT ( 'NONE',  ( 56.81924384183006538, 60.80051614449766362, -4.924951120819380357 ) ) ;
#9216=CARTESIAN_POINT ( 'NONE',  ( 42.39856655714564226, 50.10051614449766078, -2.493737253992044156 ) ) ;
#9225=CARTESIAN_POINT ( 'NONE',  ( 43.34962307344081012, 64.89948385550239607, 2.184720259617164650 ) ) ;
#9226=CARTESIAN_POINT ( 'NONE',  ( 54.09612160359786515, 61.69948385550240744, -5.676469297603166098 ) ) ;
#9231=CARTESIAN_POINT ( 'NONE',  ( 43.34962307344078880, 54.10051614449766788, -2.184720259617096705 ) ) ;
#9232=CARTESIAN_POINT ( 'NONE',  ( 55.08986747509847248, 49.79948385550240175, -3.727524721679197572 ) ) ;
#9233=CARTESIAN_POINT ( 'NONE',  ( 55.48859070151218020, 45.00000000000002132, -4.999999999999993783 ) ) ;
#9247=CARTESIAN_POINT ( 'NONE',  ( 55.69932041026405045, 47.10051614449766078, 1.875703265242156359 ) ) ;
#9249=CARTESIAN_POINT ( 'NONE',  ( 52.29715082351547295, 58.39948385550238896, 6.992620115222774047 ) ) ;
#9250=CARTESIAN_POINT ( 'NONE',  ( 49.97728705011488159, 55.49948385550240459, -7.000000000000000888 ) ) ;
#9253=CARTESIAN_POINT ( 'NONE',  ( 55.94051828345050836, 47.79948385550240886, -4.345558710429104465 ) ) ;
#9263=CARTESIAN_POINT ( 'NONE',  ( 55.08986747509849380, 63.20051614449766220, 3.727524721679155384 ) ) ;
#9267=CARTESIAN_POINT ( 'NONE',  ( 50.02271294988513972, 60.49948385550240459, 8.000000000000001776 ) ) ;
#9270=CARTESIAN_POINT ( 'NONE',  ( 42.39856655714566358, 50.89948385550240317, 2.493737253992119207 ) ) ;
#9281=CARTESIAN_POINT ( 'NONE',  ( 51.97223112728249816, 44.60051614449766078, -5.992620115222793586 ) ) ;
#9282=CARTESIAN_POINT ( 'NONE',  ( 57.36023556966787851, 51.00051614449765225, 0.02388180880515038476 ) ) ;
#9283=CARTESIAN_POINT ( 'NONE',  ( 49.97728705011495265, 57.50051614449766646, 8.000000000000001776 ) ) ;
#9285=CARTESIAN_POINT ( 'NONE',  ( 56.81924384183006538, 50.80051614449766362, -4.924951120819380357 ) ) ;
#9295=CARTESIAN_POINT ( 'NONE',  ( 55.69932041026404335, 45.89948385550240317, -1.875703265242203432 ) ) ;
#9296=CARTESIAN_POINT ( 'NONE',  ( 55.94051828345050836, 61.79948385550240175, -4.345558710429103577 ) ) ;
#9301=CARTESIAN_POINT ( 'NONE',  ( 54.09612160359792199, 51.30051614449766362, 5.676469297603124353 ) ) ;
#9302=CARTESIAN_POINT ( 'NONE',  ( 55.11794222512601493, 54.19948385550241454, 3.688883143319541702 ) ) ;
#9316=CARTESIAN_POINT ( 'NONE',  ( 51.92680522751238925, 45.40051614449765793, 6.007379884777208190 ) ) ;
#9319=CARTESIAN_POINT ( 'NONE',  ( 50.02271294988512551, 64.49948385550240459, 7.000000000000000888 ) ) ;
#9320=CARTESIAN_POINT ( 'NONE',  ( 45.90387839640214196, 50.69948385550240744, 5.676469297603166098 ) ) ;
#9326=CARTESIAN_POINT ( 'NONE',  ( 55.96859303347804371, 48.19948385550240033, 4.306917132069425946 ) ) ;
#9335=CARTESIAN_POINT ( 'NONE',  ( 54.13287192849671214, 44.70051614449766220, -5.649768623646139964 ) ) ;
#9337=CARTESIAN_POINT ( 'NONE',  ( 58.41169779390614281, 59.99948385550241170, -0.02388180880523160798 ) ) ;
#9339=CARTESIAN_POINT ( 'NONE',  ( 52.62207051974839089, 48.39948385550240317, 7.992620115222770494 ) ) ;
#9350=CARTESIAN_POINT ( 'NONE',  ( 55.71335778527780747, 62.09948385550240602, 1.832500667257165983 ) ) ;
#9351=CARTESIAN_POINT ( 'NONE',  ( 42.63976443033212149, 58.00051614449765225, -0.02388180880514948964 ) ) ;
#9352=CARTESIAN_POINT ( 'NONE',  ( 45.27934281921082516, 61.70051614449766220, 6.458785618021089192 ) ) ;
#9356=CARTESIAN_POINT ( 'NONE',  ( 56.79116909180259398, 49.20051614449766220, 4.963592699178938972 ) ) ;
#9361=( BOUNDED_SURFACE ( )  B_SPLINE_SURFACE ( 3, 2, ( 
 ( #3020, #9385, #11239, #2812, #6080, #13582, #1761, #6223, #5177, #10343, #4964, #13370, #1832, #7320, #8139, #12345, #2879, #7100, #11310, #10276, #786, #3982, #8210, #12413, #2372, #7509, #2308, #7646, #5507, #9646, #6355, #6547, #238, #11784, #11717, #4387, #10748, #1126, #3225, #10617, #1253, #5377, #9714, #4458, #2238, #10547, #6607, #11594, #39, #10808, #12811, #2106, #11652, #1198, #8684, #1058, #3288, #1325, #4264, #5308, #12877, #9583, #11852, #9513, #8482, #12684, #5572, #7383, #107, #4326, #7447, #3424, #10685, #6484, #13645, #4193, #8613, #5447, #170, #8417, #12743, #12622, #3157, #3355, #2172, #8548, #6417, #7577, #11152, #4665, #8816, #368, #5781, #2581, #3691, #9781, #494, #10043, #11083, #1391, #6806, #9976, #2722, #300, #7914, #13015, #6874, #11012, #12125, #9910, #12943, #5709, #7783, #4735, #13211, #3628, #2650, #8951, #1599, #4801, #3558, #6679, #11994, #13150, #3759, #7850, #5845, #556, #9013, #7982, #2511, #10877, #5643, #10948, #8749, #6744, #12194, #9848, #1533, #6944, #3489, #4528, #1463, #1670, #7713, #11918, #2440, #12061, #4596, #429, #8887, #13083, #5987, #8334, #7157, #11366, #12535, #1887, #11508, #13420, #906, #9087, #3064, #3963, #8262, #13563, #11429, #6130, #12261, #12465, #6198, #4040, #8192, #10326, #3001, #7084, #9158, #2860, #7229, #11293, #1954, #10395, #12396, #2794, #7300, #3830, #10189, #5912, #5087, #8054, #3894, #829, #5160, #7011, #9225, #10111, #697, #11219, #9365, #1816, #4110 ),
 ( #4947, #1742, #621, #13353, #9295, #2934, #13488, #8122, #4874, #12325, #13286, #6062, #10256, #767, #5019, #2153, #1178, #2287, #4310, #3134, #976, #7492, #12797, #6400, #1107, #7431, #4173, #11637, #9565, #4372, #5358, #10530, #11575, #8396, #2090, #10600, #8461, #8529, #9630, #86, #5227, #12729, #13626, #8593, #6531, #12604, #155, #9493, #7367, #222, #6271, #11698, #8667, #10668, #3271, #2221, #17, #10729, #6335, #6465, #1039, #3206, #7562, #5430, #3338, #4441, #11770, #1240, #5488, #9696, #12863, #3406, #7628, #5290, #2024, #4241, #10461, #9429, #12665, #9961, #412, #1309, #5693, #6592, #13196, #4650, #1517, #3678, #13069, #6794, #287, #479, #5763, #3614, #7765, #8999, #3745, #11832, #3474, #4720, #11902, #6662, #12927, #5832, #10863, #7835, #9893, #8868, #5624, #544, #4580, #11062, #8737, #2355, #10993, #8938, #11978, #13137, #12111, #12047, #7693, #10789, #2565, #7901, #2497, #10932, #3541, #4510, #6729, #2632, #6858, #1447, #1378, #2424, #8796, #1584, #12998, #4788, #10029, #5554, #9834, #9766, #353, #10174, #13471, #4999, #890, #13334, #10378, #605, #8034, #13267, #5142, #13402, #11204, #7210, #2988, #9141, #8247, #4858, #6999, #10096, #3881, #9212, #7067, #9073, #9350, #3948, #12311, #13545, #1797, #11135, #1655, #5972, #7140, #12246, #7966, #8177, #12381, #12178, #2915, #2703, #6045, #11415, #5899, #6928, #10237, #10308, #1935, #4021, #11348, #3815, #815, #12446, #6114, #750, #1870, #5067, #8107, #1725, #4929 ),
 ( #2778, #9281, #6182, #676, #2844, #11278, #5474, #6384, #7477, #9615, #5341, #12716, #6257, #6447, #11683, #9547, #1, #1228, #9678, #4095, #9416, #2204, #4156, #12587, #5214, #11751, #3118, #72, #2138, #11624, #11563, #6515, #10513, #3323, #956, #8317, #3257, #10650, #4224, #1164, #4358, #10581, #13614, #3049, #4292, #5410, #8445, #3188, #9476, #10448, #12651, #1089, #138, #7418, #7351, #8380, #1026, #8577, #5275, #10715, #12779, #7541, #2073, #2269, #12517, #6322, #7279, #8516, #11491, #2009, #2613, #6576, #269, #5537, #6839, #5676, #3457, #13120, #8922, #1361, #464, #10775, #12912, #2338, #9816, #1428, #12980, #1292, #11046, #9876, #4562, #12030, #7749, #4633, #6776, #5607, #7677, #10843, #10977, #336, #2546, #5743, #11956, #9749, #1566, #11815, #4491, #5814, #13049, #8715, #11885, #398, #4703, #2406, #3524, #203, #6647, #8781, #9943, #2478, #12091, #6712, #10913, #8851, #4424, #7611, #3594, #7816, #1495, #3660, #7886, #8647, #12845, #3389, #731, #11260, #13316, #13455, #9124, #4770, #10292, #8090, #7123, #10152, #13181, #8982, #11400, #4911, #9051, #586, #6026, #2827, #3930, #10010, #4984, #802, #11327, #1636, #7049, #10223, #2969, #2686, #10079, #657, #2760, #1781, #8160, #3864, #3721, #5952, #8017, #9193, #4004, #12296, #2898, #13388, #12365, #5052, #3796, #6911, #11116, #11186, #7948, #12226, #1850, #5880, #6100, #9263, #12161, #4838, #6981, #8231, #1921, #12431, #7196, #527, #13248, #1706, #4143, #5325, #6241 ),
 ( #12789, #1150, #9335, #8563, #4211, #8501, #126, #11666, #2125, #12501, #12703, #6435, #3243, #8364, #2191, #3174, #12765, #11548, #3308, #3034, #10434, #11470, #7530, #11611, #9403, #5398, #9603, #7336, #10635, #7261, #5196, #8300, #2062, #7401, #5262, #1994, #11738, #6369, #10499, #6164, #4076, #7465, #4347, #946, #60, #13598, #12572, #10364, #873, #10563, #5125, #1073, #9461, #9532, #3104, #13528, #6306, #8433, #1010, #12640, #4280, #10896, #10829, #4687, #3580, #1415, #6699, #2460, #7666, #11870, #9929, #5523, #5594, #9737, #5661, #2391, #8908, #384, #4549, #5464, #9803, #10705, #3647, #8769, #9865, #7803, #3510, #4618, #4412, #8837, #13035, #7735, #6632, #13103, #7869, #2256, #7599, #12014, #2326, #10764, #3376, #449, #1277, #11940, #323, #12964, #254, #6504, #8701, #1480, #12833, #1217, #2530, #6762, #1347, #10964, #5729, #9667, #11805, #188, #8631, #6564, #4479, #12900, #3444, #514, #8002, #5932, #911, #1690, #6897, #7931, #9034, #7231, #13233, #978, #3068, #2028, #12146, #8336, #5869, #8968, #10463, #2597, #3847, #5230, #11432, #10133, #13303, #10061, #7303, #13166, #641, #9996, #3778, #4112, #1957, #6968, #9431, #13566, #6201, #3003, #12467, #12213, #2742, #6274, #1621, #4892, #574, #10397, #11171, #13628, #5162, #9108, #1550, #8265, #6824, #4176, #9367, #12537, #11510, #12078, #11031, #4755, #5799, #3708, #2669, #11103, #4820, #289, #8400, #20, #2291, #8463, #3209, #9496, #2357, #7433, #158, #6468, #2223 ),
 ( #10671, #5490, #8532, #11578, #3139, #9768, #3273, #11639, #12667, #4374, #1180, #6533, #12606, #12799, #8670, #9699, #4245, #5432, #8595, #1311, #1041, #2156, #12731, #1109, #9632, #10731, #7495, #2092, #4312, #6403, #3340, #11834, #7564, #1242, #11772, #224, #3409, #10602, #5293, #5362, #9567, #7369, #88, #4443, #11700, #12865, #7632, #6337, #10533, #6594, #10792, #5556, #12113, #11064, #12049, #7695, #11904, #2499, #3680, #4583, #9001, #1380, #2634, #11980, #5627, #2705, #8739, #9963, #11138, #13139, #7838, #5765, #6731, #13198, #9836, #2567, #2426, #5695, #10032, #7903, #13070, #6930, #5834, #6861, #8941, #4722, #9896, #414, #12181, #7767, #6796, #10934, #1586, #4652, #1657, #546, #10995, #6664, #1520, #12930, #5901, #481, #4790, #3747, #7968, #10098, #10865, #4513, #3476, #355, #8871, #8798, #13000, #3543, #1450, #3616, #678, #9144, #1727, #8319, #13338, #6116, #12383, #8179, #8109, #3051, #7069, #13548, #11206, #4860, #9283, #4023, #753, #13473, #892, #2917, #5974, #13269, #10311, #11417, #5002, #13404, #6047, #2780, #10240, #7143, #2990, #3950, #3883, #10176, #11280, #8249, #1800, #7282, #5144, #4098, #4931, #10380, #7213, #2846, #6184, #11351, #11493, #9214, #2011, #7001, #12313, #1873, #6259, #817, #5069, #12520, #9352, #12450, #607, #1938, #9075, #3818, #8037, #12249, #9550, #3120, #3392, #2206, #1092, #7614, #8382, #12781, #5413, #12590, #3325, #140, #11686, #6386, #11818, #2340, #10450, #2076, #4360, #10516, #5277 ),
 ( #6450, #74, #206, #4294, #5217, #10717, #8518, #7543, #10584, #13616, #9419, #959, #5343, #9479, #1028, #10652, #3259, #8579, #4159, #1166, #1230, #11754, #6324, #7480, #9617, #7353, #11565, #3, #12718, #3191, #2272, #6518, #5476, #4227, #9680, #8447, #4427, #8649, #12847, #12653, #7420, #11626, #2141, #338, #3460, #7679, #7752, #5540, #8783, #466, #11887, #12033, #12093, #9751, #1295, #12982, #2615, #7951, #4705, #13123, #400, #271, #4493, #4564, #5746, #6650, #8985, #7818, #2549, #13183, #6778, #12164, #4635, #1568, #8719, #3723, #8854, #8924, #530, #6842, #10979, #12914, #3664, #11049, #7888, #13051, #1497, #5817, #11958, #9819, #3527, #10012, #2480, #4772, #6578, #3596, #2408, #10777, #10845, #1364, #5609, #9946, #6715, #10916, #1430, #5678, #9878, #6028, #4078, #11188, #3798, #10367, #1709, #8162, #733, #10224, #10154, #5127, #9126, #1923, #13251, #6914, #11329, #6102, #2830, #1852, #2971, #4987, #8020, #1639, #12367, #13457, #7052, #1783, #8093, #4840, #12298, #9197, #5055, #13390, #5955, #12228, #13318, #10295, #3866, #9337, #7199, #6167, #2762, #12433, #9267, #4913, #8235, #3934, #13531, #11263, #8302, #9053, #6983, #659, #2688, #2901, #7125, #875, #11403, #804, #11118, #4007, #5883, #10082, #589, #62, #11613, #5200, #5466, #4282, #3176, #9669, #10436, #1152, #3311, #9405, #6437, #6310, #13601, #10707, #3036, #8504, #191, #7468, #2128, #12705, #10502, #7532, #4145, #10566, #948, #7950, #4349, #11670, #7404 ),
 ( #9606, #4213, #10640, #8565, #6372, #8368, #1219, #12574, #3107, #4415, #2193, #7338, #1014, #3245, #12769, #11550, #1075, #12503, #2064, #5264, #11741, #8436, #7265, #9464, #12642, #5329, #11475, #6243, #9535, #5400, #128, #2259, #6506, #1996, #518, #8634, #257, #2532, #8704, #3446, #9740, #2601, #7669, #386, #6702, #5803, #12837, #6635, #12081, #7738, #3378, #8911, #10898, #5732, #8771, #11807, #7601, #9999, #3513, #11872, #12902, #4622, #1417, #6764, #2329, #13037, #13106, #9932, #4481, #5664, #8839, #1553, #1280, #2394, #12967, #1352, #9867, #10967, #11942, #6567, #4551, #10831, #3583, #6828, #2464, #1482, #7805, #451, #3650, #5596, #5525, #9805, #326, #10766, #12017, #4691, #7872, #11034, #10281, #7935, #13169, #6972, #791, #6153, #12353, #11315, #12284, #12149, #2672, #2747, #3918, #4823, #7182, #6008, #10210, #11389, #718, #10348, #2816, #13441, #6901, #1910, #7035, #7106, #12419, #5040, #4970, #11106, #1837, #9249, #2884, #11245, #9181, #6087, #5936, #8006, #1695, #3990, #10138, #8215, #2957, #1766, #1625, #4758, #5872, #9038, #8971, #8144, #10065, #11175, #13375, #3711, #577, #8078, #13236, #3782, #12217, #645, #4896, #9112, #13307, #3852, #7249, #933, #5249, #7325, #7387, #8487, #999, #4062, #10487, #12560, #10551, #4331, #8423, #7452, #1062, #12690, #9589, #8355, #11455, #1980, #2047, #13512, #3092, #3230, #6228, #6359, #6424, #8288, #9319, #11535, #10622, #2243, #11656, #2176, #12626, #12489, #3024, #6295, #44 ) ),
 .UNSPECIFIED., .T., .F., .F. ) 
 B_SPLINE_SURFACE_WITH_KNOTS ( ( 4, 3, 4 ),
 ( 3, 2, 2, 2, 2, 2, 2, 2, 2, 2, 2, 2, 2, 2, 2, 2, 2, 2, 2, 2, 2, 2, 2, 2, 2, 2, 2, 2, 2, 2, 2, 2, 2, 2, 2, 2, 2, 2, 2, 2, 2, 2, 2, 2, 2, 2, 2, 2, 2, 2, 2, 2, 2, 2, 2, 2, 2, 2, 2, 2, 2, 2, 2, 2, 2, 2, 2, 2, 2, 2, 2, 2, 2, 2, 2, 2, 2, 2, 2, 2, 2, 2, 2, 2, 2, 2, 2, 2, 2, 2, 2, 2, 2, 2, 2, 2, 2, 2, 2, 2, 3 ),
 ( 0.000000000000000000, 0.5000000000000000000, 1.000000000000000000 ),
 ( 0.000000000000000000, 0.01000000000000000021, 0.02000000000000000042, 0.02999999999999999889, 0.04000000000000000083, 0.05000000000000000278, 0.05999999999999999778, 0.07000000000000000666, 0.08000000000000000167, 0.08999999999999999667, 0.1000000000000000056, 0.1100000000000000006, 0.1199999999999999956, 0.1300000000000000044, 0.1400000000000000133, 0.1499999999999999944, 0.1600000000000000033, 0.1700000000000000122, 0.1799999999999999933, 0.1900000000000000022, 0.2000000000000000111, 0.2099999999999999922, 0.2200000000000000011, 0.2300000000000000100, 0.2399999999999999911, 0.2500000000000000000, 0.2600000000000000089, 0.2700000000000000178, 0.2800000000000000266, 0.2899999999999999800, 0.2999999999999999889, 0.3099999999999999978, 0.3200000000000000067, 0.3300000000000000155, 0.3400000000000000244, 0.3499999999999999778, 0.3599999999999999867, 0.3699999999999999956, 0.3800000000000000044, 0.3900000000000000133, 0.4000000000000000222, 0.4099999999999999756, 0.4199999999999999845, 0.4299999999999999933, 0.4400000000000000022, 0.4500000000000000111, 0.4600000000000000200, 0.4699999999999999734, 0.4799999999999999822, 0.4899999999999999911, 0.5000000000000000000, 0.5100000000000000089, 0.5200000000000000178, 0.5300000000000000266, 0.5400000000000000355, 0.5500000000000000444, 0.5600000000000000533, 0.5699999999999999512, 0.5799999999999999600, 0.5899999999999999689, 0.5999999999999999778, 0.6099999999999999867, 0.6199999999999999956, 0.6300000000000000044, 0.6400000000000000133, 0.6500000000000000222, 0.6600000000000000311, 0.6700000000000000400, 0.6800000000000000488, 0.6899999999999999467, 0.6999999999999999556, 0.7099999999999999645, 0.7199999999999999734, 0.7299999999999999822, 0.7399999999999999911, 0.7500000000000000000, 0.7600000000000000089, 0.7700000000000000178, 0.7800000000000000266, 0.7900000000000000355, 0.8000000000000000444, 0.8100000000000000533, 0.8199999999999999512, 0.8299999999999999600, 0.8399999999999999689, 0.8499999999999999778, 0.8599999999999999867, 0.8699999999999999956, 0.8800000000000000044, 0.8900000000000000133, 0.9000000000000000222, 0.9100000000000000311, 0.9200000000000000400, 0.9300000000000000488, 0.9399999999999999467, 0.9499999999999999556, 0.9599999999999999645, 0.9699999999999999734, 0.9799999999999999822, 0.9899999999999999911, 1.000000000000000000 ),
 .UNSPECIFIED. ) 
 GEOMETRIC_REPRESENTATION_ITEM ( )  RATIONAL_B_SPLINE_SURFACE ( (
 ( 1.000000000000000000, 0.9510565162951535312, 1.000000000000000000, 0.9510565162951535312, 1.000000000000000000, 0.9510565162951535312, 1.000000000000000000, 0.9510565162951535312, 1.000000000000000000, 0.9510565162951535312, 1.000000000000000000, 0.9510565162951535312, 1.000000000000000000, 0.9510565162951535312, 1.000000000000000000, 0.9510565162951535312, 1.000000000000000000, 0.9510565162951535312, 1.000000000000000000, 0.9510565162951535312, 1.000000000000000000, 0.9510565162951535312, 1.000000000000000000, 0.9510565162951535312, 1.000000000000000000, 0.9510565162951535312, 1.000000000000000000, 0.9510565162951535312, 1.000000000000000000, 0.9510565162951535312, 1.000000000000000000, 0.9510565162951535312, 1.000000000000000000, 0.9510565162951535312, 1.000000000000000000, 0.9510565162951535312, 1.000000000000000000, 0.9510565162951535312, 1.000000000000000000, 0.9510565162951535312, 1.000000000000000000, 0.9510565162951535312, 1.000000000000000000, 0.9510565162951535312, 1.000000000000000000, 0.9510565162951535312, 1.000000000000000000, 0.9510565162951535312, 1.000000000000000000, 0.9510565162951535312, 1.000000000000000000, 0.9510565162951535312, 1.000000000000000000, 0.9510565162951535312, 1.000000000000000000, 0.9510565162951535312, 1.000000000000000000, 0.9510565162951535312, 1.000000000000000000, 0.9510565162951535312, 1.000000000000000000, 0.9510565162951535312, 1.000000000000000000, 0.9510565162951535312, 1.000000000000000000, 0.9510565162951535312, 1.000000000000000000, 0.9510565162951535312, 1.000000000000000000, 0.9510565162951535312, 1.000000000000000000, 0.9510565162951535312, 1.000000000000000000, 0.9510565162951535312, 1.000000000000000000, 0.9510565162951535312, 1.000000000000000000, 0.9510565162951535312, 1.000000000000000000, 0.9510565162951535312, 1.000000000000000000, 0.9510565162951535312, 1.000000000000000000, 0.9510565162951535312, 1.000000000000000000, 0.9510565162951535312, 1.000000000000000000, 0.9510565162951535312, 1.000000000000000000, 0.9510565162951535312, 1.000000000000000000, 0.9510565162951535312, 1.000000000000000000, 0.9510565162951535312, 1.000000000000000000, 0.9510565162951535312, 1.000000000000000000, 0.9510565162951535312, 1.000000000000000000, 0.9510565162951535312, 1.000000000000000000, 0.9510565162951535312, 1.000000000000000000, 0.9510565162951535312, 1.000000000000000000, 0.9510565162951535312, 1.000000000000000000, 0.9510565162951535312, 1.000000000000000000, 0.9510565162951535312, 1.000000000000000000, 0.9510565162951535312, 1.000000000000000000, 0.9510565162951535312, 1.000000000000000000, 0.9510565162951535312, 1.000000000000000000, 0.9510565162951535312, 1.000000000000000000, 0.9510565162951535312, 1.000000000000000000, 0.9510565162951535312, 1.000000000000000000, 0.9510565162951535312, 1.000000000000000000, 0.9510565162951535312, 1.000000000000000000, 0.9510565162951535312, 1.000000000000000000, 0.9510565162951535312, 1.000000000000000000, 0.9510565162951535312, 1.000000000000000000, 0.9510565162951535312, 1.000000000000000000, 0.9510565162951535312, 1.000000000000000000, 0.9510565162951535312, 1.000000000000000000, 0.9510565162951535312, 1.000000000000000000, 0.9510565162951535312, 1.000000000000000000, 0.9510565162951535312, 1.000000000000000000, 0.9510565162951535312, 1.000000000000000000, 0.9510565162951535312, 1.000000000000000000, 0.9510565162951535312, 1.000000000000000000, 0.9510565162951535312, 1.000000000000000000, 0.9510565162951535312, 1.000000000000000000, 0.9510565162951535312, 1.000000000000000000, 0.9510565162951535312, 1.000000000000000000, 0.9510565162951535312, 1.000000000000000000, 0.9510565162951535312, 1.000000000000000000, 0.9510565162951535312, 1.000000000000000000, 0.9510565162951535312, 1.000000000000000000, 0.9510565162951535312, 1.000000000000000000, 0.9510565162951535312, 1.000000000000000000, 0.9510565162951535312, 1.000000000000000000, 0.9510565162951535312, 1.000000000000000000, 0.9510565162951535312, 1.000000000000000000, 0.9510565162951535312, 1.000000000000000000, 0.9510565162951535312, 1.000000000000000000, 0.9510565162951535312, 1.000000000000000000, 0.9510565162951535312, 1.000000000000000000, 0.9510565162951535312, 1.000000000000000000, 0.9510565162951535312, 1.000000000000000000, 0.9510565162951535312, 1.000000000000000000, 0.9510565162951535312, 1.000000000000000000, 0.9510565162951535312, 1.000000000000000000, 0.9510565162951535312, 1.000000000000000000, 0.9510565162951535312, 1.000000000000000000, 0.9510565162951535312, 1.000000000000000000),
 ( 0.3333333333333333703, 0.3170188387650512141, 0.3333333333333333703, 0.3170188387650512141, 0.3333333333333333703, 0.3170188387650512141, 0.3333333333333333703, 0.3170188387650512141, 0.3333333333333333703, 0.3170188387650512141, 0.3333333333333333703, 0.3170188387650512141, 0.3333333333333333703, 0.3170188387650512141, 0.3333333333333333703, 0.3170188387650512141, 0.3333333333333333703, 0.3170188387650512141, 0.3333333333333333703, 0.3170188387650512141, 0.3333333333333333703, 0.3170188387650512141, 0.3333333333333333703, 0.3170188387650512141, 0.3333333333333333703, 0.3170188387650512141, 0.3333333333333333703, 0.3170188387650512141, 0.3333333333333333703, 0.3170188387650512141, 0.3333333333333333703, 0.3170188387650512141, 0.3333333333333333703, 0.3170188387650512141, 0.3333333333333333703, 0.3170188387650512141, 0.3333333333333333703, 0.3170188387650512141, 0.3333333333333333703, 0.3170188387650512141, 0.3333333333333333703, 0.3170188387650512141, 0.3333333333333333703, 0.3170188387650512141, 0.3333333333333333703, 0.3170188387650512141, 0.3333333333333333703, 0.3170188387650512141, 0.3333333333333333703, 0.3170188387650512141, 0.3333333333333333703, 0.3170188387650512141, 0.3333333333333333703, 0.3170188387650512141, 0.3333333333333333703, 0.3170188387650512141, 0.3333333333333333703, 0.3170188387650512141, 0.3333333333333333703, 0.3170188387650512141, 0.3333333333333333703, 0.3170188387650512141, 0.3333333333333333703, 0.3170188387650512141, 0.3333333333333333703, 0.3170188387650512141, 0.3333333333333333703, 0.3170188387650512141, 0.3333333333333333703, 0.3170188387650512141, 0.3333333333333333703, 0.3170188387650512141, 0.3333333333333333703, 0.3170188387650512141, 0.3333333333333333703, 0.3170188387650512141, 0.3333333333333333703, 0.3170188387650512141, 0.3333333333333333703, 0.3170188387650512141, 0.3333333333333333703, 0.3170188387650512141, 0.3333333333333333703, 0.3170188387650512141, 0.3333333333333333703, 0.3170188387650512141, 0.3333333333333333703, 0.3170188387650512141, 0.3333333333333333703, 0.3170188387650512141, 0.3333333333333333703, 0.3170188387650512141, 0.3333333333333333703, 0.3170188387650512141, 0.3333333333333333703, 0.3170188387650512141, 0.3333333333333333703, 0.3170188387650512141, 0.3333333333333333703, 0.3170188387650512141, 0.3333333333333333703, 0.3170188387650512141, 0.3333333333333333703, 0.3170188387650512141, 0.3333333333333333703, 0.3170188387650512141, 0.3333333333333333703, 0.3170188387650512141, 0.3333333333333333703, 0.3170188387650512141, 0.3333333333333333703, 0.3170188387650512141, 0.3333333333333333703, 0.3170188387650512141, 0.3333333333333333703, 0.3170188387650512141, 0.3333333333333333703, 0.3170188387650512141, 0.3333333333333333703, 0.3170188387650512141, 0.3333333333333333703, 0.3170188387650512141, 0.3333333333333333703, 0.3170188387650512141, 0.3333333333333333703, 0.3170188387650512141, 0.3333333333333333703, 0.3170188387650512141, 0.3333333333333333703, 0.3170188387650512141, 0.3333333333333333703, 0.3170188387650512141, 0.3333333333333333703, 0.3170188387650512141, 0.3333333333333333703, 0.3170188387650512141, 0.3333333333333333703, 0.3170188387650512141, 0.3333333333333333703, 0.3170188387650512141, 0.3333333333333333703, 0.3170188387650512141, 0.3333333333333333703, 0.3170188387650512141, 0.3333333333333333703, 0.3170188387650512141, 0.3333333333333333703, 0.3170188387650512141, 0.3333333333333333703, 0.3170188387650512141, 0.3333333333333333703, 0.3170188387650512141, 0.3333333333333333703, 0.3170188387650512141, 0.3333333333333333703, 0.3170188387650512141, 0.3333333333333333703, 0.3170188387650512141, 0.3333333333333333703, 0.3170188387650512141, 0.3333333333333333703, 0.3170188387650512141, 0.3333333333333333703, 0.3170188387650512141, 0.3333333333333333703, 0.3170188387650512141, 0.3333333333333333703, 0.3170188387650512141, 0.3333333333333333703, 0.3170188387650512141, 0.3333333333333333703, 0.3170188387650512141, 0.3333333333333333703, 0.3170188387650512141, 0.3333333333333333703, 0.3170188387650512141, 0.3333333333333333703, 0.3170188387650512141, 0.3333333333333333703, 0.3170188387650512141, 0.3333333333333333703, 0.3170188387650512141, 0.3333333333333333703, 0.3170188387650512141, 0.3333333333333333703, 0.3170188387650512141, 0.3333333333333333703, 0.3170188387650512141, 0.3333333333333333703, 0.3170188387650512141, 0.3333333333333333703, 0.3170188387650512141, 0.3333333333333333703, 0.3170188387650512141, 0.3333333333333333703, 0.3170188387650512141, 0.3333333333333333703, 0.3170188387650512141, 0.3333333333333333703, 0.3170188387650512141, 0.3333333333333333703),
 ( 0.3333333333333333703, 0.3170188387650512141, 0.3333333333333333703, 0.3170188387650512141, 0.3333333333333333703, 0.3170188387650512141, 0.3333333333333333703, 0.3170188387650512141, 0.3333333333333333703, 0.3170188387650512141, 0.3333333333333333703, 0.3170188387650512141, 0.3333333333333333703, 0.3170188387650512141, 0.3333333333333333703, 0.3170188387650512141, 0.3333333333333333703, 0.3170188387650512141, 0.3333333333333333703, 0.3170188387650512141, 0.3333333333333333703, 0.3170188387650512141, 0.3333333333333333703, 0.3170188387650512141, 0.3333333333333333703, 0.3170188387650512141, 0.3333333333333333703, 0.3170188387650512141, 0.3333333333333333703, 0.3170188387650512141, 0.3333333333333333703, 0.3170188387650512141, 0.3333333333333333703, 0.3170188387650512141, 0.3333333333333333703, 0.3170188387650512141, 0.3333333333333333703, 0.3170188387650512141, 0.3333333333333333703, 0.3170188387650512141, 0.3333333333333333703, 0.3170188387650512141, 0.3333333333333333703, 0.3170188387650512141, 0.3333333333333333703, 0.3170188387650512141, 0.3333333333333333703, 0.3170188387650512141, 0.3333333333333333703, 0.3170188387650512141, 0.3333333333333333703, 0.3170188387650512141, 0.3333333333333333703, 0.3170188387650512141, 0.3333333333333333703, 0.3170188387650512141, 0.3333333333333333703, 0.3170188387650512141, 0.3333333333333333703, 0.3170188387650512141, 0.3333333333333333703, 0.3170188387650512141, 0.3333333333333333703, 0.3170188387650512141, 0.3333333333333333703, 0.3170188387650512141, 0.3333333333333333703, 0.3170188387650512141, 0.3333333333333333703, 0.3170188387650512141, 0.3333333333333333703, 0.3170188387650512141, 0.3333333333333333703, 0.3170188387650512141, 0.3333333333333333703, 0.3170188387650512141, 0.3333333333333333703, 0.3170188387650512141, 0.3333333333333333703, 0.3170188387650512141, 0.3333333333333333703, 0.3170188387650512141, 0.3333333333333333703, 0.3170188387650512141, 0.3333333333333333703, 0.3170188387650512141, 0.3333333333333333703, 0.3170188387650512141, 0.3333333333333333703, 0.3170188387650512141, 0.3333333333333333703, 0.3170188387650512141, 0.3333333333333333703, 0.3170188387650512141, 0.3333333333333333703, 0.3170188387650512141, 0.3333333333333333703, 0.3170188387650512141, 0.3333333333333333703, 0.3170188387650512141, 0.3333333333333333703, 0.3170188387650512141, 0.3333333333333333703, 0.3170188387650512141, 0.3333333333333333703, 0.3170188387650512141, 0.3333333333333333703, 0.3170188387650512141, 0.3333333333333333703, 0.3170188387650512141, 0.3333333333333333703, 0.3170188387650512141, 0.3333333333333333703, 0.3170188387650512141, 0.3333333333333333703, 0.3170188387650512141, 0.3333333333333333703, 0.3170188387650512141, 0.3333333333333333703, 0.3170188387650512141, 0.3333333333333333703, 0.3170188387650512141, 0.3333333333333333703, 0.3170188387650512141, 0.3333333333333333703, 0.3170188387650512141, 0.3333333333333333703, 0.3170188387650512141, 0.3333333333333333703, 0.3170188387650512141, 0.3333333333333333703, 0.3170188387650512141, 0.3333333333333333703, 0.3170188387650512141, 0.3333333333333333703, 0.3170188387650512141, 0.3333333333333333703, 0.3170188387650512141, 0.3333333333333333703, 0.3170188387650512141, 0.3333333333333333703, 0.3170188387650512141, 0.3333333333333333703, 0.3170188387650512141, 0.3333333333333333703, 0.3170188387650512141, 0.3333333333333333703, 0.3170188387650512141, 0.3333333333333333703, 0.3170188387650512141, 0.3333333333333333703, 0.3170188387650512141, 0.3333333333333333703, 0.3170188387650512141, 0.3333333333333333703, 0.3170188387650512141, 0.3333333333333333703, 0.3170188387650512141, 0.3333333333333333703, 0.3170188387650512141, 0.3333333333333333703, 0.3170188387650512141, 0.3333333333333333703, 0.3170188387650512141, 0.3333333333333333703, 0.3170188387650512141, 0.3333333333333333703, 0.3170188387650512141, 0.3333333333333333703, 0.3170188387650512141, 0.3333333333333333703, 0.3170188387650512141, 0.3333333333333333703, 0.3170188387650512141, 0.3333333333333333703, 0.3170188387650512141, 0.3333333333333333703, 0.3170188387650512141, 0.3333333333333333703, 0.3170188387650512141, 0.3333333333333333703, 0.3170188387650512141, 0.3333333333333333703, 0.3170188387650512141, 0.3333333333333333703, 0.3170188387650512141, 0.3333333333333333703, 0.3170188387650512141, 0.3333333333333333703, 0.3170188387650512141, 0.3333333333333333703, 0.3170188387650512141, 0.3333333333333333703, 0.3170188387650512141, 0.3333333333333333703, 0.3170188387650512141, 0.3333333333333333703, 0.3170188387650512141, 0.3333333333333333703, 0.3170188387650512141, 0.3333333333333333703),
 ( 1.000000000000000000, 0.9510565162951535312, 1.000000000000000000, 0.9510565162951535312, 1.000000000000000000, 0.9510565162951535312, 1.000000000000000000, 0.9510565162951535312, 1.000000000000000000, 0.9510565162951535312, 1.000000000000000000, 0.9510565162951535312, 1.000000000000000000, 0.9510565162951535312, 1.000000000000000000, 0.9510565162951535312, 1.000000000000000000, 0.9510565162951535312, 1.000000000000000000, 0.9510565162951535312, 1.000000000000000000, 0.9510565162951535312, 1.000000000000000000, 0.9510565162951535312, 1.000000000000000000, 0.9510565162951535312, 1.000000000000000000, 0.9510565162951535312, 1.000000000000000000, 0.9510565162951535312, 1.000000000000000000, 0.9510565162951535312, 1.000000000000000000, 0.9510565162951535312, 1.000000000000000000, 0.9510565162951535312, 1.000000000000000000, 0.9510565162951535312, 1.000000000000000000, 0.9510565162951535312, 1.000000000000000000, 0.9510565162951535312, 1.000000000000000000, 0.9510565162951535312, 1.000000000000000000, 0.9510565162951535312, 1.000000000000000000, 0.9510565162951535312, 1.000000000000000000, 0.9510565162951535312, 1.000000000000000000, 0.9510565162951535312, 1.000000000000000000, 0.9510565162951535312, 1.000000000000000000, 0.9510565162951535312, 1.000000000000000000, 0.9510565162951535312, 1.000000000000000000, 0.9510565162951535312, 1.000000000000000000, 0.9510565162951535312, 1.000000000000000000, 0.9510565162951535312, 1.000000000000000000, 0.9510565162951535312, 1.000000000000000000, 0.9510565162951535312, 1.000000000000000000, 0.9510565162951535312, 1.000000000000000000, 0.9510565162951535312, 1.000000000000000000, 0.9510565162951535312, 1.000000000000000000, 0.9510565162951535312, 1.000000000000000000, 0.9510565162951535312, 1.000000000000000000, 0.9510565162951535312, 1.000000000000000000, 0.9510565162951535312, 1.000000000000000000, 0.9510565162951535312, 1.000000000000000000, 0.9510565162951535312, 1.000000000000000000, 0.9510565162951535312, 1.000000000000000000, 0.9510565162951535312, 1.000000000000000000, 0.9510565162951535312, 1.000000000000000000, 0.9510565162951535312, 1.000000000000000000, 0.9510565162951535312, 1.000000000000000000, 0.9510565162951535312, 1.000000000000000000, 0.9510565162951535312, 1.000000000000000000, 0.9510565162951535312, 1.000000000000000000, 0.9510565162951535312, 1.000000000000000000, 0.9510565162951535312, 1.000000000000000000, 0.9510565162951535312, 1.000000000000000000, 0.9510565162951535312, 1.000000000000000000, 0.9510565162951535312, 1.000000000000000000, 0.9510565162951535312, 1.000000000000000000, 0.9510565162951535312, 1.000000000000000000, 0.9510565162951535312, 1.000000000000000000, 0.9510565162951535312, 1.000000000000000000, 0.9510565162951535312, 1.000000000000000000, 0.9510565162951535312, 1.000000000000000000, 0.9510565162951535312, 1.000000000000000000, 0.9510565162951535312, 1.000000000000000000, 0.9510565162951535312, 1.000000000000000000, 0.9510565162951535312, 1.000000000000000000, 0.9510565162951535312, 1.000000000000000000, 0.9510565162951535312, 1.000000000000000000, 0.9510565162951535312, 1.000000000000000000, 0.9510565162951535312, 1.000000000000000000, 0.9510565162951535312, 1.000000000000000000, 0.9510565162951535312, 1.000000000000000000, 0.9510565162951535312, 1.000000000000000000, 0.9510565162951535312, 1.000000000000000000, 0.9510565162951535312, 1.000000000000000000, 0.9510565162951535312, 1.000000000000000000, 0.9510565162951535312, 1.000000000000000000, 0.9510565162951535312, 1.000000000000000000, 0.9510565162951535312, 1.000000000000000000, 0.9510565162951535312, 1.000000000000000000, 0.9510565162951535312, 1.000000000000000000, 0.9510565162951535312, 1.000000000000000000, 0.9510565162951535312, 1.000000000000000000, 0.9510565162951535312, 1.000000000000000000, 0.9510565162951535312, 1.000000000000000000, 0.9510565162951535312, 1.000000000000000000, 0.9510565162951535312, 1.000000000000000000, 0.9510565162951535312, 1.000000000000000000, 0.9510565162951535312, 1.000000000000000000, 0.9510565162951535312, 1.000000000000000000, 0.9510565162951535312, 1.000000000000000000, 0.9510565162951535312, 1.000000000000000000, 0.9510565162951535312, 1.000000000000000000, 0.9510565162951535312, 1.000000000000000000, 0.9510565162951535312, 1.000000000000000000, 0.9510565162951535312, 1.000000000000000000, 0.9510565162951535312, 1.000000000000000000, 0.9510565162951535312, 1.000000000000000000, 0.9510565162951535312, 1.000000000000000000, 0.9510565162951535312, 1.000000000000000000),
 ( 0.3333333333333333703, 0.3170188387650512141, 0.3333333333333333703, 0.3170188387650512141, 0.3333333333333333703, 0.3170188387650512141, 0.3333333333333333703, 0.3170188387650512141, 0.3333333333333333703, 0.3170188387650512141, 0.3333333333333333703, 0.3170188387650512141, 0.3333333333333333703, 0.3170188387650512141, 0.3333333333333333703, 0.3170188387650512141, 0.3333333333333333703, 0.3170188387650512141, 0.3333333333333333703, 0.3170188387650512141, 0.3333333333333333703, 0.3170188387650512141, 0.3333333333333333703, 0.3170188387650512141, 0.3333333333333333703, 0.3170188387650512141, 0.3333333333333333703, 0.3170188387650512141, 0.3333333333333333703, 0.3170188387650512141, 0.3333333333333333703, 0.3170188387650512141, 0.3333333333333333703, 0.3170188387650512141, 0.3333333333333333703, 0.3170188387650512141, 0.3333333333333333703, 0.3170188387650512141, 0.3333333333333333703, 0.3170188387650512141, 0.3333333333333333703, 0.3170188387650512141, 0.3333333333333333703, 0.3170188387650512141, 0.3333333333333333703, 0.3170188387650512141, 0.3333333333333333703, 0.3170188387650512141, 0.3333333333333333703, 0.3170188387650512141, 0.3333333333333333703, 0.3170188387650512141, 0.3333333333333333703, 0.3170188387650512141, 0.3333333333333333703, 0.3170188387650512141, 0.3333333333333333703, 0.3170188387650512141, 0.3333333333333333703, 0.3170188387650512141, 0.3333333333333333703, 0.3170188387650512141, 0.3333333333333333703, 0.3170188387650512141, 0.3333333333333333703, 0.3170188387650512141, 0.3333333333333333703, 0.3170188387650512141, 0.3333333333333333703, 0.3170188387650512141, 0.3333333333333333703, 0.3170188387650512141, 0.3333333333333333703, 0.3170188387650512141, 0.3333333333333333703, 0.3170188387650512141, 0.3333333333333333703, 0.3170188387650512141, 0.3333333333333333703, 0.3170188387650512141, 0.3333333333333333703, 0.3170188387650512141, 0.3333333333333333703, 0.3170188387650512141, 0.3333333333333333703, 0.3170188387650512141, 0.3333333333333333703, 0.3170188387650512141, 0.3333333333333333703, 0.3170188387650512141, 0.3333333333333333703, 0.3170188387650512141, 0.3333333333333333703, 0.3170188387650512141, 0.3333333333333333703, 0.3170188387650512141, 0.3333333333333333703, 0.3170188387650512141, 0.3333333333333333703, 0.3170188387650512141, 0.3333333333333333703, 0.3170188387650512141, 0.3333333333333333703, 0.3170188387650512141, 0.3333333333333333703, 0.3170188387650512141, 0.3333333333333333703, 0.3170188387650512141, 0.3333333333333333703, 0.3170188387650512141, 0.3333333333333333703, 0.3170188387650512141, 0.3333333333333333703, 0.3170188387650512141, 0.3333333333333333703, 0.3170188387650512141, 0.3333333333333333703, 0.3170188387650512141, 0.3333333333333333703, 0.3170188387650512141, 0.3333333333333333703, 0.3170188387650512141, 0.3333333333333333703, 0.3170188387650512141, 0.3333333333333333703, 0.3170188387650512141, 0.3333333333333333703, 0.3170188387650512141, 0.3333333333333333703, 0.3170188387650512141, 0.3333333333333333703, 0.3170188387650512141, 0.3333333333333333703, 0.3170188387650512141, 0.3333333333333333703, 0.3170188387650512141, 0.3333333333333333703, 0.3170188387650512141, 0.3333333333333333703, 0.3170188387650512141, 0.3333333333333333703, 0.3170188387650512141, 0.3333333333333333703, 0.3170188387650512141, 0.3333333333333333703, 0.3170188387650512141, 0.3333333333333333703, 0.3170188387650512141, 0.3333333333333333703, 0.3170188387650512141, 0.3333333333333333703, 0.3170188387650512141, 0.3333333333333333703, 0.3170188387650512141, 0.3333333333333333703, 0.3170188387650512141, 0.3333333333333333703, 0.3170188387650512141, 0.3333333333333333703, 0.3170188387650512141, 0.3333333333333333703, 0.3170188387650512141, 0.3333333333333333703, 0.3170188387650512141, 0.3333333333333333703, 0.3170188387650512141, 0.3333333333333333703, 0.3170188387650512141, 0.3333333333333333703, 0.3170188387650512141, 0.3333333333333333703, 0.3170188387650512141, 0.3333333333333333703, 0.3170188387650512141, 0.3333333333333333703, 0.3170188387650512141, 0.3333333333333333703, 0.3170188387650512141, 0.3333333333333333703, 0.3170188387650512141, 0.3333333333333333703, 0.3170188387650512141, 0.3333333333333333703, 0.3170188387650512141, 0.3333333333333333703, 0.3170188387650512141, 0.3333333333333333703, 0.3170188387650512141, 0.3333333333333333703, 0.3170188387650512141, 0.3333333333333333703, 0.3170188387650512141, 0.3333333333333333703, 0.3170188387650512141, 0.3333333333333333703, 0.3170188387650512141, 0.3333333333333333703, 0.3170188387650512141, 0.3333333333333333703, 0.3170188387650512141, 0.3333333333333333703),
 ( 0.3333333333333333703, 0.3170188387650512141, 0.3333333333333333703, 0.3170188387650512141, 0.3333333333333333703, 0.3170188387650512141, 0.3333333333333333703, 0.3170188387650512141, 0.3333333333333333703, 0.3170188387650512141, 0.3333333333333333703, 0.3170188387650512141, 0.3333333333333333703, 0.3170188387650512141, 0.3333333333333333703, 0.3170188387650512141, 0.3333333333333333703, 0.3170188387650512141, 0.3333333333333333703, 0.3170188387650512141, 0.3333333333333333703, 0.3170188387650512141, 0.3333333333333333703, 0.3170188387650512141, 0.3333333333333333703, 0.3170188387650512141, 0.3333333333333333703, 0.3170188387650512141, 0.3333333333333333703, 0.3170188387650512141, 0.3333333333333333703, 0.3170188387650512141, 0.3333333333333333703, 0.3170188387650512141, 0.3333333333333333703, 0.3170188387650512141, 0.3333333333333333703, 0.3170188387650512141, 0.3333333333333333703, 0.3170188387650512141, 0.3333333333333333703, 0.3170188387650512141, 0.3333333333333333703, 0.3170188387650512141, 0.3333333333333333703, 0.3170188387650512141, 0.3333333333333333703, 0.3170188387650512141, 0.3333333333333333703, 0.3170188387650512141, 0.3333333333333333703, 0.3170188387650512141, 0.3333333333333333703, 0.3170188387650512141, 0.3333333333333333703, 0.3170188387650512141, 0.3333333333333333703, 0.3170188387650512141, 0.3333333333333333703, 0.3170188387650512141, 0.3333333333333333703, 0.3170188387650512141, 0.3333333333333333703, 0.3170188387650512141, 0.3333333333333333703, 0.3170188387650512141, 0.3333333333333333703, 0.3170188387650512141, 0.3333333333333333703, 0.3170188387650512141, 0.3333333333333333703, 0.3170188387650512141, 0.3333333333333333703, 0.3170188387650512141, 0.3333333333333333703, 0.3170188387650512141, 0.3333333333333333703, 0.3170188387650512141, 0.3333333333333333703, 0.3170188387650512141, 0.3333333333333333703, 0.3170188387650512141, 0.3333333333333333703, 0.3170188387650512141, 0.3333333333333333703, 0.3170188387650512141, 0.3333333333333333703, 0.3170188387650512141, 0.3333333333333333703, 0.3170188387650512141, 0.3333333333333333703, 0.3170188387650512141, 0.3333333333333333703, 0.3170188387650512141, 0.3333333333333333703, 0.3170188387650512141, 0.3333333333333333703, 0.3170188387650512141, 0.3333333333333333703, 0.3170188387650512141, 0.3333333333333333703, 0.3170188387650512141, 0.3333333333333333703, 0.3170188387650512141, 0.3333333333333333703, 0.3170188387650512141, 0.3333333333333333703, 0.3170188387650512141, 0.3333333333333333703, 0.3170188387650512141, 0.3333333333333333703, 0.3170188387650512141, 0.3333333333333333703, 0.3170188387650512141, 0.3333333333333333703, 0.3170188387650512141, 0.3333333333333333703, 0.3170188387650512141, 0.3333333333333333703, 0.3170188387650512141, 0.3333333333333333703, 0.3170188387650512141, 0.3333333333333333703, 0.3170188387650512141, 0.3333333333333333703, 0.3170188387650512141, 0.3333333333333333703, 0.3170188387650512141, 0.3333333333333333703, 0.3170188387650512141, 0.3333333333333333703, 0.3170188387650512141, 0.3333333333333333703, 0.3170188387650512141, 0.3333333333333333703, 0.3170188387650512141, 0.3333333333333333703, 0.3170188387650512141, 0.3333333333333333703, 0.3170188387650512141, 0.3333333333333333703, 0.3170188387650512141, 0.3333333333333333703, 0.3170188387650512141, 0.3333333333333333703, 0.3170188387650512141, 0.3333333333333333703, 0.3170188387650512141, 0.3333333333333333703, 0.3170188387650512141, 0.3333333333333333703, 0.3170188387650512141, 0.3333333333333333703, 0.3170188387650512141, 0.3333333333333333703, 0.3170188387650512141, 0.3333333333333333703, 0.3170188387650512141, 0.3333333333333333703, 0.3170188387650512141, 0.3333333333333333703, 0.3170188387650512141, 0.3333333333333333703, 0.3170188387650512141, 0.3333333333333333703, 0.3170188387650512141, 0.3333333333333333703, 0.3170188387650512141, 0.3333333333333333703, 0.3170188387650512141, 0.3333333333333333703, 0.3170188387650512141, 0.3333333333333333703, 0.3170188387650512141, 0.3333333333333333703, 0.3170188387650512141, 0.3333333333333333703, 0.3170188387650512141, 0.3333333333333333703, 0.3170188387650512141, 0.3333333333333333703, 0.3170188387650512141, 0.3333333333333333703, 0.3170188387650512141, 0.3333333333333333703, 0.3170188387650512141, 0.3333333333333333703, 0.3170188387650512141, 0.3333333333333333703, 0.3170188387650512141, 0.3333333333333333703, 0.3170188387650512141, 0.3333333333333333703, 0.3170188387650512141, 0.3333333333333333703, 0.3170188387650512141, 0.3333333333333333703, 0.3170188387650512141, 0.3333333333333333703, 0.3170188387650512141, 0.3333333333333333703),
 ( 1.000000000000000000, 0.9510565162951535312, 1.000000000000000000, 0.9510565162951535312, 1.000000000000000000, 0.9510565162951535312, 1.000000000000000000, 0.9510565162951535312, 1.000000000000000000, 0.9510565162951535312, 1.000000000000000000, 0.9510565162951535312, 1.000000000000000000, 0.9510565162951535312, 1.000000000000000000, 0.9510565162951535312, 1.000000000000000000, 0.9510565162951535312, 1.000000000000000000, 0.9510565162951535312, 1.000000000000000000, 0.9510565162951535312, 1.000000000000000000, 0.9510565162951535312, 1.000000000000000000, 0.9510565162951535312, 1.000000000000000000, 0.9510565162951535312, 1.000000000000000000, 0.9510565162951535312, 1.000000000000000000, 0.9510565162951535312, 1.000000000000000000, 0.9510565162951535312, 1.000000000000000000, 0.9510565162951535312, 1.000000000000000000, 0.9510565162951535312, 1.000000000000000000, 0.9510565162951535312, 1.000000000000000000, 0.9510565162951535312, 1.000000000000000000, 0.9510565162951535312, 1.000000000000000000, 0.9510565162951535312, 1.000000000000000000, 0.9510565162951535312, 1.000000000000000000, 0.9510565162951535312, 1.000000000000000000, 0.9510565162951535312, 1.000000000000000000, 0.9510565162951535312, 1.000000000000000000, 0.9510565162951535312, 1.000000000000000000, 0.9510565162951535312, 1.000000000000000000, 0.9510565162951535312, 1.000000000000000000, 0.9510565162951535312, 1.000000000000000000, 0.9510565162951535312, 1.000000000000000000, 0.9510565162951535312, 1.000000000000000000, 0.9510565162951535312, 1.000000000000000000, 0.9510565162951535312, 1.000000000000000000, 0.9510565162951535312, 1.000000000000000000, 0.9510565162951535312, 1.000000000000000000, 0.9510565162951535312, 1.000000000000000000, 0.9510565162951535312, 1.000000000000000000, 0.9510565162951535312, 1.000000000000000000, 0.9510565162951535312, 1.000000000000000000, 0.9510565162951535312, 1.000000000000000000, 0.9510565162951535312, 1.000000000000000000, 0.9510565162951535312, 1.000000000000000000, 0.9510565162951535312, 1.000000000000000000, 0.9510565162951535312, 1.000000000000000000, 0.9510565162951535312, 1.000000000000000000, 0.9510565162951535312, 1.000000000000000000, 0.9510565162951535312, 1.000000000000000000, 0.9510565162951535312, 1.000000000000000000, 0.9510565162951535312, 1.000000000000000000, 0.9510565162951535312, 1.000000000000000000, 0.9510565162951535312, 1.000000000000000000, 0.9510565162951535312, 1.000000000000000000, 0.9510565162951535312, 1.000000000000000000, 0.9510565162951535312, 1.000000000000000000, 0.9510565162951535312, 1.000000000000000000, 0.9510565162951535312, 1.000000000000000000, 0.9510565162951535312, 1.000000000000000000, 0.9510565162951535312, 1.000000000000000000, 0.9510565162951535312, 1.000000000000000000, 0.9510565162951535312, 1.000000000000000000, 0.9510565162951535312, 1.000000000000000000, 0.9510565162951535312, 1.000000000000000000, 0.9510565162951535312, 1.000000000000000000, 0.9510565162951535312, 1.000000000000000000, 0.9510565162951535312, 1.000000000000000000, 0.9510565162951535312, 1.000000000000000000, 0.9510565162951535312, 1.000000000000000000, 0.9510565162951535312, 1.000000000000000000, 0.9510565162951535312, 1.000000000000000000, 0.9510565162951535312, 1.000000000000000000, 0.9510565162951535312, 1.000000000000000000, 0.9510565162951535312, 1.000000000000000000, 0.9510565162951535312, 1.000000000000000000, 0.9510565162951535312, 1.000000000000000000, 0.9510565162951535312, 1.000000000000000000, 0.9510565162951535312, 1.000000000000000000, 0.9510565162951535312, 1.000000000000000000, 0.9510565162951535312, 1.000000000000000000, 0.9510565162951535312, 1.000000000000000000, 0.9510565162951535312, 1.000000000000000000, 0.9510565162951535312, 1.000000000000000000, 0.9510565162951535312, 1.000000000000000000, 0.9510565162951535312, 1.000000000000000000, 0.9510565162951535312, 1.000000000000000000, 0.9510565162951535312, 1.000000000000000000, 0.9510565162951535312, 1.000000000000000000, 0.9510565162951535312, 1.000000000000000000, 0.9510565162951535312, 1.000000000000000000, 0.9510565162951535312, 1.000000000000000000, 0.9510565162951535312, 1.000000000000000000, 0.9510565162951535312, 1.000000000000000000, 0.9510565162951535312, 1.000000000000000000, 0.9510565162951535312, 1.000000000000000000, 0.9510565162951535312, 1.000000000000000000, 0.9510565162951535312, 1.000000000000000000, 0.9510565162951535312, 1.000000000000000000, 0.9510565162951535312, 1.000000000000000000, 0.9510565162951535312, 1.000000000000000000) ) ) 
 REPRESENTATION_ITEM ( '' )  SURFACE ( )  );
#9365=CARTESIAN_POINT ( 'NONE',  ( 45.86712807150323812, 65.29948385550241596, -5.649768623646098220 ) ) ;
#9366=CARTESIAN_POINT ( 'NONE',  ( 56.65037692655918988, 59.89948385550241028, -2.184720259617163762 ) ) ;
#9367=CARTESIAN_POINT ( 'NONE',  ( 45.90387839640208512, 62.30051614449766362, -5.676469297603124353 ) ) ;
#9371=CARTESIAN_POINT ( 'NONE',  ( 45.90387839640208512, 50.30051614449766362, -5.676469297603124353 ) ) ;
#9372=CARTESIAN_POINT ( 'NONE',  ( 50.02271294988511841, 50.49948385550239749, 6.000000000000000888 ) ) ;
#9385=CARTESIAN_POINT ( 'NONE',  ( 52.25172492374522903, 45.59948385550240602, -7.007379884777225953 ) ) ;
#9389=CARTESIAN_POINT ( 'NONE',  ( 48.07319477248762496, 48.40051614449766504, -6.007379884777208190 ) ) ;
#9394=CARTESIAN_POINT ( 'NONE',  ( 49.97728705011488159, 51.49948385550240459, -7.000000000000000888 ) ) ;
#9396=CARTESIAN_POINT ( 'NONE',  ( 50.02271294988512551, 52.49948385550240459, 7.000000000000000888 ) ) ;
#9403=CARTESIAN_POINT ( 'NONE',  ( 56.66441430157294690, 46.90051614449765793, -2.141517661632166281 ) ) ;
#9405=CARTESIAN_POINT ( 'NONE',  ( 52.57664461997811856, 63.59948385550239891, -8.007379884777229506 ) ) ;
#9407=CARTESIAN_POINT ( 'NONE',  ( 54.68390685589033495, 57.69948385550241454, -6.485486291978119766 ) ) ;
#9416=CARTESIAN_POINT ( 'NONE',  ( 50.02271294988506156, 46.50051614449766646, -6.000000000000000888 ) ) ;
#9418=CARTESIAN_POINT ( 'NONE',  ( 47.70284917648459810, 61.60051614449765367, 6.992620115222797139 ) ) ;
#9419=CARTESIAN_POINT ( 'NONE',  ( 50.02271294988513972, 46.49948385550240459, 8.000000000000001776 ) ) ;
#9421=CARTESIAN_POINT ( 'NONE',  ( 58.41169779390614281, 51.00051614449765935, 0.02388180880515032231 ) ) ;
#9429=CARTESIAN_POINT ( 'NONE',  ( 44.88205777487398507, 53.19948385550240744, -3.688883143319540814 ) ) ;
#9431=CARTESIAN_POINT ( 'NONE',  ( 45.90387839640208512, 60.30051614449766362, -5.676469297603124353 ) ) ;
#9434=CARTESIAN_POINT ( 'NONE',  ( 52.07576163693497051, 45.00000000000001421, -7.275735003127095979 ) ) ;
#9435=CARTESIAN_POINT ( 'NONE',  ( 54.13287192849671214, 52.70051614449766220, -5.649768623646139964 ) ) ;
#9436=CARTESIAN_POINT ( 'NONE',  ( 53.50833635130540955, 57.69948385550241454, -4.867452303228209765 ) ) ;
#9437=CARTESIAN_POINT ( 'NONE',  ( 55.32279841668061238, 44.85244137215321558, -4.999999999999997335 ) ) ;
#9448=CARTESIAN_POINT ( 'NONE',  ( 44.30067958973594955, 54.10051614449766078, -1.875703265242155693 ) ) ;
#9451=CARTESIAN_POINT ( 'NONE',  ( 49.97728705011488159, 63.49948385550241170, -7.000000000000000888 ) ) ;
#9452=CARTESIAN_POINT ( 'NONE',  ( 49.97728705011488159, 61.49948385550240459, -7.000000000000000888 ) ) ;
#9461=CARTESIAN_POINT ( 'NONE',  ( 45.86712807150329496, 49.70051614449766220, 5.649768623646139964 ) ) ;
#9464=CARTESIAN_POINT ( 'NONE',  ( 55.94051828345050836, 47.79948385550240886, -4.345558710429104465 ) ) ;
#9466=CARTESIAN_POINT ( 'NONE',  ( 56.79116909180255135, 57.79948385550240175, -4.963592699179005585 ) ) ;
#9468=VERTEX_POINT ( 'NONE', #874 ) ;
#9471=CARTESIAN_POINT ( 'NONE',  ( 54.42198456365324688, 44.83981687677464834, -4.999999999999773515 ) ) ;
#9476=CARTESIAN_POINT ( 'NONE',  ( 53.50833635130544508, 49.30051614449766362, 4.867452303228181343 ) ) ;
#9477=CARTESIAN_POINT ( 'NONE',  ( 47.74827507625470702, 58.40051614449766504, -7.007379884777204637 ) ) ;
#9479=CARTESIAN_POINT ( 'NONE',  ( 43.20883090819745576, 46.79948385550240886, 4.963592699179006473 ) ) ;
#9482=CARTESIAN_POINT ( 'NONE',  ( 54.68390685589039890, 59.30051614449766362, 6.485486291978072693 ) ) ;
#9493=CARTESIAN_POINT ( 'NONE',  ( 55.11794222512601493, 50.19948385550241454, 3.688883143319541702 ) ) ;
#9495=CARTESIAN_POINT ( 'NONE',  ( 47.74827507625477807, 62.59948385550239891, 7.007379884777229506 ) ) ;
#9496=CARTESIAN_POINT ( 'NONE',  ( 42.63976443033212860, 64.00051614449765225, -0.02388180880514948964 ) ) ;
#9501=CARTESIAN_POINT ( 'NONE',  ( 54.09612160359792199, 55.30051614449765651, 5.676469297603124353 ) ) ;
#9503=CARTESIAN_POINT ( 'NONE',  ( 44.30067958973596376, 56.89948385550240317, 1.875703265242204099 ) ) ;
#9513=CARTESIAN_POINT ( 'NONE',  ( 55.94051828345050836, 51.79948385550240175, -4.345558710429104465 ) ) ;
#9516=CARTESIAN_POINT ( 'NONE',  ( 50.02271294988506156, 54.50051614449765935, -6.000000000000000888 ) ) ;
#9520=CARTESIAN_POINT ( 'NONE',  ( 50.02271294988512551, 60.49948385550240459, 7.000000000000000888 ) ) ;
#9521=CARTESIAN_POINT ( 'NONE',  ( 50.02271294988512551, 60.49948385550240459, 7.000000000000000888 ) ) ;
#9530=CARTESIAN_POINT ( 'NONE',  ( 43.34962307344081012, 46.89948385550240317, 2.184720259617164650 ) ) ;
#9532=CARTESIAN_POINT ( 'NONE',  ( 44.03140696652198471, 49.80051614449766362, 4.306917132069485454 ) ) ;
#9535=CARTESIAN_POINT ( 'NONE',  ( 54.13287192849676188, 48.29948385550240175, 5.649768623646098220 ) ) ;
#9537=CARTESIAN_POINT ( 'NONE',  ( 54.68390685589033495, 59.69948385550240744, -6.485486291978119766 ) ) ;
#9547=CARTESIAN_POINT ( 'NONE',  ( 43.69122665457040000, 46.00051614449764514, -0.02388180880515696977 ) ) ;
#9548=CARTESIAN_POINT ( 'NONE',  ( 47.70284917648459810, 57.60051614449765367, 6.992620115222797139 ) ) ;
#9550=CARTESIAN_POINT ( 'NONE',  ( 50.02271294988505446, 62.50051614449767357, -8.000000000000001776 ) ) ;
#9552=CARTESIAN_POINT ( 'NONE',  ( 42.39856655714564226, 54.10051614449766078, -2.493737253992044156 ) ) ;
#9554=( BOUNDED_CURVE ( )  B_SPLINE_CURVE ( 2, ( #12571, #11469, #2968, #6239, #3102, #7399, #7334, #872, #6163, #3033, #1008, #10433, #8499, #1072, #9530, #10362, #2123, #11610, #8299, #6368, #11547, #13454, #5324, #5261, #12702, #4002, #58, #7195, #11398, #2060, #5123, #12499, #13661, #13526, #4210, #4279, #4073, #3242, #11665, #6099, #3760, #7665, #6563, #9015, #125, #4548, #6875, #12764, #12831, #3443, #4346, #6434, #10633, #11869, #13213, #10828, #5522, #2390, #187, #11084, #3307, #7734, #6631, #8562, #7529, #1345, #8768, #3374, #1600, #4477, #5592, #7983, #2190, #7598, #11803, #11736, #5846, #12962, #3509, #1275, #10763, #12898, #2325, #9736, #1147, #5397, #8700, #11939, #5463, #9802, #321, #2254, #9601, #2458, #253, #10044, #557, #6503, #10703, #1216, #4802, #9666, #4411, #8630, #11295, #3895, #622, #8123, #6063, #831, #1817, #7012, #8055, #9159, #7158, #13354, #908, #3002, #1956, #12262, #8263, #12327, #10190, #8194, #6199, #11153, #12466, #11367, #5161, #2723, #13490, #6945, #3831, #2862, #1671, #698, #6131, #1743, #12397, #4041, #2795, #13422, #10257, #4875, #9366, #3964, #7085, #13565, #10113, #5088, #7230, #9088, #768, #2935, #13287, #5914, #11222, #1888, #4111, #10327, #5020, #12195, #9226, #9296, #10396, #11430, #5988, #4948, #10462, #8530, #1179, #9495, #3339, #10601, #7494, #9698, #223, #18, #5292, #13627, #7563, #11638, #4243, #4311, #4175, #5360, #8462, #2155, #3066, #8335, #1108, #156, #11576, #11699, #9566, #8398, #1241, #12666, #4373, #10730, #6467 ),
 .UNSPECIFIED., .F., .F. ) 
 B_SPLINE_CURVE_WITH_KNOTS ( ( 3, 2, 2, 2, 2, 2, 2, 2, 2, 2, 2, 2, 2, 2, 2, 2, 2, 2, 2, 2, 2, 2, 2, 2, 2, 2, 2, 2, 2, 2, 2, 2, 2, 2, 2, 2, 2, 2, 2, 2, 2, 2, 2, 2, 2, 2, 2, 2, 2, 2, 2, 2, 2, 2, 2, 2, 2, 2, 2, 2, 2, 2, 2, 2, 2, 2, 2, 2, 2, 2, 2, 2, 2, 2, 2, 2, 2, 2, 2, 2, 2, 2, 2, 2, 2, 2, 2, 2, 2, 2, 2, 2, 2, 2, 2, 2, 2, 2, 2, 2, 3 ),
 ( 0.000000000000000000, 0.01000000000000000021, 0.02000000000000000042, 0.02999999999999999889, 0.04000000000000000083, 0.05000000000000000278, 0.05999999999999999778, 0.07000000000000000666, 0.08000000000000000167, 0.08999999999999999667, 0.1000000000000000056, 0.1100000000000000006, 0.1199999999999999956, 0.1300000000000000044, 0.1400000000000000133, 0.1499999999999999944, 0.1600000000000000033, 0.1700000000000000122, 0.1799999999999999933, 0.1900000000000000022, 0.2000000000000000111, 0.2099999999999999922, 0.2200000000000000011, 0.2300000000000000100, 0.2399999999999999911, 0.2500000000000000000, 0.2600000000000000089, 0.2700000000000000178, 0.2800000000000000266, 0.2899999999999999800, 0.2999999999999999889, 0.3099999999999999978, 0.3200000000000000067, 0.3300000000000000155, 0.3400000000000000244, 0.3499999999999999778, 0.3599999999999999867, 0.3699999999999999956, 0.3800000000000000044, 0.3900000000000000133, 0.4000000000000000222, 0.4099999999999999756, 0.4199999999999999845, 0.4299999999999999933, 0.4400000000000000022, 0.4500000000000000111, 0.4600000000000000200, 0.4699999999999999734, 0.4799999999999999822, 0.4899999999999999911, 0.5000000000000000000, 0.5100000000000000089, 0.5200000000000000178, 0.5300000000000000266, 0.5400000000000000355, 0.5500000000000000444, 0.5600000000000000533, 0.5699999999999999512, 0.5799999999999999600, 0.5899999999999999689, 0.5999999999999999778, 0.6099999999999999867, 0.6199999999999999956, 0.6300000000000000044, 0.6400000000000000133, 0.6500000000000000222, 0.6600000000000000311, 0.6700000000000000400, 0.6800000000000000488, 0.6899999999999999467, 0.6999999999999999556, 0.7099999999999999645, 0.7199999999999999734, 0.7299999999999999822, 0.7399999999999999911, 0.7500000000000000000, 0.7600000000000000089, 0.7700000000000000178, 0.7800000000000000266, 0.7900000000000000355, 0.8000000000000000444, 0.8100000000000000533, 0.8199999999999999512, 0.8299999999999999600, 0.8399999999999999689, 0.8499999999999999778, 0.8599999999999999867, 0.8699999999999999956, 0.8800000000000000044, 0.8900000000000000133, 0.9000000000000000222, 0.9100000000000000311, 0.9200000000000000400, 0.9300000000000000488, 0.9399999999999999467, 0.9499999999999999556, 0.9599999999999999645, 0.9699999999999999734, 0.9799999999999999822, 0.9899999999999999911, 1.000000000000000000 ),
 .UNSPECIFIED. ) 
 CURVE ( )  GEOMETRIC_REPRESENTATION_ITEM ( )  RATIONAL_B_SPLINE_CURVE ( ( 1.000000000000000000, 0.9510565162951535312, 1.000000000000000000, 0.9510565162951535312, 1.000000000000000000, 0.9510565162951535312, 1.000000000000000000, 0.9510565162951535312, 1.000000000000000000, 0.9510565162951535312, 1.000000000000000000, 0.9510565162951535312, 1.000000000000000000, 0.9510565162951535312, 1.000000000000000000, 0.9510565162951535312, 1.000000000000000000, 0.9510565162951535312, 1.000000000000000000, 0.9510565162951535312, 1.000000000000000000, 0.9510565162951535312, 1.000000000000000000, 0.9510565162951535312, 1.000000000000000000, 0.9510565162951535312, 1.000000000000000000, 0.9510565162951535312, 1.000000000000000000, 0.9510565162951535312, 1.000000000000000000, 0.9510565162951535312, 1.000000000000000000, 0.9510565162951535312, 1.000000000000000000, 0.9510565162951535312, 1.000000000000000000, 0.9510565162951535312, 1.000000000000000000, 0.9510565162951535312, 1.000000000000000000, 0.9510565162951535312, 1.000000000000000000, 0.9510565162951535312, 1.000000000000000000, 0.9510565162951535312, 1.000000000000000000, 0.9510565162951535312, 1.000000000000000000, 0.9510565162951535312, 1.000000000000000000, 0.9510565162951535312, 1.000000000000000000, 0.9510565162951535312, 1.000000000000000000, 0.9510565162951535312, 1.000000000000000000, 0.9510565162951535312, 1.000000000000000000, 0.9510565162951535312, 1.000000000000000000, 0.9510565162951535312, 1.000000000000000000, 0.9510565162951535312, 1.000000000000000000, 0.9510565162951535312, 1.000000000000000000, 0.9510565162951535312, 1.000000000000000000, 0.9510565162951535312, 1.000000000000000000, 0.9510565162951535312, 1.000000000000000000, 0.9510565162951535312, 1.000000000000000000, 0.9510565162951535312, 1.000000000000000000, 0.9510565162951535312, 1.000000000000000000, 0.9510565162951535312, 1.000000000000000000, 0.9510565162951535312, 1.000000000000000000, 0.9510565162951535312, 1.000000000000000000, 0.9510565162951535312, 1.000000000000000000, 0.9510565162951535312, 1.000000000000000000, 0.9510565162951535312, 1.000000000000000000, 0.9510565162951535312, 1.000000000000000000, 0.9510565162951535312, 1.000000000000000000, 0.9510565162951535312, 1.000000000000000000, 0.9510565162951535312, 1.000000000000000000, 0.9510565162951535312, 1.000000000000000000, 0.9510565162951535312, 1.000000000000000000, 0.9510565162951535312, 1.000000000000000000, 0.9510565162951535312, 1.000000000000000000, 0.9510565162951535312, 1.000000000000000000, 0.9510565162951535312, 1.000000000000000000, 0.9510565162951535312, 1.000000000000000000, 0.9510565162951535312, 1.000000000000000000, 0.9510565162951535312, 1.000000000000000000, 0.9510565162951535312, 1.000000000000000000, 0.9510565162951535312, 1.000000000000000000, 0.9510565162951535312, 1.000000000000000000, 0.9510565162951535312, 1.000000000000000000, 0.9510565162951535312, 1.000000000000000000, 0.9510565162951535312, 1.000000000000000000, 0.9510565162951535312, 1.000000000000000000, 0.9510565162951535312, 1.000000000000000000, 0.9510565162951535312, 1.000000000000000000, 0.9510565162951535312, 1.000000000000000000, 0.9510565162951535312, 1.000000000000000000, 0.9510565162951535312, 1.000000000000000000, 0.9510565162951535312, 1.000000000000000000, 0.9510565162951535312, 1.000000000000000000, 0.9510565162951535312, 1.000000000000000000, 0.9510565162951535312, 1.000000000000000000, 0.9510565162951535312, 1.000000000000000000, 0.9510565162951535312, 1.000000000000000000, 0.9510565162951535312, 1.000000000000000000, 0.9510565162951535312, 1.000000000000000000, 0.9510565162951535312, 1.000000000000000000, 0.9510565162951535312, 1.000000000000000000, 0.9510565162951535312, 1.000000000000000000, 0.9510565162951535312, 1.000000000000000000, 0.9510565162951535312, 1.000000000000000000, 0.9510565162951535312, 1.000000000000000000, 0.9510565162951535312, 1.000000000000000000, 0.9510565162951535312, 1.000000000000000000, 0.9510565162951535312, 1.000000000000000000, 0.9510565162951535312, 1.000000000000000000, 0.9510565162951535312, 1.000000000000000000, 0.9510565162951535312, 1.000000000000000000, 0.9510565162951535312, 1.000000000000000000, 0.9510565162951535312, 1.000000000000000000, 0.9510565162951535312, 1.000000000000000000, 0.9510565162951535312, 1.000000000000000000, 0.9510565162951535312, 1.000000000000000000, 0.9510565162951535312, 1.000000000000000000, 0.9510565162951535312, 1.000000000000000000, 0.9510565162951535312, 1.000000000000000000, 0.9510565162951535312, 1.000000000000000000, 0.9510565162951535312, 1.000000000000000000 ) ) 
 REPRESENTATION_ITEM ( '' )  );
#9565=CARTESIAN_POINT ( 'NONE',  ( 53.54508667620428497, 48.29948385550240175, 4.840751629271157874 ) ) ;
#9566=CARTESIAN_POINT ( 'NONE',  ( 43.34962307344081012, 64.89948385550239607, 2.184720259617164650 ) ) ;
#9567=CARTESIAN_POINT ( 'NONE',  ( 50.02271294988505446, 48.50051614449765935, -8.000000000000001776 ) ) ;
#9571=CARTESIAN_POINT ( 'NONE',  ( 55.94051828345053679, 57.20051614449766930, 4.345558710429044069 ) ) ;
#9572=CARTESIAN_POINT ( 'NONE',  ( 49.97728705011488870, 57.49948385550241170, -6.000000000000000888 ) ) ;
#9583=CARTESIAN_POINT ( 'NONE',  ( 52.25172492374522903, 51.59948385550240602, -7.007379884777225953 ) ) ;
#9586=CARTESIAN_POINT ( 'NONE',  ( 46.49166364869456913, 50.30051614449766362, -4.867452303228181343 ) ) ;
#9589=CARTESIAN_POINT ( 'NONE',  ( 45.86712807150323812, 63.29948385550240886, -5.649768623646098220 ) ) ;
#9591=CARTESIAN_POINT ( 'NONE',  ( 47.74827507625478518, 58.59948385550238470, 7.007379884777227730 ) ) ;
#9601=CARTESIAN_POINT ( 'NONE',  ( 45.90387839640214196, 54.69948385550240744, 5.676469297603166098 ) ) ;
#9603=CARTESIAN_POINT ( 'NONE',  ( 56.65037692655921120, 47.10051614449766078, 2.184720259617097593 ) ) ;
#9606=CARTESIAN_POINT ( 'NONE',  ( 49.97728705011488159, 45.49948385550240459, -7.000000000000000888 ) ) ;
#9609=CARTESIAN_POINT ( 'NONE',  ( 58.41169779390614281, 53.99948385550241170, -0.02388180880523160798 ) ) ;
#9615=CARTESIAN_POINT ( 'NONE',  ( 51.92680522751238925, 45.40051614449765793, 6.007379884777208190 ) ) ;
#9616=CARTESIAN_POINT ( 'NONE',  ( 57.36023556966787851, 57.00051614449766646, 0.02388180880515038476 ) ) ;
#9617=CARTESIAN_POINT ( 'NONE',  ( 57.60143344285433642, 47.89948385550240317, -2.493737253992118319 ) ) ;
#9619=CARTESIAN_POINT ( 'NONE',  ( 45.31609314410960820, 56.30051614449766362, -6.485486291978072693 ) ) ;
#9630=CARTESIAN_POINT ( 'NONE',  ( 46.45491332379572924, 49.29948385550240886, -4.840751629271157874 ) ) ;
#9632=CARTESIAN_POINT ( 'NONE',  ( 57.61547081786810764, 46.90051614449766504, -2.450534656007114176 ) ) ;
#9637=CARTESIAN_POINT ( 'NONE',  ( 50.02271294988505446, 60.50051614449765935, -7.000000000000000888 ) ) ;
#9638=CARTESIAN_POINT ( 'NONE',  ( 48.07319477248768180, 60.59948385550240602, 6.007379884777225953 ) ) ;
#9646=CARTESIAN_POINT ( 'NONE',  ( 52.29715082351547295, 48.39948385550240317, 6.992620115222774047 ) ) ;
#9648=CARTESIAN_POINT ( 'NONE',  ( 55.71335778527780036, 48.90051614449766504, -1.832500667257213056 ) ) ;
#9653=CARTESIAN_POINT ( 'NONE',  ( 56.65037692655918988, 59.89948385550241028, -2.184720259617163762 ) ) ;
#9666=CARTESIAN_POINT ( 'NONE',  ( 52.25172492374522903, 55.59948385550241312, -7.007379884777227730 ) ) ;
#9667=CARTESIAN_POINT ( 'NONE',  ( 44.05948171654945611, 56.20051614449764799, -4.345558710429044069 ) ) ;
#9669=CARTESIAN_POINT ( 'NONE',  ( 43.18075615816989199, 63.19948385550240744, -4.924951120819313743 ) ) ;
#9671=CARTESIAN_POINT ( 'NONE',  ( 45.31609314410967926, 56.69948385550240744, 6.485486291978119766 ) ) ;
#9678=CARTESIAN_POINT ( 'NONE',  ( 46.49166364869456913, 46.30051614449766362, -4.867452303228181343 ) ) ;
#9680=CARTESIAN_POINT ( 'NONE',  ( 42.39856655714566358, 48.89948385550241028, 2.493737253992119207 ) ) ;
#9682=CARTESIAN_POINT ( 'NONE',  ( 52.62207051974829852, 54.60051614449766788, -7.992620115222797139 ) ) ;
#9696=CARTESIAN_POINT ( 'NONE',  ( 51.97223112728254790, 52.39948385550241028, 5.992620115222778487 ) ) ;
#9698=CARTESIAN_POINT ( 'NONE',  ( 42.63976443033212149, 62.99948385550241170, 0.02388180880522514787 ) ) ;
#9699=CARTESIAN_POINT ( 'NONE',  ( 41.58830220609386430, 46.00051614449764514, -0.02388180880514929535 ) ) ;
#9703=CARTESIAN_POINT ( 'NONE',  ( 47.74827507625469281, 60.40051614449767214, -7.007379884777203749 ) ) ;
#9704=CARTESIAN_POINT ( 'NONE',  ( 55.08986747509847248, 57.79948385550240175, -3.727524721679197572 ) ) ;
#9705=VERTEX_POINT ( 'NONE', #12834 ) ;
#9714=CARTESIAN_POINT ( 'NONE',  ( 54.09612160359786515, 49.69948385550240744, -5.676469297603166098 ) ) ;
#9718=CARTESIAN_POINT ( 'NONE',  ( 49.97728705011494554, 59.50051614449765935, 6.000000000000000888 ) ) ;
#9723=CARTESIAN_POINT ( 'NONE',  ( 56.66441430157296821, 62.09948385550239891, 2.141517661632100111 ) ) ;
#9726=VERTEX_POINT ( 'NONE', #3377 ) ;
#9736=CARTESIAN_POINT ( 'NONE',  ( 55.94051828345050836, 53.79948385550240175, -4.345558710429103577 ) ) ;
#9737=CARTESIAN_POINT ( 'NONE',  ( 44.03140696652198471, 51.80051614449766362, 4.306917132069485454 ) ) ;
#9740=CARTESIAN_POINT ( 'NONE',  ( 49.97728705011488159, 49.49948385550240459, -7.000000000000000888 ) ) ;
#9743=CARTESIAN_POINT ( 'NONE',  ( 56.79116909180255135, 59.79948385550240175, -4.963592699179005585 ) ) ;
#9749=CARTESIAN_POINT ( 'NONE',  ( 55.11794222512599362, 54.80051614449764941, -3.688883143319583446 ) ) ;
#9751=CARTESIAN_POINT ( 'NONE',  ( 43.20883090819745576, 50.79948385550240175, 4.963592699179006473 ) ) ;
#9752=CARTESIAN_POINT ( 'NONE',  ( 54.09612160359786515, 55.69948385550240744, -5.676469297603166098 ) ) ;
#9754=CARTESIAN_POINT ( 'NONE',  ( 45.31609314410960820, 58.30051614449765651, -6.485486291978072693 ) ) ;
#9766=CARTESIAN_POINT ( 'NONE',  ( 51.92680522751233951, 59.59948385550240602, -6.007379884777223289 ) ) ;
#9767=CARTESIAN_POINT ( 'NONE',  ( 45.86712807150329496, 45.70051614449766220, 5.649768623646139964 ) ) ;
#9768=CARTESIAN_POINT ( 'NONE',  ( 58.41169779390614281, 45.00051614449765225, 0.02388180880515032231 ) ) ;
#9771=CARTESIAN_POINT ( 'NONE',  ( 43.34962307344078880, 58.10051614449766078, -2.184720259617096705 ) ) ;
#9772=CARTESIAN_POINT ( 'NONE',  ( 44.30067958973596376, 62.89948385550240317, 1.875703265242204099 ) ) ;
#9781=CARTESIAN_POINT ( 'NONE',  ( 42.63976443033212860, 54.99948385550241170, 0.02388180880522514787 ) ) ;
#9784=CARTESIAN_POINT ( 'NONE',  ( 44.28664221472221385, 57.90051614449765793, 1.832500667257213722 ) ) ;
#9788=CARTESIAN_POINT ( 'NONE',  ( 54.13287192849676188, 64.29948385550241596, 5.649768623646098220 ) ) ;
#9802=CARTESIAN_POINT ( 'NONE',  ( 52.29715082351547295, 54.39948385550239607, 6.992620115222774047 ) ) ;
#9803=CARTESIAN_POINT ( 'NONE',  ( 50.02271294988505446, 52.50051614449765935, -7.000000000000000888 ) ) ;
#9805=CARTESIAN_POINT ( 'NONE',  ( 47.74827507625478518, 54.59948385550239180, 7.007379884777227730 ) ) ;
#9806=CARTESIAN_POINT ( 'NONE',  ( 45.27934281921075410, 61.29948385550240886, -6.458785618021043895 ) ) ;
#9816=CARTESIAN_POINT ( 'NONE',  ( 55.71335778527780036, 52.90051614449766504, -1.832500667257213056 ) ) ;
#9817=CARTESIAN_POINT ( 'NONE',  ( 44.03140696652198471, 63.80051614449764941, 4.306917132069485454 ) ) ;
#9819=CARTESIAN_POINT ( 'NONE',  ( 52.62207051974839089, 54.39948385550241028, 7.992620115222770494 ) ) ;
#9820=CARTESIAN_POINT ( 'NONE',  ( 54.13287192849676188, 58.29948385550240175, 5.649768623646098220 ) ) ;
#9823=CARTESIAN_POINT ( 'NONE',  ( 57.60143344285435774, 63.10051614449766078, 2.493737253992045044 ) ) ;
#9834=CARTESIAN_POINT ( 'NONE',  ( 49.97728705011488870, 59.49948385550240459, -6.000000000000000888 ) ) ;
#9835=CARTESIAN_POINT ( 'NONE',  ( 57.36023556966787851, 49.00051614449764514, 0.02388180880515038476 ) ) ;
#9836=CARTESIAN_POINT ( 'NONE',  ( 42.38452918213190657, 51.90051614449765793, 2.450534656007115508 ) ) ;
#9839=CARTESIAN_POINT ( 'NONE',  ( 44.03140696652198471, 61.80051614449767072, 4.306917132069485454 ) ) ;
#9848=CARTESIAN_POINT ( 'NONE',  ( 44.03140696652192787, 59.19948385550238612, -4.306917132069425058 ) ) ;
#9851=CARTESIAN_POINT ( 'NONE',  ( 56.30877334542961421, 57.00051614449766646, 0.02388180880515774693 ) ) ;
#9854=CARTESIAN_POINT ( 'NONE',  ( 49.97728705011488870, 45.49948385550240459, -6.000000000000000888 ) ) ;
#9865=CARTESIAN_POINT ( 'NONE',  ( 56.66441430157294690, 52.90051614449765793, -2.141517661632166281 ) ) ;
#9867=CARTESIAN_POINT ( 'NONE',  ( 43.33558569842703179, 53.09948385550240602, -2.141517661632099223 ) ) ;
#9869=CARTESIAN_POINT ( 'NONE',  ( 42.38452918213188525, 63.09948385550240602, -2.450534656007040013 ) ) ;
#9871=ORIENTED_EDGE ( 'NONE', *, *, #9017, .T. ) ;
#9876=CARTESIAN_POINT ( 'NONE',  ( 51.92680522751238925, 53.40051614449765793, 6.007379884777208190 ) ) ;
#9878=CARTESIAN_POINT ( 'NONE',  ( 57.61547081786812896, 56.09948385550240602, 2.450534656007040901 ) ) ;
#9879=CARTESIAN_POINT ( 'NONE',  ( 47.70284917648453415, 55.39948385550238896, -6.992620115222774047 ) ) ;
#9882=CARTESIAN_POINT ( 'NONE',  ( 52.62207051974829852, 60.60051614449765367, -7.992620115222797139 ) ) ;
#9893=CARTESIAN_POINT ( 'NONE',  ( 55.71335778527780747, 56.09948385550240602, 1.832500667257165983 ) ) ;
#9894=CARTESIAN_POINT ( 'NONE',  ( 54.09612160359792199, 45.30051614449766362, 5.676469297603124353 ) ) ;
#9896=CARTESIAN_POINT ( 'NONE',  ( 57.60143344285435774, 53.10051614449767499, 2.493737253992045044 ) ) ;
#9901=CARTESIAN_POINT ( 'NONE',  ( 56.65037692655921120, 63.10051614449766078, 2.184720259617097593 ) ) ;
#9910=CARTESIAN_POINT ( 'NONE',  ( 52.29715082351547295, 56.39948385550238896, 6.992620115222774047 ) ) ;
#9912=CARTESIAN_POINT ( 'NONE',  ( 53.50833635130544508, 59.30051614449766362, 4.867452303228181343 ) ) ;
#9915=CARTESIAN_POINT ( 'NONE',  ( 44.91013252490150620, 62.20051614449766220, -3.727524721679154940 ) ) ;
#9916=CARTESIAN_POINT ( 'NONE',  ( 52.25172492374522903, 63.59948385550237759, -7.007379884777225953 ) ) ;
#9929=CARTESIAN_POINT ( 'NONE',  ( 49.97728705011495265, 51.50051614449765935, 7.000000000000000888 ) ) ;
#9932=CARTESIAN_POINT ( 'NONE',  ( 55.96859303347804371, 52.19948385550240033, 4.306917132069425946 ) ) ;
#9933=CARTESIAN_POINT ( 'NONE',  ( 52.25172492374522903, 45.59948385550240602, -7.007379884777225953 ) ) ;
#9934=CARTESIAN_POINT ( 'NONE',  ( 56.65037692655918988, 45.89948385550240317, -2.184720259617163762 ) ) ;
#9943=CARTESIAN_POINT ( 'NONE',  ( 46.49166364869456913, 56.30051614449766362, -4.867452303228181343 ) ) ;
#9946=CARTESIAN_POINT ( 'NONE',  ( 52.57664461997811856, 55.59948385550240602, -8.007379884777229506 ) ) ;
#9947=CARTESIAN_POINT ( 'NONE',  ( 56.65037692655918988, 57.89948385550240317, -2.184720259617163762 ) ) ;
#9949=CARTESIAN_POINT ( 'NONE',  ( 54.68390685589039890, 63.30051614449767072, 6.485486291978072693 ) ) ;
#9956=VERTEX_POINT ( 'NONE', #3158 ) ;
#9961=CARTESIAN_POINT ( 'NONE',  ( 48.02776887271745210, 53.39948385550241028, -5.992620115222778487 ) ) ;
#9963=CARTESIAN_POINT ( 'NONE',  ( 56.79116909180259398, 51.20051614449766220, 4.963592699178938972 ) ) ;
#9968=CARTESIAN_POINT ( 'NONE',  ( 47.70284917648459100, 61.60051614449764656, 6.992620115222796251 ) ) ;
#9976=CARTESIAN_POINT ( 'NONE',  ( 52.25172492374522903, 55.59948385550241312, -7.007379884777225953 ) ) ;
#9977=CARTESIAN_POINT ( 'NONE',  ( 51.97223112728249816, 56.60051614449765367, -5.992620115222793586 ) ) ;
#9980=CARTESIAN_POINT ( 'NONE',  ( 46.45491332379576477, 61.70051614449766220, 4.840751629271188961 ) ) ;
#9981=CARTESIAN_POINT ( 'NONE',  ( 46.45491332379572924, 49.29948385550240886, -4.840751629271157874 ) ) ;
#9996=CARTESIAN_POINT ( 'NONE',  ( 44.03140696652198471, 59.80051614449766362, 4.306917132069485454 ) ) ;
#9999=CARTESIAN_POINT ( 'NONE',  ( 44.03140696652192787, 51.19948385550238612, -4.306917132069425058 ) ) ;
#10000=CARTESIAN_POINT ( 'NONE',  ( 45.86712807150323812, 47.29948385550240886, -5.649768623646098220 ) ) ;
#10001=CARTESIAN_POINT ( 'NONE',  ( 49.97728705011486738, 63.49948385550241170, -8.000000000000001776 ) ) ;
#10010=CARTESIAN_POINT ( 'NONE',  ( 44.88205777487401349, 59.80051614449766362, 3.688883143319584779 ) ) ;
#10012=CARTESIAN_POINT ( 'NONE',  ( 47.42335538002188144, 54.59948385550240602, 8.007379884777233059 ) ) ;
#10014=CARTESIAN_POINT ( 'NONE',  ( 54.09612160359786515, 59.69948385550240033, -5.676469297603166098 ) ) ;
#10017=CARTESIAN_POINT ( 'NONE',  ( 45.27934281921082516, 61.70051614449766220, 6.458785618021089192 ) ) ;
#10029=CARTESIAN_POINT ( 'NONE',  ( 46.45491332379572924, 59.29948385550240886, -4.840751629271157874 ) ) ;
#10030=CARTESIAN_POINT ( 'NONE',  ( 56.65037692655921120, 49.10051614449766078, 2.184720259617097593 ) ) ;
#10032=CARTESIAN_POINT ( 'NONE',  ( 45.31609314410960820, 52.30051614449766362, -6.485486291978072693 ) ) ;
#10035=CARTESIAN_POINT ( 'NONE',  ( 57.36023556966787851, 63.00051614449767357, 0.02388180880515038476 ) ) ;
#10037=ORIENTED_EDGE ( 'NONE', *, *, #1753, .T. ) ;
#10043=CARTESIAN_POINT ( 'NONE',  ( 44.03140696652192787, 55.19948385550238612, -4.306917132069425058 ) ) ;
#10044=CARTESIAN_POINT ( 'NONE',  ( 42.63976443033212149, 54.99948385550239749, 0.02388180880522514787 ) ) ;
#10048=CARTESIAN_POINT ( 'NONE',  ( 45.86712807150329496, 45.70051614449766220, 5.649768623646139964 ) ) ;
#10049=CARTESIAN_POINT ( 'NONE',  ( 43.69122665457040000, 48.99948385550241170, 0.02388180880521036456 ) ) ;
#10061=CARTESIAN_POINT ( 'NONE',  ( 52.25172492374527877, 59.40051614449765083, 7.007379884777203749 ) ) ;
#10065=CARTESIAN_POINT ( 'NONE',  ( 54.13287192849676188, 60.29948385550240886, 5.649768623646098220 ) ) ;
#10067=CARTESIAN_POINT ( 'NONE',  ( 43.33558569842703179, 49.09948385550240602, -2.141517661632099223 ) ) ;
#10070=CARTESIAN_POINT ( 'NONE',  ( 57.36023556966787851, 51.99948385550238328, -0.02388180880522424582 ) ) ;
#10079=CARTESIAN_POINT ( 'NONE',  ( 53.54508667620424234, 60.70051614449766930, -4.840751629271188961 ) ) ;
#10082=CARTESIAN_POINT ( 'NONE',  ( 52.62207051974839089, 62.39948385550240317, 7.992620115222770494 ) ) ;
#10084=CARTESIAN_POINT ( 'NONE',  ( 55.96859303347804371, 62.19948385550240744, 4.306917132069425946 ) ) ;
#10086=CARTESIAN_POINT ( 'NONE',  ( 58.41169779390614281, 45.99948385550240459, -0.02388180880523160798 ) ) ;
#10096=CARTESIAN_POINT ( 'NONE',  ( 51.92680522751233951, 61.59948385550240602, -6.007379884777223289 ) ) ;
#10097=CARTESIAN_POINT ( 'NONE',  ( 43.33558569842706021, 53.90051614449765793, 2.141517661632167169 ) ) ;
#10098=CARTESIAN_POINT ( 'NONE',  ( 58.41169779390614281, 55.00051614449766646, 0.02388180880515032231 ) ) ;
#10101=CARTESIAN_POINT ( 'NONE',  ( 53.61415392313774220, 44.99999999999997868, -5.449226822604907206 ) ) ;
#10102=CARTESIAN_POINT ( 'NONE',  ( 56.81924384183006538, 46.80051614449766362, -4.924951120819380357 ) ) ;
#10111=CARTESIAN_POINT ( 'NONE',  ( 42.63976443033212860, 64.99948385550240459, 0.02388180880522514787 ) ) ;
#10113=CARTESIAN_POINT ( 'NONE',  ( 54.13287192849676188, 60.29948385550240886, 5.649768623646098220 ) ) ;
#10117=CARTESIAN_POINT ( 'NONE',  ( 56.30877334542961421, 63.00051614449766646, 0.02388180880515774693 ) ) ;
#10118=CARTESIAN_POINT ( 'NONE',  ( 53.54508667620428497, 52.29948385550240886, 4.840751629271157874 ) ) ;
#10133=CARTESIAN_POINT ( 'NONE',  ( 55.94051828345053679, 59.20051614449766220, 4.345558710429044069 ) ) ;
#10136=CARTESIAN_POINT ( 'NONE',  ( 51.97223112728249816, 48.60051614449766788, -5.992620115222793586 ) ) ;
#10138=CARTESIAN_POINT ( 'NONE',  ( 45.86712807150323812, 59.29948385550240175, -5.649768623646098220 ) ) ;
#10139=CARTESIAN_POINT ( 'NONE',  ( 43.33558569842703179, 53.09948385550240602, -2.141517661632099223 ) ) ;
#10140=CARTESIAN_POINT ( 'NONE',  ( 52.25172492374522903, 49.59948385550240602, -7.007379884777225953 ) ) ;
#10152=CARTESIAN_POINT ( 'NONE',  ( 55.11794222512599362, 58.80051614449766362, -3.688883143319583446 ) ) ;
#10154=CARTESIAN_POINT ( 'NONE',  ( 42.38452918213188525, 57.09948385550240602, -2.450534656007040013 ) ) ;
#10156=CARTESIAN_POINT ( 'NONE',  ( 54.13287192849676188, 60.29948385550240886, 5.649768623646098220 ) ) ;
#10158=CARTESIAN_POINT ( 'NONE',  ( 57.61547081786812896, 50.09948385550240602, 2.450534656007040901 ) ) ;
#10174=CARTESIAN_POINT ( 'NONE',  ( 55.08986747509847248, 59.79948385550240175, -3.727524721679197572 ) ) ;
#10175=CARTESIAN_POINT ( 'NONE',  ( 54.09612160359792199, 53.30051614449766362, 5.676469297603124353 ) ) ;
#10176=CARTESIAN_POINT ( 'NONE',  ( 52.57664461997821093, 59.40051614449765793, 8.007379884777206414 ) ) ;
#10179=CARTESIAN_POINT ( 'NONE',  ( 52.57664461997821093, 49.40051614449766504, 8.007379884777206414 ) ) ;
#10189=CARTESIAN_POINT ( 'NONE',  ( 56.66441430157296821, 64.09948385550239891, 2.141517661632100111 ) ) ;
#10190=CARTESIAN_POINT ( 'NONE',  ( 54.09612160359786515, 57.69948385550240744, -5.676469297603166098 ) ) ;
#10194=CARTESIAN_POINT ( 'NONE',  ( 55.94051828345053679, 53.20051614449766220, 4.345558710429044069 ) ) ;
#10195=CARTESIAN_POINT ( 'NONE',  ( 48.02776887271745210, 53.39948385550241028, -5.992620115222778487 ) ) ;
#10208=CARTESIAN_POINT ( 'NONE',  ( 43.69122665457040000, 64.99948385550240459, 0.02388180880521036456 ) ) ;
#10210=CARTESIAN_POINT ( 'NONE',  ( 43.34962307344081012, 56.89948385550240317, 2.184720259617164650 ) ) ;
#10211=CARTESIAN_POINT ( 'NONE',  ( 52.29715082351547295, 50.39948385550240317, 6.992620115222774047 ) ) ;
#10215=CARTESIAN_POINT ( 'NONE',  ( 50.02271294988512551, 46.49948385550240459, 7.000000000000000888 ) ) ;
#10223=CARTESIAN_POINT ( 'NONE',  ( 48.07319477248762496, 60.40051614449765793, -6.007379884777208190 ) ) ;
#10224=CARTESIAN_POINT ( 'NONE',  ( 41.58830220609386430, 56.99948385550241170, 0.02388180880523263147 ) ) ;
#10225=CARTESIAN_POINT ( 'NONE',  ( 52.29715082351547295, 62.39948385550239607, 6.992620115222774047 ) ) ;
#10226=FACE_OUTER_BOUND ( 'NONE', #5154, .T. ) ;
#10227=CARTESIAN_POINT ( 'NONE',  ( 41.58830220609386430, 48.99948385550241170, 0.02388180880523263147 ) ) ;
#10237=CARTESIAN_POINT ( 'NONE',  ( 55.71335778527780747, 64.09948385550239891, 1.832500667257165983 ) ) ;
#10238=CARTESIAN_POINT ( 'NONE',  ( 43.34962307344078880, 52.10051614449766078, -2.184720259617096705 ) ) ;
#10240=CARTESIAN_POINT ( 'NONE',  ( 57.61547081786810764, 58.90051614449766504, -2.450534656007114176 ) ) ;
#10243=CARTESIAN_POINT ( 'NONE',  ( 41.58830220609386430, 52.00051614449766646, -0.02388180880514929535 ) ) ;
#10256=CARTESIAN_POINT ( 'NONE',  ( 46.49166364869460466, 46.69948385550240744, 4.867452303228209765 ) ) ;
#10257=CARTESIAN_POINT ( 'NONE',  ( 54.09612160359786515, 59.69948385550240033, -5.676469297603166098 ) ) ;
#10265=CARTESIAN_POINT ( 'NONE',  ( 56.66441430157294690, 48.90051614449766504, -2.141517661632166281 ) ) ;
#10266=CARTESIAN_POINT ( 'NONE',  ( 46.49166364869460466, 54.69948385550240033, 4.867452303228209765 ) ) ;
#10276=CARTESIAN_POINT ( 'NONE',  ( 47.70284917648453415, 47.39948385550238896, -6.992620115222774047 ) ) ;
#10279=CARTESIAN_POINT ( 'NONE',  ( 55.11794222512599362, 44.80051614449766362, -3.688883143319583446 ) ) ;
#10281=CARTESIAN_POINT ( 'NONE',  ( 45.86712807150323812, 55.29948385550240175, -5.649768623646098220 ) ) ;
#10282=CARTESIAN_POINT ( 'NONE',  ( 43.33558569842703179, 55.09948385550241312, -2.141517661632099223 ) ) ;
#10284=CARTESIAN_POINT ( 'NONE',  ( 42.63976443033212860, 50.99948385550240459, 0.02388180880522514787 ) ) ;
#10292=CARTESIAN_POINT ( 'NONE',  ( 50.02271294988506156, 58.50051614449765225, -6.000000000000000888 ) ) ;
#10295=CARTESIAN_POINT ( 'NONE',  ( 56.79116909180255135, 59.79948385550240175, -4.963592699179005585 ) ) ;
#10296=CARTESIAN_POINT ( 'NONE',  ( 50.02271294988512551, 62.49948385550240459, 7.000000000000000888 ) ) ;
#10298=CARTESIAN_POINT ( 'NONE',  ( 49.97728705011486738, 49.49948385550241170, -8.000000000000001776 ) ) ;
#10303=VECTOR ( 'NONE', #11347, 1000.000000000000000 ) ;
#10306=DIRECTION ( 'NONE',  ( -0.04542589977017699732, 0.9989677110047501252, 0.000000000000000000 ) ) ;
#10308=CARTESIAN_POINT ( 'NONE',  ( 55.11794222512601493, 64.19948385550240744, 3.688883143319541702 ) ) ;
#10309=CARTESIAN_POINT ( 'NONE',  ( 52.29715082351539479, 54.60051614449766788, -6.992620115222796251 ) ) ;
#10311=CARTESIAN_POINT ( 'NONE',  ( 45.31609314410960820, 58.30051614449765651, -6.485486291978072693 ) ) ;
#10313=CARTESIAN_POINT ( 'NONE',  ( 57.60143344285435774, 49.10051614449766788, 2.493737253992045044 ) ) ;
#10326=CARTESIAN_POINT ( 'NONE',  ( 44.05948171654949874, 62.79948385550241596, 4.345558710429105354 ) ) ;
#10327=CARTESIAN_POINT ( 'NONE',  ( 47.70284917648453415, 61.39948385550241028, -6.992620115222774047 ) ) ;
#10331=CARTESIAN_POINT ( 'NONE',  ( 52.29715082351538769, 50.60051614449766788, -6.992620115222796251 ) ) ;
#10332=CARTESIAN_POINT ( 'NONE',  ( 53.50833635130540955, 55.69948385550240744, -4.867452303228209765 ) ) ;
#10343=CARTESIAN_POINT ( 'NONE',  ( 52.29715082351547295, 46.39948385550240317, 6.992620115222774047 ) ) ;
#10346=CARTESIAN_POINT ( 'NONE',  ( 55.08986747509849380, 47.20051614449766220, 3.727524721679155384 ) ) ;
#10348=CARTESIAN_POINT ( 'NONE',  ( 44.03140696652192787, 57.19948385550238612, -4.306917132069425058 ) ) ;
#10349=CARTESIAN_POINT ( 'NONE',  ( 56.66441430157296821, 56.09948385550240602, 2.141517661632100111 ) ) ;
#10352=CARTESIAN_POINT ( 'NONE',  ( 47.70284917648453415, 49.39948385550238896, -6.992620115222774047 ) ) ;
#10362=CARTESIAN_POINT ( 'NONE',  ( 42.63976443033212149, 46.99948385550240459, 0.02388180880522514787 ) ) ;
#10364=CARTESIAN_POINT ( 'NONE',  ( 55.94051828345053679, 49.20051614449766930, 4.345558710429044069 ) ) ;
#10367=CARTESIAN_POINT ( 'NONE',  ( 47.42335538002188144, 56.59948385550239891, 8.007379884777233059 ) ) ;
#10369=CARTESIAN_POINT ( 'NONE',  ( 56.79116909180255135, 51.79948385550240175, -4.963592699179005585 ) ) ;
#10378=CARTESIAN_POINT ( 'NONE',  ( 53.54508667620428497, 60.29948385550240175, 4.840751629271157874 ) ) ;
#10379=CARTESIAN_POINT ( 'NONE',  ( 47.74827507625470702, 62.40051614449765793, -7.007379884777204637 ) ) ;
#10380=CARTESIAN_POINT ( 'NONE',  ( 43.20883090819742023, 60.20051614449766220, -4.963592699178938972 ) ) ;
#10382=CARTESIAN_POINT ( 'NONE',  ( 47.37792948025170858, 51.60051614449766788, 7.992620115222797139 ) ) ;
#10395=CARTESIAN_POINT ( 'NONE',  ( 52.25172492374522903, 63.59948385550237759, -7.007379884777225953 ) ) ;
#10396=CARTESIAN_POINT ( 'NONE',  ( 56.65037692655918988, 61.89948385550241028, -2.184720259617163762 ) ) ;
#10397=CARTESIAN_POINT ( 'NONE',  ( 52.25172492374527877, 61.40051614449765083, 7.007379884777203749 ) ) ;
#10402=CARTESIAN_POINT ( 'NONE',  ( 50.02271294988505446, 50.50051614449765935, -7.000000000000000888 ) ) ;
#10403=CARTESIAN_POINT ( 'NONE',  ( 43.69122665457040000, 52.99948385550241170, 0.02388180880521036456 ) ) ;
#10414=CARTESIAN_POINT ( 'NONE',  ( 44.88205777487401349, 45.80051614449766362, 3.688883143319584779 ) ) ;
#10417=CARTESIAN_POINT ( 'NONE',  ( 55.96859303347804371, 52.19948385550240033, 4.306917132069425946 ) ) ;
#10423=CARTESIAN_POINT ( 'NONE',  ( 47.70284917648453415, 53.39948385550238186, -6.992620115222774047 ) ) ;
#10433=CARTESIAN_POINT ( 'NONE',  ( 47.74827507625477807, 46.59948385550239180, 7.007379884777229506 ) ) ;
#10434=CARTESIAN_POINT ( 'NONE',  ( 50.02271294988505446, 46.50051614449765935, -7.000000000000000888 ) ) ;
#10436=CARTESIAN_POINT ( 'NONE',  ( 45.27934281921075410, 63.29948385550240175, -6.458785618021043895 ) ) ;
#10439=CARTESIAN_POINT ( 'NONE',  ( 49.97728705011486738, 59.49948385550240459, -8.000000000000001776 ) ) ;
#10442=CARTESIAN_POINT ( 'NONE',  ( 54.89903213687075834, 44.74560054925188268, -5.000000000000007105 ) ) ;
#10448=CARTESIAN_POINT ( 'NONE',  ( 51.92680522751238925, 49.40051614449766504, 6.007379884777208190 ) ) ;
#10449=CARTESIAN_POINT ( 'NONE',  ( 52.25172492374528588, 59.40051614449765793, 7.007379884777204637 ) ) ;
#10450=CARTESIAN_POINT ( 'NONE',  ( 42.39856655714564226, 64.10051614449766078, -2.493737253992044156 ) ) ;
#10452=CARTESIAN_POINT ( 'NONE',  ( 58.41169779390614281, 47.00051614449766646, 0.02388180880515032231 ) ) ;
#10461=CARTESIAN_POINT ( 'NONE',  ( 44.28664221472220675, 53.09948385550240602, -1.832500667257165317 ) ) ;
#10462=CARTESIAN_POINT ( 'NONE',  ( 54.13287192849676188, 62.29948385550240886, 5.649768623646098220 ) ) ;
#10463=CARTESIAN_POINT ( 'NONE',  ( 54.13287192849671214, 58.70051614449765509, -5.649768623646139964 ) ) ;
#10468=CARTESIAN_POINT ( 'NONE',  ( 45.90387839640208512, 52.30051614449766362, -5.676469297603124353 ) ) ;
#10469=CARTESIAN_POINT ( 'NONE',  ( 46.45491332379572924, 57.29948385550240175, -4.840751629271157874 ) ) ;
#10479=CIRCLE ( 'NONE', #11592, 0.4999999999999972244 ) ;
#10483=CARTESIAN_POINT ( 'NONE',  ( 55.71335778527780036, 52.90051614449766504, -1.832500667257213056 ) ) ;
#10487=CARTESIAN_POINT ( 'NONE',  ( 50.02271294988512551, 62.49948385550240459, 7.000000000000000888 ) ) ;
#10488=CARTESIAN_POINT ( 'NONE',  ( 55.96859303347804371, 58.19948385550241454, 4.306917132069425946 ) ) ;
#10499=CARTESIAN_POINT ( 'NONE',  ( 45.90387839640208512, 48.30051614449765651, -5.676469297603124353 ) ) ;
#10502=CARTESIAN_POINT ( 'NONE',  ( 45.31609314410967926, 64.69948385550240744, 6.485486291978119766 ) ) ;
#10504=CARTESIAN_POINT ( 'NONE',  ( 52.57664461997811856, 55.59948385550240602, -8.007379884777229506 ) ) ;
#10513=CARTESIAN_POINT ( 'NONE',  ( 46.45491332379576477, 47.70051614449766220, 4.840751629271188961 ) ) ;
#10515=CARTESIAN_POINT ( 'NONE',  ( 49.97728705011495265, 57.50051614449766646, 7.000000000000000888 ) ) ;
#10516=CARTESIAN_POINT ( 'NONE',  ( 47.42335538002180328, 64.40051614449764372, -8.007379884777206414 ) ) ;
#10518=CARTESIAN_POINT ( 'NONE',  ( 58.41169779390614281, 57.00051614449766646, 0.02388180880515032231 ) ) ;
#10530=CARTESIAN_POINT ( 'NONE',  ( 48.07319477248768180, 48.59948385550239891, 6.007379884777225953 ) ) ;
#10533=CARTESIAN_POINT ( 'NONE',  ( 54.68390685589039890, 49.30051614449766362, 6.485486291978072693 ) ) ;
#10537=CARTESIAN_POINT ( 'NONE',  ( 56.66441430157294690, 54.90051614449765793, -2.141517661632166281 ) ) ;
#10538=CARTESIAN_POINT ( 'NONE',  ( 56.30877334542961421, 59.99948385550241170, -0.02388180880520959434 ) ) ;
#10547=CARTESIAN_POINT ( 'NONE',  ( 57.36023556966787851, 49.99948385550238328, -0.02388180880522424582 ) ) ;
#10549=CARTESIAN_POINT ( 'NONE',  ( 46.49166364869456913, 52.30051614449766362, -4.867452303228181343 ) ) ;
#10551=CARTESIAN_POINT ( 'NONE',  ( 45.90387839640214196, 62.69948385550240744, 5.676469297603166098 ) ) ;
#10552=CARTESIAN_POINT ( 'NONE',  ( 47.70284917648453415, 61.39948385550241738, -6.992620115222774047 ) ) ;
#10553=CARTESIAN_POINT ( 'NONE',  ( 50.02271294988512551, 62.49948385550240459, 7.000000000000000888 ) ) ;
#10563=CARTESIAN_POINT ( 'NONE',  ( 52.25172492374527877, 49.40051614449766504, 7.007379884777203749 ) ) ;
#10566=CARTESIAN_POINT ( 'NONE',  ( 41.58830220609386430, 64.99948385550240459, 0.02388180880523263147 ) ) ;
#10569=CARTESIAN_POINT ( 'NONE',  ( 43.18075615816989199, 57.19948385550241454, -4.924951120819313743 ) ) ;
#10573=ORIENTED_EDGE ( 'NONE', *, *, #10798, .F. ) ;
#10581=CARTESIAN_POINT ( 'NONE',  ( 51.97223112728249816, 48.60051614449766788, -5.992620115222793586 ) ) ;
#10582=CARTESIAN_POINT ( 'NONE',  ( 56.65037692655921120, 59.10051614449766078, 2.184720259617097593 ) ) ;
#10584=CARTESIAN_POINT ( 'NONE',  ( 54.72065718078924590, 46.29948385550240886, 6.458785618021043895 ) ) ;
#10586=CARTESIAN_POINT ( 'NONE',  ( 54.68390685589039890, 53.30051614449767072, 6.485486291978072693 ) ) ;
#10600=CARTESIAN_POINT ( 'NONE',  ( 43.69122665457040000, 48.99948385550241170, 0.02388180880521036456 ) ) ;
#10601=CARTESIAN_POINT ( 'NONE',  ( 44.05948171654949874, 62.79948385550240886, 4.345558710429104465 ) ) ;
#10602=CARTESIAN_POINT ( 'NONE',  ( 43.20883090819742023, 48.20051614449766930, -4.963592699178938972 ) ) ;
#10605=CARTESIAN_POINT ( 'NONE',  ( 44.03140696652198471, 59.80051614449766362, 4.306917132069485454 ) ) ;
#10606=CARTESIAN_POINT ( 'NONE',  ( 44.28664221472220675, 61.09948385550241312, -1.832500667257165317 ) ) ;
#10617=CARTESIAN_POINT ( 'NONE',  ( 47.70284917648453415, 49.39948385550238896, -6.992620115222774047 ) ) ;
#10620=CARTESIAN_POINT ( 'NONE',  ( 55.11794222512599362, 52.80051614449766362, -3.688883143319583446 ) ) ;
#10622=CARTESIAN_POINT ( 'NONE',  ( 45.90387839640214196, 64.69948385550240744, 5.676469297603166098 ) ) ;
#10624=CARTESIAN_POINT ( 'NONE',  ( 44.03140696652192787, 57.19948385550238612, -4.306917132069425058 ) ) ;
#10633=CARTESIAN_POINT ( 'NONE',  ( 45.90387839640214196, 50.69948385550240744, 5.676469297603166098 ) ) ;
#10635=CARTESIAN_POINT ( 'NONE',  ( 54.09612160359792199, 47.30051614449765651, 5.676469297603124353 ) ) ;
#10640=CARTESIAN_POINT ( 'NONE',  ( 54.09612160359786515, 45.69948385550240744, -5.676469297603166098 ) ) ;
#10642=PRODUCT_DEFINITION ( 'UNKNOWN', '', #4194, #8186 ) ;
#10643=CARTESIAN_POINT ( 'NONE',  ( 50.02271294988513972, 58.49948385550241170, 8.000000000000001776 ) ) ;
#10650=CARTESIAN_POINT ( 'NONE',  ( 44.91013252490150620, 48.20051614449766930, -3.727524721679154940 ) ) ;
#10651=CARTESIAN_POINT ( 'NONE',  ( 45.86712807150329496, 57.70051614449765509, 5.649768623646139964 ) ) ;
#10652=CARTESIAN_POINT ( 'NONE',  ( 41.58830220609386430, 46.99948385550239749, 0.02388180880523263147 ) ) ;
#10655=CARTESIAN_POINT ( 'NONE',  ( 41.58830220609386430, 56.00051614449765935, -0.02388180880514929535 ) ) ;
#10668=CARTESIAN_POINT ( 'NONE',  ( 44.91013252490152752, 50.79948385550240175, 3.727524721679198461 ) ) ;
#10671=CARTESIAN_POINT ( 'NONE',  ( 50.02271294988505446, 44.50051614449765935, -8.000000000000001776 ) ) ;
#10675=CARTESIAN_POINT ( 'NONE',  ( 47.70284917648459100, 57.60051614449764656, 6.992620115222796251 ) ) ;
#10676=CARTESIAN_POINT ( 'NONE',  ( 53.54508667620428497, 58.29948385550240886, 4.840751629271157874 ) ) ;
#10685=CARTESIAN_POINT ( 'NONE',  ( 45.90387839640214196, 52.69948385550240033, 5.676469297603166098 ) ) ;
#10687=CARTESIAN_POINT ( 'NONE',  ( 49.97728705011494554, 51.50051614449765935, 6.000000000000000888 ) ) ;
#10692=CARTESIAN_POINT ( 'NONE',  ( 57.36023556966787851, 59.99948385550240459, -0.02388180880522424582 ) ) ;
#10703=CARTESIAN_POINT ( 'NONE',  ( 45.86712807150323812, 55.29948385550240175, -5.649768623646098220 ) ) ;
#10705=CARTESIAN_POINT ( 'NONE',  ( 52.29715082351538769, 52.60051614449766788, -6.992620115222796251 ) ) ;
#10707=CARTESIAN_POINT ( 'NONE',  ( 58.41169779390614281, 63.99948385550241170, -0.02388180880523160798 ) ) ;
#10710=CARTESIAN_POINT ( 'NONE',  ( 41.58830220609386430, 56.99948385550241170, 0.02388180880523263147 ) ) ;
#10715=CARTESIAN_POINT ( 'NONE',  ( 48.07319477248762496, 50.40051614449766504, -6.007379884777208190 ) ) ;
#10717=CARTESIAN_POINT ( 'NONE',  ( 58.41169779390614281, 45.99948385550240459, -0.02388180880523160798 ) ) ;
#10719=CARTESIAN_POINT ( 'NONE',  ( 47.42335538002180328, 56.40051614449765793, -8.007379884777206414 ) ) ;
#10721=EDGE_LOOP ( 'NONE', ( #10573, #1807, #937 ) ) ;
#10729=CARTESIAN_POINT ( 'NONE',  ( 44.88205777487398507, 51.19948385550240744, -3.688883143319540814 ) ) ;
#10730=CARTESIAN_POINT ( 'NONE',  ( 47.70284917648453415, 65.39948385550239607, -6.992620115222774047 ) ) ;
#10731=CARTESIAN_POINT ( 'NONE',  ( 58.41169779390614281, 47.00051614449766646, 0.02388180880515032231 ) ) ;
#10735=CARTESIAN_POINT ( 'NONE',  ( 45.90387839640208512, 56.30051614449765651, -5.676469297603124353 ) ) ;
#10736=CARTESIAN_POINT ( 'NONE',  ( 56.30877334542961421, 55.99948385550241170, -0.02388180880520959434 ) ) ;
#10748=CARTESIAN_POINT ( 'NONE',  ( 43.33558569842703179, 49.09948385550240602, -2.141517661632099223 ) ) ;
#10750=CARTESIAN_POINT ( 'NONE',  ( 55.11794222512599362, 50.80051614449766362, -3.688883143319583446 ) ) ;
#10752=CARTESIAN_POINT ( 'NONE',  ( -74.99999999999997158, 45.00000000000001421, 15.00000000000000000 ) ) ;
#10754=CARTESIAN_POINT ( 'NONE',  ( 52.25172492374522903, 57.59948385550241312, -7.007379884777225953 ) ) ;
#10763=CARTESIAN_POINT ( 'NONE',  ( 49.97728705011488159, 53.49948385550240459, -7.000000000000000888 ) ) ;
#10764=CARTESIAN_POINT ( 'NONE',  ( 47.74827507625469281, 54.40051614449766504, -7.007379884777203749 ) ) ;
#10766=CARTESIAN_POINT ( 'NONE',  ( 44.05948171654949874, 54.79948385550241596, 4.345558710429105354 ) ) ;
#10768=CARTESIAN_POINT ( 'NONE',  ( 57.61547081786812896, 64.09948385550239891, 2.450534656007040901 ) ) ;
#10775=CARTESIAN_POINT ( 'NONE',  ( 51.97223112728249816, 52.60051614449765367, -5.992620115222793586 ) ) ;
#10777=CARTESIAN_POINT ( 'NONE',  ( 43.18075615816989199, 55.19948385550240744, -4.924951120819313743 ) ) ;
#10778=CARTESIAN_POINT ( 'NONE',  ( 55.94051828345050836, 55.79948385550238044, -4.345558710429104465 ) ) ;
#10780=CARTESIAN_POINT ( 'NONE',  ( 50.02271294988505446, 54.50051614449765935, -8.000000000000001776 ) ) ;
#10789=CARTESIAN_POINT ( 'NONE',  ( 51.92680522751233951, 57.59948385550240602, -6.007379884777223289 ) ) ;
#10791=CARTESIAN_POINT ( 'NONE',  ( 44.05948171654945611, 48.20051614449764799, -4.345558710429044069 ) ) ;
#10792=CARTESIAN_POINT ( 'NONE',  ( 49.97728705011495265, 49.50051614449766646, 8.000000000000001776 ) ) ;
#10796=CARTESIAN_POINT ( 'NONE',  ( 54.09612160359792199, 59.30051614449766362, 5.676469297603124353 ) ) ;
#10797=CARTESIAN_POINT ( 'NONE',  ( 44.91013252490152752, 62.79948385550240175, 3.727524721679198461 ) ) ;
#10798=EDGE_CURVE ( 'NONE', #9705, #9468, #797, .T. ) ;
#10808=CARTESIAN_POINT ( 'NONE',  ( 52.29715082351547295, 50.39948385550240317, 6.992620115222774047 ) ) ;
#10811=CARTESIAN_POINT ( 'NONE',  ( 51.92680522751238925, 59.40051614449765793, 6.007379884777208190 ) ) ;
#10815=CARTESIAN_POINT ( 'NONE',  ( 44.91013252490152752, 46.79948385550240886, 3.727524721679198461 ) ) ;
#10828=CARTESIAN_POINT ( 'NONE',  ( 42.63976443033212149, 50.99948385550240459, 0.02388180880522514787 ) ) ;
#10829=CARTESIAN_POINT ( 'NONE',  ( 54.13287192849671214, 50.70051614449766220, -5.649768623646139964 ) ) ;
#10831=CARTESIAN_POINT ( 'NONE',  ( 52.25172492374522903, 53.59948385550241312, -7.007379884777225953 ) ) ;
#10835=CARTESIAN_POINT ( 'NONE',  ( 45.27934281921075410, 63.29948385550240175, -6.458785618021043895 ) ) ;
#10843=CARTESIAN_POINT ( 'NONE',  ( 44.91013252490150620, 54.20051614449766220, -3.727524721679154940 ) ) ;
#10845=CARTESIAN_POINT ( 'NONE',  ( 45.27934281921075410, 55.29948385550240175, -6.458785618021043895 ) ) ;
#10847=CARTESIAN_POINT ( 'NONE',  ( 56.66441430157296821, 54.09948385550240602, 2.141517661632100111 ) ) ;
#10849=CARTESIAN_POINT ( 'NONE',  ( 57.61547081786810764, 62.90051614449765083, -2.450534656007114176 ) ) ;
#10863=CARTESIAN_POINT ( 'NONE',  ( 55.69932041026404335, 55.89948385550241028, -1.875703265242203432 ) ) ;
#10864=CARTESIAN_POINT ( 'NONE',  ( 44.03140696652198471, 45.80051614449766362, 4.306917132069485454 ) ) ;
#10865=CARTESIAN_POINT ( 'NONE',  ( 57.60143344285435774, 55.10051614449765367, 2.493737253992045044 ) ) ;
#10868=CARTESIAN_POINT ( 'NONE',  ( 52.57664461997821093, 45.40051614449765793, 8.007379884777206414 ) ) ;
#10877=CARTESIAN_POINT ( 'NONE',  ( 47.74827507625478518, 58.59948385550238470, 7.007379884777227730 ) ) ;
#10879=CARTESIAN_POINT ( 'NONE',  ( 55.08986747509849380, 55.20051614449766220, 3.727524721679155384 ) ) ;
#10883=CARTESIAN_POINT ( 'NONE',  ( 53.50833635130540955, 47.69948385550240744, -4.867452303228209765 ) ) ;
#10896=CARTESIAN_POINT ( 'NONE',  ( 52.29715082351538769, 50.60051614449766788, -6.992620115222796251 ) ) ;
#10898=CARTESIAN_POINT ( 'NONE',  ( 45.90387839640214196, 50.69948385550240744, 5.676469297603166098 ) ) ;
#10899=CARTESIAN_POINT ( 'NONE',  ( 52.62207051974839089, 64.39948385550239607, 7.992620115222770494 ) ) ;
#10913=CARTESIAN_POINT ( 'NONE',  ( 53.54508667620424234, 56.70051614449766930, -4.840751629271188961 ) ) ;
#10916=CARTESIAN_POINT ( 'NONE',  ( 56.79116909180255135, 55.79948385550239465, -4.963592699179005585 ) ) ;
#10917=CARTESIAN_POINT ( 'NONE',  ( 43.33558569842703179, 55.09948385550241312, -2.141517661632099223 ) ) ;
#10920=CARTESIAN_POINT ( 'NONE',  ( 45.31609314410960820, 62.30051614449766362, -6.485486291978072693 ) ) ;
#10932=CARTESIAN_POINT ( 'NONE',  ( 56.30877334542961421, 57.99948385550241170, -0.02388180880520959434 ) ) ;
#10933=CARTESIAN_POINT ( 'NONE',  ( 47.70284917648459810, 45.60051614449765367, 6.992620115222797139 ) ) ;
#10934=CARTESIAN_POINT ( 'NONE',  ( 47.37792948025170858, 53.60051614449765367, 7.992620115222797139 ) ) ;
#10937=CARTESIAN_POINT ( 'NONE',  ( 47.37792948025170858, 45.60051614449765367, 7.992620115222797139 ) ) ;
#10948=CARTESIAN_POINT ( 'NONE',  ( 44.05948171654949874, 58.79948385550240886, 4.345558710429105354 ) ) ;
#10949=CARTESIAN_POINT ( 'NONE',  ( 44.30067958973594955, 56.10051614449766078, -1.875703265242155693 ) ) ;
#10952=CARTESIAN_POINT ( 'NONE',  ( 47.74827507625469281, 46.40051614449764372, -7.007379884777203749 ) ) ;
#10953=CARTESIAN_POINT ( 'NONE',  ( 55.11794222512601493, 48.19948385550240744, 3.688883143319541702 ) ) ;
#10964=CARTESIAN_POINT ( 'NONE',  ( 42.63976443033212860, 56.00051614449765935, -0.02388180880514948964 ) ) ;
#10967=CARTESIAN_POINT ( 'NONE',  ( 44.03140696652192787, 53.19948385550238612, -4.306917132069425058 ) ) ;
#10968=CARTESIAN_POINT ( 'NONE',  ( 56.66441430157296821, 50.09948385550240602, 2.141517661632100111 ) ) ;
#10969=CARTESIAN_POINT ( 'NONE',  ( 41.58830220609386430, 60.99948385550241170, 0.02388180880523263147 ) ) ;
#10977=CARTESIAN_POINT ( 'NONE',  ( 46.49166364869456913, 54.30051614449765651, -4.867452303228181343 ) ) ;
#10979=CARTESIAN_POINT ( 'NONE',  ( 49.97728705011486738, 53.49948385550240459, -8.000000000000001776 ) ) ;
#10980=CARTESIAN_POINT ( 'NONE',  ( 52.29715082351547295, 58.39948385550238896, 6.992620115222774047 ) ) ;
#10982=CARTESIAN_POINT ( 'NONE',  ( 52.57664461997811856, 45.59948385550240602, -8.007379884777229506 ) ) ;
#10990=DIRECTION ( 'NONE',  ( 0.000000000000000000, 0.000000000000000000, 1.000000000000000000 ) ) ;
#10993=CARTESIAN_POINT ( 'NONE',  ( 44.30067958973596376, 56.89948385550240317, 1.875703265242204099 ) ) ;
#10994=CARTESIAN_POINT ( 'NONE',  ( 54.09612160359792199, 47.30051614449765651, 5.676469297603124353 ) ) ;
#10995=CARTESIAN_POINT ( 'NONE',  ( 42.39856655714564226, 54.10051614449766078, -2.493737253992044156 ) ) ;
#10997=FACE_OUTER_BOUND ( 'NONE', #4672, .T. ) ;
#11000=CARTESIAN_POINT ( 'NONE',  ( 50.02271294988505446, 46.50051614449766646, -8.000000000000001776 ) ) ;
#11012=CARTESIAN_POINT ( 'NONE',  ( 55.96859303347804371, 56.19948385550241454, 4.306917132069425946 ) ) ;
#11014=CARTESIAN_POINT ( 'NONE',  ( 53.50833635130544508, 61.30051614449766362, 4.867452303228181343 ) ) ;
#11017=CARTESIAN_POINT ( 'NONE',  ( 56.65037692655921120, 47.10051614449766078, 2.184720259617097593 ) ) ;
#11018=CARTESIAN_POINT ( 'NONE',  ( 44.88205777487398507, 49.19948385550240744, -3.688883143319540814 ) ) ;
#11031=CARTESIAN_POINT ( 'NONE',  ( 54.13287192849671214, 62.70051614449766220, -5.649768623646139964 ) ) ;
#11034=CARTESIAN_POINT ( 'NONE',  ( 44.03140696652192787, 55.19948385550238612, -4.306917132069425058 ) ) ;
#11035=CARTESIAN_POINT ( 'NONE',  ( 56.65037692655918988, 49.89948385550240317, -2.184720259617163762 ) ) ;
#11037=CARTESIAN_POINT ( 'NONE',  ( 56.79116909180255135, 61.79948385550240175, -4.963592699179005585 ) ) ;
#11046=CARTESIAN_POINT ( 'NONE',  ( 53.50833635130544508, 53.30051614449767072, 4.867452303228181343 ) ) ;
#11049=CARTESIAN_POINT ( 'NONE',  ( 56.79116909180255135, 53.79948385550241596, -4.963592699179005585 ) ) ;
#11050=CARTESIAN_POINT ( 'NONE',  ( 52.25172492374522903, 59.59948385550240602, -7.007379884777225953 ) ) ;
#11052=CARTESIAN_POINT ( 'NONE',  ( 43.20883090819742023, 62.20051614449766220, -4.963592699178938972 ) ) ;
#11061=CARTESIAN_POINT ( 'NONE',  ( 49.99999999999997158, 45.00000000000001421, -7.000000000000000888 ) ) ;
#11062=CARTESIAN_POINT ( 'NONE',  ( 48.07319477248768180, 56.59948385550239891, 6.007379884777225953 ) ) ;
#11063=CARTESIAN_POINT ( 'NONE',  ( 43.34962307344078880, 48.10051614449766078, -2.184720259617096705 ) ) ;
#11064=CARTESIAN_POINT ( 'NONE',  ( 43.18075615816994173, 49.80051614449765651, 4.924951120819380357 ) ) ;
#11070=CARTESIAN_POINT ( 'NONE',  ( 49.97728705011495265, 63.50051614449765935, 7.000000000000000888 ) ) ;
#11083=CARTESIAN_POINT ( 'NONE',  ( 45.86712807150323812, 55.29948385550240175, -5.649768623646098220 ) ) ;
#11084=CARTESIAN_POINT ( 'NONE',  ( 47.70284917648453415, 51.39948385550240317, -6.992620115222774047 ) ) ;
#11085=CARTESIAN_POINT ( 'NONE',  ( 44.88205777487401349, 55.80051614449766362, 3.688883143319584779 ) ) ;
#11089=CARTESIAN_POINT ( 'NONE',  ( 50.02271294988506156, 62.50051614449767357, -6.000000000000000888 ) ) ;
#11090=CARTESIAN_POINT ( 'NONE',  ( 53.50833635130540955, 45.69948385550240033, -4.867452303228209765 ) ) ;
#11103=CARTESIAN_POINT ( 'NONE',  ( 55.94051828345053679, 63.20051614449765509, 4.345558710429044069 ) ) ;
#11106=CARTESIAN_POINT ( 'NONE',  ( 55.96859303347804371, 58.19948385550241454, 4.306917132069425946 ) ) ;
#11107=( NAMED_UNIT ( * ) PLANE_ANGLE_UNIT ( ) SI_UNIT ( $, .RADIAN. ) );
#11108=CARTESIAN_POINT ( 'NONE',  ( 47.70284917648453415, 51.39948385550238896, -6.992620115222774047 ) ) ;
#11116=CARTESIAN_POINT ( 'NONE',  ( 50.02271294988506156, 62.50051614449767357, -6.000000000000000888 ) ) ;
#11118=CARTESIAN_POINT ( 'NONE',  ( 57.61547081786812896, 62.09948385550240602, 2.450534656007040901 ) ) ;
#11119=CARTESIAN_POINT ( 'NONE',  ( 56.66441430157296821, 60.09948385550240602, 2.141517661632100111 ) ) ;
#11122=CARTESIAN_POINT ( 'NONE',  ( 52.62207051974829852, 62.60051614449765367, -7.992620115222797139 ) ) ;
#11135=CARTESIAN_POINT ( 'NONE',  ( 48.07319477248768180, 62.59948385550238470, 6.007379884777225953 ) ) ;
#11136=CARTESIAN_POINT ( 'NONE',  ( 52.29715082351539479, 50.60051614449766078, -6.992620115222796251 ) ) ;
#11138=CARTESIAN_POINT ( 'NONE',  ( 54.68390685589039890, 51.30051614449765651, 6.485486291978072693 ) ) ;
#11142=CARTESIAN_POINT ( 'NONE',  ( 45.86712807150329496, 61.70051614449766220, 5.649768623646139964 ) ) ;
#11152=CARTESIAN_POINT ( 'NONE',  ( 54.13287192849676188, 54.29948385550240886, 5.649768623646098220 ) ) ;
#11153=CARTESIAN_POINT ( 'NONE',  ( 57.36023556966787851, 57.99948385550240459, -0.02388180880522424582 ) ) ;
#11158=CARTESIAN_POINT ( 'NONE',  ( 56.66441430157294690, 44.90051614449765793, -2.141517661632166281 ) ) ;
#11159=CARTESIAN_POINT ( 'NONE',  ( 46.45491332379572924, 53.29948385550240886, -4.840751629271157874 ) ) ;
#11171=CARTESIAN_POINT ( 'NONE',  ( 49.97728705011495265, 61.50051614449765935, 7.000000000000000888 ) ) ;
#11173=CARTESIAN_POINT ( 'NONE',  ( 43.69122665457040000, 48.00051614449766646, -0.02388180880515696977 ) ) ;
#11175=CARTESIAN_POINT ( 'NONE',  ( 52.29715082351547295, 60.39948385550239607, 6.992620115222774047 ) ) ;
#11176=CARTESIAN_POINT ( 'NONE',  ( 54.13287192849676188, 46.29948385550240886, 5.649768623646098220 ) ) ;
#11178=CARTESIAN_POINT ( 'NONE',  ( 44.05948171654949874, 46.79948385550238754, 4.345558710429105354 ) ) ;
#11186=CARTESIAN_POINT ( 'NONE',  ( 51.97223112728249816, 62.60051614449765367, -5.992620115222793586 ) ) ;
#11188=CARTESIAN_POINT ( 'NONE',  ( 52.62207051974839089, 56.39948385550241028, 7.992620115222770494 ) ) ;
#11189=CARTESIAN_POINT ( 'NONE',  ( 54.09612160359786515, 63.69948385550240744, -5.676469297603166098 ) ) ;
#11190=DIRECTION ( 'NONE',  ( 0.04542589977017006536, -0.9989677110047503472, 0.000000000000000000 ) ) ;
#11192=CARTESIAN_POINT ( 'NONE',  ( 45.31609314410967926, 48.69948385550241454, 6.485486291978119766 ) ) ;
#11204=CARTESIAN_POINT ( 'NONE',  ( 44.30067958973596376, 60.89948385550241028, 1.875703265242204099 ) ) ;
#11205=CARTESIAN_POINT ( 'NONE',  ( 54.13287192849671214, 50.70051614449766220, -5.649768623646139964 ) ) ;
#11206=CARTESIAN_POINT ( 'NONE',  ( 54.68390685589039890, 57.30051614449767072, 6.485486291978072693 ) ) ;
#11209=CARTESIAN_POINT ( 'NONE',  ( 49.97728705011495265, 49.50051614449766646, 8.000000000000001776 ) ) ;
#11219=CARTESIAN_POINT ( 'NONE',  ( 44.03140696652192787, 65.19948385550240744, -4.306917132069425058 ) ) ;
#11222=CARTESIAN_POINT ( 'NONE',  ( 43.33558569842703179, 61.09948385550240602, -2.141517661632099223 ) ) ;
#11228=CARTESIAN_POINT ( 'NONE',  ( 44.30067958973594955, 64.10051614449766078, -1.875703265242155693 ) ) ;
#11229=CARTESIAN_POINT ( 'NONE',  ( 46.45491332379572924, 51.29948385550240175, -4.840751629271157874 ) ) ;
#11233=ORIENTED_EDGE ( 'NONE', *, *, #9017, .F. ) ;
#11239=CARTESIAN_POINT ( 'NONE',  ( 54.09612160359786515, 45.69948385550240744, -5.676469297603166098 ) ) ;
#11243=CARTESIAN_POINT ( 'NONE',  ( 48.02776887271745210, 63.39948385550238896, -5.992620115222778487 ) ) ;
#11245=CARTESIAN_POINT ( 'NONE',  ( 47.74827507625478518, 58.59948385550238470, 7.007379884777227730 ) ) ;
#11246=CARTESIAN_POINT ( 'NONE',  ( 52.29715082351547295, 52.39948385550241738, 6.992620115222774047 ) ) ;
#11249=CARTESIAN_POINT ( 'NONE',  ( 52.29715082351547295, 50.39948385550240317, 6.992620115222774047 ) ) ;
#11260=CARTESIAN_POINT ( 'NONE',  ( 43.69122665457040000, 58.00051614449765935, -0.02388180880515696977 ) ) ;
#11263=CARTESIAN_POINT ( 'NONE',  ( 41.58830220609386430, 60.99948385550241170, 0.02388180880523263147 ) ) ;
#11267=CARTESIAN_POINT ( 'NONE',  ( 42.39856655714566358, 52.89948385550241028, 2.493737253992119207 ) ) ;
#11278=CARTESIAN_POINT ( 'NONE',  ( 56.30877334542961421, 45.00051614449765225, 0.02388180880515774693 ) ) ;
#11279=CARTESIAN_POINT ( 'NONE',  ( 42.63976443033212149, 54.00051614449765935, -0.02388180880514948964 ) ) ;
#11280=CARTESIAN_POINT ( 'NONE',  ( 49.97728705011495265, 59.50051614449765935, 8.000000000000001776 ) ) ;
#11282=CARTESIAN_POINT ( 'NONE',  ( 43.18075615816994173, 47.80051614449764941, 4.924951120819380357 ) ) ;
#11293=CARTESIAN_POINT ( 'NONE',  ( 47.70284917648453415, 63.39948385550240317, -6.992620115222774047 ) ) ;
#11295=CARTESIAN_POINT ( 'NONE',  ( 56.65037692655918988, 55.89948385550240317, -2.184720259617163762 ) ) ;
#11298=CARTESIAN_POINT ( 'NONE',  ( 52.29715082351538769, 52.60051614449766788, -6.992620115222796251 ) ) ;
#11299=CARTESIAN_POINT ( 'NONE',  ( 53.50833635130540955, 51.69948385550241454, -4.867452303228209765 ) ) ;
#11310=CARTESIAN_POINT ( 'NONE',  ( 45.86712807150323812, 47.29948385550240886, -5.649768623646098220 ) ) ;
#11313=CARTESIAN_POINT ( 'NONE',  ( 50.02271294988511841, 64.49948385550239038, 6.000000000000000888 ) ) ;
#11315=CARTESIAN_POINT ( 'NONE',  ( 57.36023556966787851, 55.99948385550239038, -0.02388180880522424582 ) ) ;
#11316=CARTESIAN_POINT ( 'NONE',  ( 56.65037692655918988, 53.89948385550240317, -2.184720259617163762 ) ) ;
#11318=CARTESIAN_POINT ( 'NONE',  ( 54.09612160359786515, 51.69948385550240744, -5.676469297603166098 ) ) ;
#11327=CARTESIAN_POINT ( 'NONE',  ( 44.30067958973594955, 60.10051614449766788, -1.875703265242155693 ) ) ;
#11329=CARTESIAN_POINT ( 'NONE',  ( 54.68390685589033495, 57.69948385550241454, -6.485486291978119766 ) ) ;
#11332=CARTESIAN_POINT ( 'NONE',  ( 45.86712807150323812, 65.29948385550241596, -5.649768623646098220 ) ) ;
#11337=CARTESIAN_POINT ( 'NONE',  ( 45.27934281921075410, 47.29948385550241596, -6.458785618021043895 ) ) ;
#11347=DIRECTION ( 'NONE',  ( -1.387778780781445991E-14, 0.000000000000000000, -1.000000000000000000 ) ) ;
#11348=CARTESIAN_POINT ( 'NONE',  ( 50.02271294988511841, 64.49948385550239038, 6.000000000000000888 ) ) ;
#11349=CARTESIAN_POINT ( 'NONE',  ( 50.02271294988505446, 52.50051614449765935, -7.000000000000000888 ) ) ;
#11351=CARTESIAN_POINT ( 'NONE',  ( 52.62207051974829852, 60.60051614449765367, -7.992620115222797139 ) ) ;
#11353=CARTESIAN_POINT ( 'NONE',  ( 56.81924384183006538, 48.80051614449767072, -4.924951120819380357 ) ) ;
#11366=CARTESIAN_POINT ( 'NONE',  ( 42.63976443033212860, 60.99948385550238328, 0.02388180880522514787 ) ) ;
#11367=CARTESIAN_POINT ( 'NONE',  ( 55.96859303347805081, 58.19948385550240744, 4.306917132069425058 ) ) ;
#11372=CARTESIAN_POINT ( 'NONE',  ( 51.03999344061968912, 45.00000000000002132, -7.500000000000003553 ) ) ;
#11373=CARTESIAN_POINT ( 'NONE',  ( 44.03140696652198471, 47.80051614449764230, 4.306917132069485454 ) ) ;
#11374=CARTESIAN_POINT ( 'NONE',  ( 49.97728705011488870, 55.49948385550241170, -6.000000000000000888 ) ) ;
#11387=CARTESIAN_POINT ( 'NONE',  ( 55.69932041026404335, 63.89948385550240317, -1.875703265242203432 ) ) ;
#11389=CARTESIAN_POINT ( 'NONE',  ( 42.63976443033212860, 56.99948385550241170, 0.02388180880522514787 ) ) ;
#11390=CARTESIAN_POINT ( 'NONE',  ( 43.34962307344081012, 54.89948385550240317, 2.184720259617164650 ) ) ;
#11392=CARTESIAN_POINT ( 'NONE',  ( 44.03140696652192787, 49.19948385550240033, -4.306917132069425058 ) ) ;
#11398=CARTESIAN_POINT ( 'NONE',  ( 54.13287192849676188, 48.29948385550240175, 5.649768623646098220 ) ) ;
#11400=CARTESIAN_POINT ( 'NONE',  ( 55.69932041026405045, 59.10051614449766078, 1.875703265242156359 ) ) ;
#11403=CARTESIAN_POINT ( 'NONE',  ( 57.60143344285433642, 61.89948385550241738, -2.493737253992118319 ) ) ;
#11406=CARTESIAN_POINT ( 'NONE',  ( 50.02271294988513972, 52.49948385550241170, 8.000000000000001776 ) ) ;
#11415=CARTESIAN_POINT ( 'NONE',  ( 55.08986747509847248, 63.79948385550241596, -3.727524721679197572 ) ) ;
#11416=CARTESIAN_POINT ( 'NONE',  ( 52.29715082351539479, 56.60051614449766078, -6.992620115222796251 ) ) ;
#11417=CARTESIAN_POINT ( 'NONE',  ( 47.42335538002180328, 58.40051614449765793, -8.007379884777206414 ) ) ;
#11419=CARTESIAN_POINT ( 'NONE',  ( 42.39856655714564226, 52.10051614449766788, -2.493737253992044156 ) ) ;
#11429=CARTESIAN_POINT ( 'NONE',  ( 56.66441430157296821, 62.09948385550239891, 2.141517661632100111 ) ) ;
#11430=CARTESIAN_POINT ( 'NONE',  ( 57.36023556966787851, 61.99948385550240459, -0.02388180880522424582 ) ) ;
#11432=CARTESIAN_POINT ( 'NONE',  ( 56.65037692655921120, 59.10051614449766078, 2.184720259617097593 ) ) ;
#11437=CARTESIAN_POINT ( 'NONE',  ( 55.31939397794342028, 44.99999999999998579, -5.196074157289758411 ) ) ;
#11438=CARTESIAN_POINT ( 'NONE',  ( 56.65037692655921120, 49.10051614449766078, 2.184720259617097593 ) ) ;
#11439=CARTESIAN_POINT ( 'NONE',  ( 44.91013252490152752, 50.79948385550240175, 3.727524721679198461 ) ) ;
#11453=CARTESIAN_POINT ( 'NONE',  ( 49.97728705011494554, 47.50051614449765935, 6.000000000000000888 ) ) ;
#11455=CARTESIAN_POINT ( 'NONE',  ( 49.97728705011488159, 63.49948385550241170, -7.000000000000000888 ) ) ;
#11456=CARTESIAN_POINT ( 'NONE',  ( 47.74827507625478518, 56.59948385550238470, 7.007379884777227730 ) ) ;
#11459=CARTESIAN_POINT ( 'NONE',  ( 42.63976443033212860, 52.99948385550240459, 0.02388180880522514787 ) ) ;
#11469=CARTESIAN_POINT ( 'NONE',  ( 52.25172492374522903, 45.59948385550240602, -7.007379884777227730 ) ) ;
#11470=CARTESIAN_POINT ( 'NONE',  ( 52.29715082351538769, 46.60051614449766078, -6.992620115222796251 ) ) ;
#11475=CARTESIAN_POINT ( 'NONE',  ( 56.66441430157296821, 48.09948385550240602, 2.141517661632100111 ) ) ;
#11478=CARTESIAN_POINT ( 'NONE',  ( 58.41169779390614281, 47.99948385550239038, -0.02388180880523160798 ) ) ;
#11483=CARTESIAN_POINT ( 'NONE',  ( 54.65205120807737416, 44.75923773080658918, -4.999999999999772626 ) ) ;
#11491=CARTESIAN_POINT ( 'NONE',  ( 53.50833635130544508, 51.30051614449765651, 4.867452303228181343 ) ) ;
#11492=CARTESIAN_POINT ( 'NONE',  ( 43.33558569842706021, 57.90051614449766504, 2.141517661632167169 ) ) ;
#11493=CARTESIAN_POINT ( 'NONE',  ( 54.72065718078918906, 60.70051614449766930, -6.458785618021089192 ) ) ;
#11495=CARTESIAN_POINT ( 'NONE',  ( 54.68390685589039890, 47.30051614449766362, 6.485486291978072693 ) ) ;
#11501=ORIENTED_EDGE ( 'NONE', *, *, #22, .T. ) ;
#11503=CARTESIAN_POINT ( 'NONE',  ( 49.99999999999997158, 45.00000000000003553, -7.000000000000000888 ) ) ;
#11508=CARTESIAN_POINT ( 'NONE',  ( 45.86712807150323812, 61.29948385550240886, -5.649768623646098220 ) ) ;
#11510=CARTESIAN_POINT ( 'NONE',  ( 50.02271294988505446, 62.50051614449766646, -7.000000000000000888 ) ) ;
#11515=CARTESIAN_POINT ( 'NONE',  ( 44.05948171654945611, 50.20051614449764088, -4.345558710429044069 ) ) ;
#11516=CARTESIAN_POINT ( 'NONE',  ( 56.30877334542961421, 61.99948385550241170, -0.02388180880520959434 ) ) ;
#11533=CARTESIAN_POINT ( 'NONE',  ( 53.54508667620424234, 50.70051614449766220, -4.840751629271188961 ) ) ;
#11535=CARTESIAN_POINT ( 'NONE',  ( 47.74827507625478518, 64.59948385550239891, 7.007379884777227730 ) ) ;
#11536=CARTESIAN_POINT ( 'NONE',  ( 52.25172492374522903, 55.59948385550241312, -7.007379884777225953 ) ) ;
#11547=CARTESIAN_POINT ( 'NONE',  ( 49.97728705011488159, 47.49948385550240459, -7.000000000000000888 ) ) ;
#11548=CARTESIAN_POINT ( 'NONE',  ( 44.05948171654945611, 46.20051614449766930, -4.345558710429044069 ) ) ;
#11550=CARTESIAN_POINT ( 'NONE',  ( 42.63976443033212860, 46.99948385550240459, 0.02388180880522514787 ) ) ;
#11552=CARTESIAN_POINT ( 'NONE',  ( 52.57664461997811856, 57.59948385550240602, -8.007379884777229506 ) ) ;
#11563=CARTESIAN_POINT ( 'NONE',  ( 49.97728705011494554, 47.50051614449765935, 6.000000000000000888 ) ) ;
#11564=CARTESIAN_POINT ( 'NONE',  ( 55.96859303347802239, 62.80051614449766362, -4.306917132069484566 ) ) ;
#11565=CARTESIAN_POINT ( 'NONE',  ( 57.61547081786812896, 48.09948385550240602, 2.450534656007040901 ) ) ;
#11567=CARTESIAN_POINT ( 'NONE',  ( 43.18075615816994173, 53.80051614449766362, 4.924951120819380357 ) ) ;
#11575=CARTESIAN_POINT ( 'NONE',  ( 46.49166364869460466, 48.69948385550241454, 4.867452303228209765 ) ) ;
#11576=CARTESIAN_POINT ( 'NONE',  ( 45.90387839640214196, 64.69948385550240744, 5.676469297603166098 ) ) ;
#11578=CARTESIAN_POINT ( 'NONE',  ( 56.81924384183006538, 44.80051614449766362, -4.924951120819380357 ) ) ;
#11582=CARTESIAN_POINT ( 'NONE',  ( 52.25172492374527877, 51.40051614449767214, 7.007379884777203749 ) ) ;
#11583=CARTESIAN_POINT ( 'NONE',  ( 48.07319477248768180, 56.59948385550239891, 6.007379884777225953 ) ) ;
#11592=AXIS2_PLACEMENT_3D ( 'NONE', #3442, #2121, #7664 ) ;
#11594=CARTESIAN_POINT ( 'NONE',  ( 55.96859303347804371, 50.19948385550240744, 4.306917132069425946 ) ) ;
#11596=CARTESIAN_POINT ( 'NONE',  ( 48.02776887271750184, 49.60051614449766788, 5.992620115222795363 ) ) ;
#11601=CARTESIAN_POINT ( 'NONE',  ( 55.96859303347804371, 64.19948385550239323, 4.306917132069425946 ) ) ;
#11602=CARTESIAN_POINT ( 'NONE',  ( 42.63976443033212860, 58.99948385550239038, 0.02388180880522514787 ) ) ;
#11610=CARTESIAN_POINT ( 'NONE',  ( 44.03140696652193498, 47.19948385550240744, -4.306917132069424170 ) ) ;
#11611=CARTESIAN_POINT ( 'NONE',  ( 55.96859303347802239, 46.80051614449767072, -4.306917132069484566 ) ) ;
#11613=CARTESIAN_POINT ( 'NONE',  ( 45.31609314410967926, 62.69948385550240744, 6.485486291978119766 ) ) ;
#11616=CARTESIAN_POINT ( 'NONE',  ( 41.58830220609386430, 58.99948385550239749, 0.02388180880523263147 ) ) ;
#11624=CARTESIAN_POINT ( 'NONE',  ( 51.92680522751238925, 47.40051614449765793, 6.007379884777208190 ) ) ;
#11625=CARTESIAN_POINT ( 'NONE',  ( 45.86712807150329496, 59.70051614449766220, 5.649768623646139964 ) ) ;
#11626=CARTESIAN_POINT ( 'NONE',  ( 52.57664461997811856, 49.59948385550241312, -8.007379884777229506 ) ) ;
#11628=CARTESIAN_POINT ( 'NONE',  ( 54.68390685589039890, 55.30051614449765651, 6.485486291978072693 ) ) ;
#11637=CARTESIAN_POINT ( 'NONE',  ( 55.11794222512601493, 48.19948385550240744, 3.688883143319541702 ) ) ;
#11638=CARTESIAN_POINT ( 'NONE',  ( 52.25172492374522903, 63.59948385550239180, -7.007379884777227730 ) ) ;
#11639=CARTESIAN_POINT ( 'NONE',  ( 56.79116909180259398, 45.20051614449766220, 4.963592699178938972 ) ) ;
#11642=CARTESIAN_POINT ( 'NONE',  ( 52.29715082351538769, 56.60051614449766788, -6.992620115222796251 ) ) ;
#11643=CARTESIAN_POINT ( 'NONE',  ( 48.02776887271745210, 59.39948385550240317, -5.992620115222778487 ) ) ;
#11649=EDGE_CURVE ( 'NONE', #9468, #7204, #745, .T. ) ;
#11652=CARTESIAN_POINT ( 'NONE',  ( 45.90387839640214196, 50.69948385550240744, 5.676469297603166098 ) ) ;
#11654=CARTESIAN_POINT ( 'NONE',  ( 50.02271294988506156, 50.50051614449765935, -6.000000000000000888 ) ) ;
#11656=CARTESIAN_POINT ( 'NONE',  ( 43.34962307344081012, 64.89948385550239607, 2.184720259617164650 ) ) ;
#11658=CARTESIAN_POINT ( 'NONE',  ( 55.96859303347804371, 60.19948385550240744, 4.306917132069425946 ) ) ;
#11665=CARTESIAN_POINT ( 'NONE',  ( 45.86712807150323812, 49.29948385550240175, -5.649768623646098220 ) ) ;
#11666=CARTESIAN_POINT ( 'NONE',  ( 55.94051828345053679, 45.20051614449764088, 4.345558710429044069 ) ) ;
#11670=CARTESIAN_POINT ( 'NONE',  ( 47.37792948025162332, 65.39948385550239607, -7.992620115222770494 ) ) ;
#11673=CARTESIAN_POINT ( 'NONE',  ( 57.60143344285433642, 53.89948385550240317, -2.493737253992118319 ) ) ;
#11683=CARTESIAN_POINT ( 'NONE',  ( 44.28664221472221385, 45.90051614449766504, 1.832500667257213722 ) ) ;
#11684=CARTESIAN_POINT ( 'NONE',  ( 55.96859303347802239, 58.80051614449765651, -4.306917132069484566 ) ) ;
#11686=CARTESIAN_POINT ( 'NONE',  ( 45.27934281921082516, 63.70051614449766930, 6.458785618021089192 ) ) ;
#11688=CARTESIAN_POINT ( 'NONE',  ( 52.57664461997821093, 55.40051614449767214, 8.007379884777206414 ) ) ;
#11690=ORIENTED_EDGE ( 'NONE', *, *, #3106, .F. ) ;
#11698=CARTESIAN_POINT ( 'NONE',  ( 48.07319477248768180, 50.59948385550240602, 6.007379884777225953 ) ) ;
#11699=CARTESIAN_POINT ( 'NONE',  ( 44.05948171654949874, 64.79948385550240175, 4.345558710429104465 ) ) ;
#11700=CARTESIAN_POINT ( 'NONE',  ( 57.61547081786810764, 48.90051614449766504, -2.450534656007114176 ) ) ;
#11705=CARTESIAN_POINT ( 'NONE',  ( 55.94051828345053679, 59.20051614449766220, 4.345558710429044069 ) ) ;
#11707=CARTESIAN_POINT ( 'NONE',  ( 46.49166364869460466, 60.69948385550240033, 4.867452303228209765 ) ) ;
#11717=CARTESIAN_POINT ( 'NONE',  ( 43.34962307344081012, 48.89948385550240317, 2.184720259617164650 ) ) ;
#11720=CARTESIAN_POINT ( 'NONE',  ( 46.45491332379576477, 51.70051614449765509, 4.840751629271188961 ) ) ;
#11724=CARTESIAN_POINT ( 'NONE',  ( 43.33558569842703179, 57.09948385550240602, -2.141517661632099223 ) ) ;
#11725=CARTESIAN_POINT ( 'NONE',  ( 50.02271294988505446, 64.50051614449765225, -7.000000000000000888 ) ) ;
#11728=UNCERTAINTY_MEASURE_WITH_UNIT (LENGTH_MEASURE( 1.000000000000000082E-05 ), #5726, 'distance_accuracy_value', 'NONE');
#11736=CARTESIAN_POINT ( 'NONE',  ( 42.63976443033212149, 52.99948385550240459, 0.02388180880522514787 ) ) ;
#11738=CARTESIAN_POINT ( 'NONE',  ( 43.34962307344078880, 48.10051614449766078, -2.184720259617096705 ) ) ;
#11741=CARTESIAN_POINT ( 'NONE',  ( 49.97728705011488159, 47.49948385550240459, -7.000000000000000888 ) ) ;
#11743=CARTESIAN_POINT ( 'NONE',  ( 49.97728705011486738, 55.49948385550241170, -8.000000000000001776 ) ) ;
#11751=CARTESIAN_POINT ( 'NONE',  ( 56.30877334542961421, 47.00051614449766646, 0.02388180880515774693 ) ) ;
#11752=CARTESIAN_POINT ( 'NONE',  ( 43.34962307344078880, 62.10051614449766078, -2.184720259617096705 ) ) ;
#11754=CARTESIAN_POINT ( 'NONE',  ( 52.57664461997811856, 47.59948385550239891, -8.007379884777229506 ) ) ;
#11757=CARTESIAN_POINT ( 'NONE',  ( 47.37792948025170858, 55.60051614449765367, 7.992620115222797139 ) ) ;
#11770=CARTESIAN_POINT ( 'NONE',  ( 55.71335778527780747, 52.09948385550241312, 1.832500667257165983 ) ) ;
#11772=CARTESIAN_POINT ( 'NONE',  ( 42.38452918213190657, 47.90051614449765793, 2.450534656007115508 ) ) ;
#11775=CARTESIAN_POINT ( 'NONE',  ( 44.05948171654945611, 58.20051614449764799, -4.345558710429044069 ) ) ;
#11776=CARTESIAN_POINT ( 'NONE',  ( 53.50833635130540955, 59.69948385550240744, -4.867452303228209765 ) ) ;
#11778=CARTESIAN_POINT ( 'NONE',  ( 49.97728705011488159, 45.49948385550240459, -7.000000000000000888 ) ) ;
#11784=CARTESIAN_POINT ( 'NONE',  ( 44.05948171654949874, 48.79948385550238754, 4.345558710429105354 ) ) ;
#11786=CARTESIAN_POINT ( 'NONE',  ( 46.45491332379576477, 53.70051614449766220, 4.840751629271188961 ) ) ;
#11792=CARTESIAN_POINT ( 'NONE',  ( 47.70284917648453415, 59.39948385550241028, -6.992620115222774047 ) ) ;
#11803=CARTESIAN_POINT ( 'NONE',  ( 43.34962307344081012, 52.89948385550240317, 2.184720259617164650 ) ) ;
#11805=CARTESIAN_POINT ( 'NONE',  ( 45.90387839640208512, 56.30051614449765651, -5.676469297603124353 ) ) ;
#11807=CARTESIAN_POINT ( 'NONE',  ( 42.63976443033212860, 50.99948385550240459, 0.02388180880522514787 ) ) ;
#11810=CARTESIAN_POINT ( 'NONE',  ( 45.27934281921075410, 59.29948385550240886, -6.458785618021043895 ) ) ;
#11815=CARTESIAN_POINT ( 'NONE',  ( 56.30877334542961421, 55.00051614449766646, 0.02388180880515774693 ) ) ;
#11816=CARTESIAN_POINT ( 'NONE',  ( 52.25172492374528588, 63.40051614449765083, 7.007379884777204637 ) ) ;
#11818=CARTESIAN_POINT ( 'NONE',  ( 42.38452918213190657, 63.90051614449765793, 2.450534656007115508 ) ) ;
#11819=CARTESIAN_POINT ( 'NONE',  ( 47.74827507625478518, 56.59948385550238470, 7.007379884777227730 ) ) ;
#11822=CARTESIAN_POINT ( 'NONE',  ( 49.97728705011495265, 57.50051614449766646, 8.000000000000001776 ) ) ;
#11832=CARTESIAN_POINT ( 'NONE',  ( 44.88205777487398507, 55.19948385550240744, -3.688883143319540814 ) ) ;
#11833=CARTESIAN_POINT ( 'NONE',  ( 54.09612160359792199, 49.30051614449765651, 5.676469297603124353 ) ) ;
#11834=CARTESIAN_POINT ( 'NONE',  ( 47.37792948025170858, 47.60051614449766078, 7.992620115222797139 ) ) ;
#11835=APPLICATION_CONTEXT ( 'automotive_design' ) ;
#11840=CARTESIAN_POINT ( 'NONE',  ( 50.02271294988505446, 56.50051614449766646, -7.000000000000000888 ) ) ;
#11841=CARTESIAN_POINT ( 'NONE',  ( 55.11794222512601493, 62.19948385550240744, 3.688883143319541702 ) ) ;
#11852=CARTESIAN_POINT ( 'NONE',  ( 54.09612160359786515, 51.69948385550240744, -5.676469297603166098 ) ) ;
#11855=CARTESIAN_POINT ( 'NONE',  ( 55.08986747509849380, 57.20051614449766220, 3.727524721679155384 ) ) ;
#11859=CARTESIAN_POINT ( 'NONE',  ( 42.63976443033212860, 60.99948385550238328, 0.02388180880522514787 ) ) ;
#11869=CARTESIAN_POINT ( 'NONE',  ( 44.05948171654949874, 50.79948385550239465, 4.345558710429104465 ) ) ;
#11870=CARTESIAN_POINT ( 'NONE',  ( 52.25172492374527877, 51.40051614449767214, 7.007379884777203749 ) ) ;
#11872=CARTESIAN_POINT ( 'NONE',  ( 47.70284917648453415, 51.39948385550238896, -6.992620115222774047 ) ) ;
#11876=CARTESIAN_POINT ( 'NONE',  ( 47.37792948025162332, 63.39948385550238896, -7.992620115222770494 ) ) ;
#11885=CARTESIAN_POINT ( 'NONE',  ( 49.97728705011494554, 55.50051614449766646, 6.000000000000000888 ) ) ;
#11886=CARTESIAN_POINT ( 'NONE',  ( 43.33558569842706021, 63.90051614449765793, 2.141517661632167169 ) ) ;
#11887=CARTESIAN_POINT ( 'NONE',  ( 50.02271294988513972, 50.49948385550239749, 8.000000000000001776 ) ) ;
#11888=CARTESIAN_POINT ( 'NONE',  ( 55.94051828345050836, 59.79948385550238754, -4.345558710429104465 ) ) ;
#11890=CARTESIAN_POINT ( 'NONE',  ( 43.20883090819745576, 46.79948385550240886, 4.963592699179006473 ) ) ;
#11902=CARTESIAN_POINT ( 'NONE',  ( 49.97728705011488870, 55.49948385550241170, -6.000000000000000888 ) ) ;
#11903=CARTESIAN_POINT ( 'NONE',  ( 47.70284917648459810, 49.60051614449765367, 6.992620115222797139 ) ) ;
#11904=CARTESIAN_POINT ( 'NONE',  ( 42.39856655714564226, 50.10051614449766078, -2.493737253992044156 ) ) ;
#11907=CARTESIAN_POINT ( 'NONE',  ( 43.34962307344078880, 60.10051614449766078, -2.184720259617096705 ) ) ;
#11918=CARTESIAN_POINT ( 'NONE',  ( 57.36023556966787851, 59.99948385550240459, -0.02388180880522424582 ) ) ;
#11920=CARTESIAN_POINT ( 'NONE',  ( 55.69932041026405045, 61.10051614449766788, 1.875703265242156359 ) ) ;
#11924=CARTESIAN_POINT ( 'NONE',  ( 46.45491332379572924, 47.29948385550241596, -4.840751629271157874 ) ) ;
#11934=AXIS2_PLACEMENT_3D ( 'NONE', #1795, #12244, #10306 ) ;
#11939=CARTESIAN_POINT ( 'NONE',  ( 55.96859303347805081, 54.19948385550240033, 4.306917132069425058 ) ) ;
#11940=CARTESIAN_POINT ( 'NONE',  ( 55.96859303347802239, 54.80051614449764230, -4.306917132069484566 ) ) ;
#11942=CARTESIAN_POINT ( 'NONE',  ( 45.86712807150323812, 53.29948385550240886, -5.649768623646098220 ) ) ;
#11943=CARTESIAN_POINT ( 'NONE',  ( 52.29715082351547295, 46.39948385550240317, 6.992620115222774047 ) ) ;
#11946=CARTESIAN_POINT ( 'NONE',  ( 52.57664461997811856, 61.59948385550240602, -8.007379884777229506 ) ) ;
#11956=CARTESIAN_POINT ( 'NONE',  ( 53.54508667620424234, 54.70051614449765509, -4.840751629271188961 ) ) ;
#11958=CARTESIAN_POINT ( 'NONE',  ( 54.72065718078924590, 54.29948385550241596, 6.458785618021043895 ) ) ;
#11959=CARTESIAN_POINT ( 'NONE',  ( 52.25172492374522903, 55.59948385550241312, -7.007379884777225953 ) ) ;
#11962=CARTESIAN_POINT ( 'NONE',  ( 58.41169779390614281, 63.00051614449766646, 0.02388180880515032231 ) ) ;
#11978=CARTESIAN_POINT ( 'NONE',  ( 44.28664221472220675, 57.09948385550240602, -1.832500667257165317 ) ) ;
#11979=CARTESIAN_POINT ( 'NONE',  ( 43.33558569842706021, 49.90051614449766504, 2.141517661632167169 ) ) ;
#11980=CARTESIAN_POINT ( 'NONE',  ( 56.81924384183006538, 50.80051614449766362, -4.924951120819380357 ) ) ;
#11983=CARTESIAN_POINT ( 'NONE',  ( 51.88965917396063077, 45.00000000000000711, -6.239765512074564313 ) ) ;
#11984=CARTESIAN_POINT ( 'NONE',  ( 54.68390685589039890, 45.30051614449766362, 6.485486291978072693 ) ) ;
#11994=CARTESIAN_POINT ( 'NONE',  ( 54.09612160359786515, 57.69948385550240744, -5.676469297603166098 ) ) ;
#11995=CARTESIAN_POINT ( 'NONE',  ( 48.07319477248762496, 58.40051614449765793, -6.007379884777208190 ) ) ;
#11999=CARTESIAN_POINT ( 'NONE',  ( 55.94051828345053679, 45.20051614449764088, 4.345558710429044069 ) ) ;
#12000=CARTESIAN_POINT ( 'NONE',  ( 55.69932041026404335, 47.89948385550240317, -1.875703265242203432 ) ) ;
#12014=CARTESIAN_POINT ( 'NONE',  ( 44.05948171654945611, 54.20051614449764799, -4.345558710429044069 ) ) ;
#12017=CARTESIAN_POINT ( 'NONE',  ( 43.34962307344081012, 54.89948385550240317, 2.184720259617164650 ) ) ;
#12018=FACE_OUTER_BOUND ( 'NONE', #4402, .T. ) ;
#12019=CARTESIAN_POINT ( 'NONE',  ( 49.97728705011488159, 45.49948385550240459, -7.000000000000000888 ) ) ;
#12030=CARTESIAN_POINT ( 'NONE',  ( 48.02776887271750184, 53.60051614449765367, 5.992620115222795363 ) ) ;
#12033=CARTESIAN_POINT ( 'NONE',  ( 47.42335538002188144, 50.59948385550240602, 8.007379884777233059 ) ) ;
#12035=CARTESIAN_POINT ( 'NONE',  ( 44.03140696652192787, 57.19948385550238612, -4.306917132069425058 ) ) ;
#12037=CARTESIAN_POINT ( 'NONE',  ( 57.61547081786810764, 60.90051614449766504, -2.450534656007114176 ) ) ;
#12047=CARTESIAN_POINT ( 'NONE',  ( 48.02776887271745210, 57.39948385550241028, -5.992620115222778487 ) ) ;
#12048=CARTESIAN_POINT ( 'NONE',  ( 45.90387839640208512, 46.30051614449766362, -5.676469297603124353 ) ) ;
#12049=CARTESIAN_POINT ( 'NONE',  ( 42.38452918213190657, 49.90051614449766504, 2.450534656007115508 ) ) ;
#12051=CARTESIAN_POINT ( 'NONE',  ( 52.95539523038642926, 45.00000000000002132, -5.827023132204991462 ) ) ;
#12053=CARTESIAN_POINT ( 'NONE',  ( 57.61547081786810764, 44.90051614449765793, -2.450534656007114176 ) ) ;
#12061=CARTESIAN_POINT ( 'NONE',  ( 55.96859303347804371, 60.19948385550240744, 4.306917132069425946 ) ) ;
#12063=CARTESIAN_POINT ( 'NONE',  ( 51.97223112728249816, 60.60051614449765367, -5.992620115222793586 ) ) ;
#12066=CARTESIAN_POINT ( 'NONE',  ( 54.09612160359792199, 45.30051614449766362, 5.676469297603124353 ) ) ;
#12067=CARTESIAN_POINT ( 'NONE',  ( 46.49166364869460466, 48.69948385550241454, 4.867452303228209765 ) ) ;
#12078=CARTESIAN_POINT ( 'NONE',  ( 52.29715082351538769, 62.60051614449766078, -6.992620115222796251 ) ) ;
#12081=CARTESIAN_POINT ( 'NONE',  ( 54.13287192849676188, 50.29948385550240175, 5.649768623646098220 ) ) ;
#12082=CARTESIAN_POINT ( 'NONE',  ( 56.66441430157296821, 48.09948385550240602, 2.141517661632100111 ) ) ;
#12083=CARTESIAN_POINT ( 'NONE',  ( 54.72065718078924590, 60.29948385550240175, 6.458785618021043895 ) ) ;
#12091=CARTESIAN_POINT ( 'NONE',  ( 50.02271294988506156, 56.50051614449767357, -6.000000000000000888 ) ) ;
#12092=CARTESIAN_POINT ( 'NONE',  ( 54.09612160359792199, 63.30051614449766362, 5.676469297603124353 ) ) ;
#12093=CARTESIAN_POINT ( 'NONE',  ( 45.31609314410967926, 50.69948385550240744, 6.485486291978119766 ) ) ;
#12094=CARTESIAN_POINT ( 'NONE',  ( 45.86712807150323812, 55.29948385550240175, -5.649768623646098220 ) ) ;
#12097=CARTESIAN_POINT ( 'NONE',  ( 54.68390685589033495, 45.69948385550240033, -6.485486291978119766 ) ) ;
#12103=ORIENTED_EDGE ( 'NONE', *, *, #11649, .T. ) ;
#12111=CARTESIAN_POINT ( 'NONE',  ( 46.45491332379572924, 57.29948385550240175, -4.840751629271157874 ) ) ;
#12112=CARTESIAN_POINT ( 'NONE',  ( 56.65037692655921120, 45.10051614449766078, 2.184720259617097593 ) ) ;
#12113=CARTESIAN_POINT ( 'NONE',  ( 45.27934281921082516, 49.70051614449766220, 6.458785618021089192 ) ) ;
#12115=CARTESIAN_POINT ( 'NONE',  ( 53.45216259278994642, 45.00000000000002132, -5.549029329376620190 ) ) ;
#12116=CARTESIAN_POINT ( 'NONE',  ( 52.25172492374527877, 61.40051614449765083, 7.007379884777203749 ) ) ;
#12125=CARTESIAN_POINT ( 'NONE',  ( 54.13287192849676188, 56.29948385550240175, 5.649768623646098220 ) ) ;
#12127=CARTESIAN_POINT ( 'NONE',  ( 44.28664221472221385, 55.90051614449766504, 1.832500667257213722 ) ) ;
#12129=MECHANICAL_DESIGN_GEOMETRIC_PRESENTATION_REPRESENTATION('',(#8819),#5302);
#12131=CARTESIAN_POINT ( 'NONE',  ( 57.36023556966787851, 45.00051614449763804, 0.02388180880515038476 ) ) ;
#12132=CARTESIAN_POINT ( 'NONE',  ( 50.02271294988512551, 64.49948385550240459, 7.000000000000000888 ) ) ;
#12146=CARTESIAN_POINT ( 'NONE',  ( 45.90387839640208512, 58.30051614449766362, -5.676469297603124353 ) ) ;
#12149=CARTESIAN_POINT ( 'NONE',  ( 55.96859303347804371, 56.19948385550241454, 4.306917132069425946 ) ) ;
#12150=( NAMED_UNIT ( * ) SI_UNIT ( $, .STERADIAN. ) SOLID_ANGLE_UNIT ( ) );
#12151=CARTESIAN_POINT ( 'NONE',  ( 57.60143344285433642, 63.89948385550240317, -2.493737253992118319 ) ) ;
#12161=CARTESIAN_POINT ( 'NONE',  ( 53.50833635130544508, 63.30051614449767072, 4.867452303228181343 ) ) ;
#12164=CARTESIAN_POINT ( 'NONE',  ( 47.42335538002188144, 52.59948385550240602, 8.007379884777233059 ) ) ;
#12165=CARTESIAN_POINT ( 'NONE',  ( 42.63976443033212860, 64.99948385550240459, 0.02388180880522514787 ) ) ;
#12168=CARTESIAN_POINT ( 'NONE',  ( 47.37792948025170858, 63.60051614449764656, 7.992620115222797139 ) ) ;
#12178=CARTESIAN_POINT ( 'NONE',  ( 48.02776887271745210, 63.39948385550238896, -5.992620115222778487 ) ) ;
#12179=CARTESIAN_POINT ( 'NONE',  ( 45.90387839640208512, 50.30051614449766362, -5.676469297603124353 ) ) ;
#12181=CARTESIAN_POINT ( 'NONE',  ( 54.68390685589039890, 53.30051614449767072, 6.485486291978072693 ) ) ;
#12188=CARTESIAN_POINT ( 'NONE',  ( 42.39856655714564226, 46.10051614449766078, -2.493737253992044156 ) ) ;
#12192=DIRECTION ( 'NONE',  ( -1.224646799147353207E-16, 0.000000000000000000, -1.000000000000000000 ) ) ;
#12194=CARTESIAN_POINT ( 'NONE',  ( 43.33558569842703179, 59.09948385550240602, -2.141517661632099223 ) ) ;
#12195=CARTESIAN_POINT ( 'NONE',  ( 52.25172492374522903, 61.59948385550239891, -7.007379884777227730 ) ) ;
#12199=CARTESIAN_POINT ( 'NONE',  ( 52.25172492374527877, 47.40051614449766504, 7.007379884777203749 ) ) ;
#12200=CARTESIAN_POINT ( 'NONE',  ( 55.69932041026404335, 53.89948385550240317, -1.875703265242203432 ) ) ;
#12213=CARTESIAN_POINT ( 'NONE',  ( 55.96859303347802239, 60.80051614449764941, -4.306917132069484566 ) ) ;
#12215=CARTESIAN_POINT ( 'NONE',  ( 49.97728705011488870, 65.49948385550240459, -6.000000000000000888 ) ) ;
#12217=CARTESIAN_POINT ( 'NONE',  ( 43.33558569842703179, 61.09948385550240602, -2.141517661632099223 ) ) ;
#12218=CARTESIAN_POINT ( 'NONE',  ( 43.33558569842703179, 47.09948385550240602, -2.141517661632099223 ) ) ;
#12219=CARTESIAN_POINT ( 'NONE',  ( 43.34962307344081012, 46.89948385550240317, 2.184720259617164650 ) ) ;
#12226=CARTESIAN_POINT ( 'NONE',  ( 55.11794222512599362, 62.80051614449766362, -3.688883143319583446 ) ) ;
#12228=CARTESIAN_POINT ( 'NONE',  ( 52.57664461997811856, 59.59948385550240602, -8.007379884777229506 ) ) ;
#12229=CARTESIAN_POINT ( 'NONE',  ( 47.70284917648453415, 65.39948385550239607, -6.992620115222774047 ) ) ;
#12232=CARTESIAN_POINT ( 'NONE',  ( 56.79116909180255135, 49.79948385550240175, -4.963592699179005585 ) ) ;
#12244=DIRECTION ( 'NONE',  ( 0.9989677110047502362, 0.04542589977017699732, -6.931730960091013400E-15 ) ) ;
#12246=CARTESIAN_POINT ( 'NONE',  ( 43.69122665457040000, 62.99948385550241170, 0.02388180880521036456 ) ) ;
#12247=CARTESIAN_POINT ( 'NONE',  ( 52.25172492374528588, 55.40051614449765083, 7.007379884777204637 ) ) ;
#12249=CARTESIAN_POINT ( 'NONE',  ( 47.42335538002180328, 62.40051614449765793, -8.007379884777206414 ) ) ;
#12252=CARTESIAN_POINT ( 'NONE',  ( 45.31609314410960820, 50.30051614449766362, -6.485486291978072693 ) ) ;
#12261=CARTESIAN_POINT ( 'NONE',  ( 54.13287192849676188, 62.29948385550240886, 5.649768623646098220 ) ) ;
#12262=CARTESIAN_POINT ( 'NONE',  ( 47.70284917648453415, 57.39948385550240317, -6.992620115222774047 ) ) ;
#12267=CARTESIAN_POINT ( 'NONE',  ( 45.90387839640208512, 46.30051614449766362, -5.676469297603124353 ) ) ;
#12268=CARTESIAN_POINT ( 'NONE',  ( 53.54508667620428497, 50.29948385550240886, 4.840751629271157874 ) ) ;
#12279=FACE_OUTER_BOUND ( 'NONE', #1422, .T. ) ;
#12282=CARTESIAN_POINT ( 'NONE',  ( 55.71335778527780747, 64.09948385550239891, 1.832500667257165983 ) ) ;
#12284=CARTESIAN_POINT ( 'NONE',  ( 56.66441430157296821, 56.09948385550240602, 2.141517661632100111 ) ) ;
#12285=CARTESIAN_POINT ( 'NONE',  ( 55.94051828345050836, 53.79948385550238754, -4.345558710429104465 ) ) ;
#12288=CARTESIAN_POINT ( 'NONE',  ( 52.29715082351547295, 46.39948385550240317, 6.992620115222774047 ) ) ;
#12296=CARTESIAN_POINT ( 'NONE',  ( 44.88205777487401349, 61.80051614449766362, 3.688883143319584779 ) ) ;
#12298=CARTESIAN_POINT ( 'NONE',  ( 42.38452918213188525, 59.09948385550240602, -2.450534656007040013 ) ) ;
#12301=CARTESIAN_POINT ( 'NONE',  ( 43.18075615816989199, 51.19948385550240744, -4.924951120819313743 ) ) ;
#12311=CARTESIAN_POINT ( 'NONE',  ( 53.54508667620428497, 62.29948385550241596, 4.840751629271157874 ) ) ;
#12312=CARTESIAN_POINT ( 'NONE',  ( 45.86712807150329496, 51.70051614449766220, 5.649768623646139964 ) ) ;
#12313=CARTESIAN_POINT ( 'NONE',  ( 57.60143344285435774, 61.10051614449766788, 2.493737253992045044 ) ) ;
#12315=CARTESIAN_POINT ( 'NONE',  ( 58.41169779390614281, 53.00051614449765935, 0.02388180880515032231 ) ) ;
#12325=CARTESIAN_POINT ( 'NONE',  ( 51.97223112728254790, 46.39948385550240317, 5.992620115222778487 ) ) ;
#12327=CARTESIAN_POINT ( 'NONE',  ( 52.25172492374522903, 57.59948385550240602, -7.007379884777227730 ) ) ;
#12332=CARTESIAN_POINT ( 'NONE',  ( 47.70284917648459100, 49.60051614449763946, 6.992620115222796251 ) ) ;
#12333=CARTESIAN_POINT ( 'NONE',  ( 55.71335778527780747, 54.09948385550241312, 1.832500667257165983 ) ) ;
#12345=CARTESIAN_POINT ( 'NONE',  ( 42.63976443033212860, 46.99948385550240459, 0.02388180880522514787 ) ) ;
#12350=CARTESIAN_POINT ( 'NONE',  ( 50.02271294988506156, 44.50051614449765935, -6.000000000000000888 ) ) ;
#12353=CARTESIAN_POINT ( 'NONE',  ( 56.65037692655918988, 55.89948385550240317, -2.184720259617163762 ) ) ;
#12354=CARTESIAN_POINT ( 'NONE',  ( 45.90387839640214196, 52.69948385550240033, 5.676469297603166098 ) ) ;
#12357=CARTESIAN_POINT ( 'NONE',  ( 56.65037692655918988, 49.89948385550240317, -2.184720259617163762 ) ) ;
#12365=CARTESIAN_POINT ( 'NONE',  ( 44.30067958973594955, 62.10051614449765367, -1.875703265242155693 ) ) ;
#12367=CARTESIAN_POINT ( 'NONE',  ( 50.02271294988513972, 58.49948385550241170, 8.000000000000001776 ) ) ;
#12369=CARTESIAN_POINT ( 'NONE',  ( 47.70284917648453415, 63.39948385550240317, -6.992620115222774047 ) ) ;
#12371=CARTESIAN_POINT ( 'NONE',  ( 49.97728705011486738, 51.49948385550240459, -8.000000000000001776 ) ) ;
#12381=CARTESIAN_POINT ( 'NONE',  ( 46.45491332379572924, 63.29948385550240175, -4.840751629271157874 ) ) ;
#12382=CARTESIAN_POINT ( 'NONE',  ( 47.74827507625470702, 56.40051614449766504, -7.007379884777204637 ) ) ;
#12383=CARTESIAN_POINT ( 'NONE',  ( 54.72065718078918906, 56.70051614449766930, -6.458785618021089192 ) ) ;
#12387=CARTESIAN_POINT ( 'NONE',  ( 54.68390685589039890, 49.30051614449766362, 6.485486291978072693 ) ) ;
#12396=CARTESIAN_POINT ( 'NONE',  ( 54.09612160359786515, 63.69948385550240744, -5.676469297603166098 ) ) ;
#12397=CARTESIAN_POINT ( 'NONE',  ( 45.86712807150323812, 59.29948385550240175, -5.649768623646098220 ) ) ;
#12401=CARTESIAN_POINT ( 'NONE',  ( 56.65037692655921120, 51.10051614449766078, 2.184720259617097593 ) ) ;
#12402=CARTESIAN_POINT ( 'NONE',  ( 44.88205777487398507, 53.19948385550240744, -3.688883143319540814 ) ) ;
#12413=CARTESIAN_POINT ( 'NONE',  ( 55.94051828345050836, 47.79948385550240886, -4.345558710429104465 ) ) ;
#12417=CARTESIAN_POINT ( 'NONE',  ( 49.97728705011488870, 63.49948385550241170, -6.000000000000000888 ) ) ;
#12419=CARTESIAN_POINT ( 'NONE',  ( 56.65037692655918988, 57.89948385550240317, -2.184720259617163762 ) ) ;
#12420=CARTESIAN_POINT ( 'NONE',  ( 43.33558569842703179, 51.09948385550240602, -2.141517661632099223 ) ) ;
#12422=ORIENTED_EDGE ( 'NONE', *, *, #6451, .F. ) ;
#12423=CARTESIAN_POINT ( 'NONE',  ( 54.09612160359786515, 47.69948385550240744, -5.676469297603166098 ) ) ;
#12431=CARTESIAN_POINT ( 'NONE',  ( 44.88205777487401349, 63.80051614449766362, 3.688883143319584779 ) ) ;
#12433=CARTESIAN_POINT ( 'NONE',  ( 52.62207051974839089, 60.39948385550241028, 7.992620115222770494 ) ) ;
#12435=CARTESIAN_POINT ( 'NONE',  ( 52.62207051974839089, 52.39948385550241028, 7.992620115222770494 ) ) ;
#12446=CARTESIAN_POINT ( 'NONE',  ( 44.91013252490152752, 64.79948385550240175, 3.727524721679198461 ) ) ;
#12448=CARTESIAN_POINT ( 'NONE',  ( 44.03140696652198471, 55.80051614449765651, 4.306917132069485454 ) ) ;
#12450=CARTESIAN_POINT ( 'NONE',  ( 43.18075615816994173, 61.80051614449766362, 4.924951120819380357 ) ) ;
#12452=CARTESIAN_POINT ( 'NONE',  ( 57.61547081786810764, 50.90051614449765793, -2.450534656007114176 ) ) ;
#12465=CARTESIAN_POINT ( 'NONE',  ( 52.29715082351547295, 62.39948385550239607, 6.992620115222774047 ) ) ;
#12466=CARTESIAN_POINT ( 'NONE',  ( 56.66441430157296821, 58.09948385550240602, 2.141517661632100111 ) ) ;
#12467=CARTESIAN_POINT ( 'NONE',  ( 54.13287192849671214, 60.70051614449766220, -5.649768623646139964 ) ) ;
#12473=CARTESIAN_POINT ( 'NONE',  ( 47.70284917648459100, 51.60051614449765367, 6.992620115222796251 ) ) ;
#12474=CARTESIAN_POINT ( 'NONE',  ( 44.28664221472220675, 51.09948385550240602, -1.832500667257165317 ) ) ;
#12487=CARTESIAN_POINT ( 'NONE',  ( 51.97223112728254790, 64.39948385550239607, 5.992620115222778487 ) ) ;
#12489=CARTESIAN_POINT ( 'NONE',  ( 44.03140696652192787, 65.19948385550240744, -4.306917132069425058 ) ) ;
#12490=CARTESIAN_POINT ( 'NONE',  ( 47.70284917648453415, 53.39948385550238186, -6.992620115222774047 ) ) ;
#12492=CARTESIAN_POINT ( 'NONE',  ( 45.86712807150323812, 53.29948385550240886, -5.649768623646098220 ) ) ;
#12499=CARTESIAN_POINT ( 'NONE',  ( 47.74827507625477807, 48.59948385550239891, 7.007379884777229506 ) ) ;
#12501=CARTESIAN_POINT ( 'NONE',  ( 52.25172492374527877, 45.40051614449766504, 7.007379884777203749 ) ) ;
#12503=CARTESIAN_POINT ( 'NONE',  ( 44.03140696652192787, 47.19948385550240744, -4.306917132069425058 ) ) ;
#12507=CARTESIAN_POINT ( 'NONE',  ( 50.02271294988513972, 50.49948385550239749, 8.000000000000001776 ) ) ;
#12509=ORIENTED_EDGE ( 'NONE', *, *, #6451, .T. ) ;
#12513=( LENGTH_UNIT ( ) NAMED_UNIT ( * ) SI_UNIT ( .MILLI., .METRE. ) );
#12517=CARTESIAN_POINT ( 'NONE',  ( 55.71335778527780036, 50.90051614449765793, -1.832500667257213056 ) ) ;
#12518=CARTESIAN_POINT ( 'NONE',  ( 52.29715082351539479, 58.60051614449766078, -6.992620115222796251 ) ) ;
#12520=CARTESIAN_POINT ( 'NONE',  ( 47.37792948025170858, 61.60051614449765367, 7.992620115222797139 ) ) ;
#12524=CARTESIAN_POINT ( 'NONE',  ( 58.41169779390614281, 49.00051614449765935, 0.02388180880515032231 ) ) ;
#12534=CARTESIAN_POINT ( 'NONE',  ( 49.99999999999997158, 65.00000000000002842, -7.000000000000000888 ) ) ;
#12535=CARTESIAN_POINT ( 'NONE',  ( 43.33558569842703179, 61.09948385550240602, -2.141517661632099223 ) ) ;
#12537=CARTESIAN_POINT ( 'NONE',  ( 47.74827507625469281, 62.40051614449766504, -7.007379884777203749 ) ) ;
#12542=( BOUNDED_SURFACE ( )  B_SPLINE_SURFACE ( 3, 2, ( 
 ( #2466, #9933, #1554, #3651, #6703, #6973, #5804, #4692, #11176, #11943, #2673, #4824, #1418, #7936, #2533, #5665, #12218, #4552, #10000, #1696, #8972, #7873, #4760, #6765, #9039, #387, #12082, #4624, #1483, #2602, #3515, #6829, #13170, #3712, #12968, #6902, #10067, #1626, #13237, #8840, #3783, #8007, #2748, #327, #11035, #7739, #10968, #452, #4063, #10211, #4971, #3919, #9320, #5182, #3991, #8216, #12420, #8145, #12561, #2885, #9394, #7036, #646, #792, #4897, #8079, #7250, #10417, #2958, #11246, #9113, #9182, #12354, #6009, #13308, #3853, #10139, #719, #2817, #12490, #13442, #13376, #7107, #12285, #11316, #7183, #1981, #934, #13587, #1838, #6229, #3025, #6088, #4134, #11390, #3093, #10282, #7326, #1767, #5041, #9250, #11536, #1911, #6154, #8356, #2048, #10349, #861, #5111, #13513, #8289, #11456, #7517, #5384, #12628, #12885, #11724, #10624, #3432, #4201, #8621, #10754, #3163, #176, #46, #7389, #4464, #10488, #2244, #7654, #1206, #9591, #6491, #4271, #1261, #11602, #4333, #8425, #7454, #11792, #5453, #1132, #8690, #7585, #9653, #10692, #4394, #11658, #2178, #243, #9521, #113, #8489, #12818, #6426, #11859, #3361, #6296, #8554, #5512, #9452, #1001, #12750, #2315, #5251, #6553, #9723, #2113, #13652, #6361, #10553, #3294, #1064, #5316, #12692, #3232, #13022, #13155, #3565, #501, #7920, #9916, #8756, #4808, #307, #2446, #13219, #1539, #9788, #1398, #12132, #2656, #4535, #5716, #3766, #6685, #7721, #6880, #7788, #564, #8957 ),
 ( #9854, #5787, #11090, #437, #4670, #8894, #373, #9022, #8822, #1605, #12950, #6615, #6750, #10815, #3495, #3697, #5855, #13089, #11924, #1332, #5650, #4604, #10883, #5579, #12000, #2379, #2517, #10953, #4741, #3635, #1469, #7856, #12067, #2586, #6813, #10049, #7988, #11018, #9981, #8270, #838, #703, #4046, #9232, #5168, #3903, #916, #4883, #12268, #3836, #9372, #3970, #1749, #11439, #7236, #13360, #12474, #9093, #11229, #629, #8128, #13428, #11299, #13292, #13572, #8200, #2868, #4117, #10118, #5094, #3008, #8062, #6138, #5994, #2801, #10403, #2729, #12402, #11159, #10195, #4954, #7017, #6953, #1677, #12200, #9167, #12333, #9302, #1822, #7091, #6068, #5920, #10266, #2940, #1963, #6207, #775, #5026, #7164, #13496, #11374, #1893, #10332, #1246, #27, #10736, #983, #8406, #13634, #5496, #92, #11583, #7568, #3346, #9503, #8602, #5235, #7374, #10469, #4250, #9572, #7438, #9436, #9704, #4317, #12672, #230, #6280, #10676, #12803, #4183, #2228, #2097, #12611, #6537, #12545, #8537, #8341, #3277, #11643, #12735, #6343, #11776, #3144, #6409, #10538, #8469, #162, #7500, #3215, #3074, #9638, #11707, #6472, #1184, #2161, #10606, #2297, #1046, #1114, #5299, #5436, #5367, #7308, #4379, #11516, #2033, #11841, #2361, #6598, #4447, #1316, #5562, #10797, #9772, #12869, #8674, #3414, #7637, #11243, #12417, #858, #1692, #9110, #11387, #3849, #12282, #1764, #2955, #12487, #11313, #1835, #6084, #6006, #6227, #10208, #3022, #643, #8004, #8142, #12215 ),
 ( #12350, #2814, #2744, #10279, #716, #5108, #2882, #8285, #4967, #9316, #13305, #789, #3987, #10414, #3780, #1908, #7032, #13510, #5038, #6151, #3916, #6970, #13373, #9179, #13439, #7247, #9247, #10346, #8213, #4060, #11453, #7104, #4894, #8076, #7179, #11173, #1978, #930, #5179, #9389, #5934, #10136, #8353, #2108, #9648, #1256, #7513, #6486, #7449, #3090, #7323, #11596, #12745, #13647, #2311, #1128, #5380, #6550, #9586, #5509, #11654, #8617, #11533, #10750, #2174, #2241, #7581, #5449, #109, #6292, #10687, #172, #11720, #6422, #4328, #1202, #1060, #3159, #10549, #4389, #5312, #12814, #3357, #10620, #10483, #13584, #2045, #4197, #4131, #3290, #997, #12624, #11786, #12558, #5247, #3227, #9448, #8421, #7385, #6357, #9516, #42, #8550, #4267, #8484, #12687, #3427, #10879, #1393, #8751, #2442, #5711, #12880, #11085, #12127, #433, #10949, #13018, #13151, #8817, #4460, #9977, #7650, #5645, #7852, #9851, #8888, #11855, #12947, #5782, #496, #2375, #3559, #1601, #9784, #1327, #4736, #369, #7916, #11995, #8953, #3693, #2652, #6609, #4600, #7784, #3492, #6681, #9912, #10811, #9718, #6876, #4666, #1465, #2512, #240, #6746, #8686, #5575, #302, #13085, #12063, #3629, #4531, #7715, #2582, #11920, #6809, #11014, #1535, #5786, #2516, #9980, #7919, #2728, #3696, #8893, #9915, #3564, #13088, #11089, #5919, #4882, #3835, #436, #10117, #6952, #2585, #628, #1604, #7016, #500, #2800, #6749, #4669, #5715, #11228, #5854, #3634, #13291, #9092 ),
 ( #6812, #8061, #1748, #7987, #11158, #12131, #7787, #11999, #12066, #13218, #7855, #5993, #10048, #563, #372, #4807, #4603, #2655, #12267, #10952, #8821, #6879, #1676, #13021, #1468, #9021, #11017, #1538, #4740, #12199, #3765, #8956, #13154, #11373, #13427, #7163, #7307, #1892, #8340, #2032, #4045, #2867, #12610, #8127, #10265, #7373, #11438, #8199, #5234, #7090, #8269, #12332, #6137, #6279, #5167, #5093, #3143, #11515, #9371, #915, #10402, #10331, #837, #4182, #3969, #13495, #12401, #13571, #9301, #11582, #12544, #12473, #13359, #3007, #1962, #4116, #4953, #3073, #10468, #6206, #982, #11298, #9435, #13633, #8405, #2939, #2096, #10194, #1821, #6067, #702, #774, #5025, #7235, #9166, #3902, #9231, #4378, #161, #91, #8742, #12734, #5561, #3214, #10537, #8601, #3413, #6471, #9501, #1045, #7699, #1183, #5366, #5298, #12802, #3276, #7636, #6342, #10735, #6597, #11840, #11642, #3345, #6536, #12936, #26, #228, #9571, #2360, #7567, #4446, #10675, #4249, #2227, #4316, #2296, #9771, #11775, #12868, #1245, #8673, #1314, #8536, #7437, #2160, #7499, #8468, #11705, #10796, #6408, #5495, #292, #12671, #10605, #5435, #4518, #11907, #3480, #1113, #9703, #9637, #5631, #418, #1590, #2502, #4864, #3683, #7906, #9078, #12116, #8040, #9968, #11142, #9839, #2639, #1524, #8803, #13276, #6865, #6799, #3823, #359, #4794, #6934, #13003, #10035, #9901, #3547, #611, #6668, #11070, #2430, #5836, #5769, #549, #4655, #1660, #7773, #485, #4587, #3619 ),
 ( #7842, #5700, #13075, #13201, #12053, #9004, #7971, #4726, #11984, #10868, #6735, #10937, #1383, #3751, #1454, #8876, #12188, #2709, #2572, #8944, #11000, #13142, #5904, #10102, #13407, #10452, #819, #8321, #11495, #964, #5978, #3953, #8181, #11282, #5004, #8252, #1732, #13618, #5219, #2992, #13476, #1876, #2012, #11353, #7004, #12524, #10313, #9356, #12387, #10179, #11209, #4162, #7146, #1805, #684, #5073, #9216, #13551, #12252, #7216, #3053, #4100, #3885, #9285, #12452, #9421, #2784, #6187, #6050, #7285, #4028, #10382, #2921, #4936, #6118, #10243, #11419, #6262, #1940, #5148, #894, #9148, #13340, #756, #8112, #12315, #2849, #7073, #10586, #2274, #5, #143, #209, #11567, #6454, #6327, #9552, #4429, #3327, #3262, #10780, #9682, #7545, #12784, #8581, #76, #4297, #2343, #11628, #11688, #2143, #11757, #8520, #1299, #6521, #10655, #2079, #2208, #9619, #10719, #3122, #1231, #8652, #4362, #5478, #10518, #12849, #3395, #7617, #6388, #11822, #6581, #1031, #4229, #5543, #8450, #3194, #1096, #9754, #275, #1168, #5416, #8385, #5345, #12592, #12720, #7356, #5279, #9482, #12655, #7422, #7482, #3668, #4775, #6782, #5612, #3463, #3531, #6720, #342, #8725, #9882, #6653, #403, #12037, #6847, #7823, #12985, #4568, #7682, #7755, #1501, #10017, #8989, #7955, #8786, #534, #11052, #10920, #13186, #5750, #11122, #4638, #6917, #10849, #11962, #9823, #1643, #9949, #2484, #3727, #12168, #5682, #2691, #1367, #1433, #8857, #13054, #469, #3600, #2552 ),
 ( #5887, #10982, #12097, #4709, #8929, #10086, #12918, #13126, #4496, #7891, #2618, #1571, #5820, #11890, #2412, #2976, #2833, #6169, #11337, #7268, #6033, #3040, #6986, #663, #5960, #11478, #6105, #3869, #13536, #9339, #1786, #879, #11192, #13321, #2766, #10227, #1856, #13393, #1713, #2000, #10298, #4990, #6245, #12232, #7201, #5129, #10158, #8237, #8096, #4917, #12507, #4844, #806, #593, #9270, #3937, #5057, #12301, #4083, #9130, #12371, #7056, #737, #10369, #13461, #9200, #9058, #1925, #4010, #12435, #11406, #8166, #2904, #8306, #11267, #7128, #13254, #3802, #8023, #12839, #8569, #12707, #13605, #64, #11673, #9609, #5204, #130, #2262, #2196, #5402, #12576, #12771, #4352, #6439, #4216, #3314, #7535, #8371, #2066, #11743, #10504, #5266, #8437, #6508, #5468, #4284, #8507, #3250, #12644, #3381, #3178, #9671, #7340, #949, #10710, #1221, #10569, #196, #4418, #7470, #11552, #9407, #9466, #7408, #6313, #4147, #2131, #3111, #6374, #10643, #8637, #1154, #6418, #1017, #11616, #1078, #7602, #11810, #2331, #10439, #5333, #9537, #9743, #8974, #388, #8912, #519, #12083, #2535, #12906, #13110, #6831, #4693, #4625, #10969, #3652, #7740, #9806, #3516, #7875, #11946, #2604, #11037, #8842, #3448, #13171, #4484, #6638, #3713, #5734, #259, #5598, #1556, #5806, #8706, #9869, #7938, #10835, #11876, #10001, #2468, #4762, #13040, #12151, #6570, #10768, #7671, #6705, #10899, #329, #12970, #6767, #2398, #1284, #5530, #1485, #7808, #3584, #1354, #5667 ),
 ( #12019, #4554, #8773, #1420, #9934, #455, #6903, #8081, #4826, #12288, #10215, #5043, #6013, #11178, #12219, #5873, #1698, #13378, #8220, #7187, #6156, #2750, #12423, #9253, #4900, #2960, #3921, #9326, #2819, #5114, #9041, #6974, #8009, #13517, #8149, #5941, #1913, #11392, #3855, #10352, #13239, #10140, #3785, #7040, #12357, #1769, #647, #4065, #2888, #11249, #8291, #578, #13445, #863, #9115, #10284, #13309, #721, #2676, #11108, #7111, #1627, #11318, #4974, #9184, #10070, #1841, #6091, #794, #3994, #9396, #3027, #6231, #4136, #7253, #11459, #13590, #1984, #12492, #10423, #938, #5184, #531, #5541, #12983, #3529, #10847, #4565, #7820, #1297, #13184, #4773, #2550, #13052, #1431, #1569, #10917, #6579, #12094, #9879, #8925, #11959, #9752, #10778, #3724, #6717, #1365, #273, #401, #8784, #13124, #11819, #6779, #2616, #3666, #3461, #8855, #12035, #8987, #2341, #5748, #5610, #7889, #4636, #9947, #2482, #4494, #7753, #9820, #10980, #5818, #5679, #4707, #1498, #467, #6844, #339, #8720, #12915, #3597, #7680, #11050, #10014, #11888, #2410, #6651, #11119, #2689, #10156, #4200, #9520, #1853, #1000, #1784, #1641, #5884, #5957, #7126, #8021, #10552, #9198, #13391, #1063, #3935, #45, #6029, #3162, #10084, #5315, #10225, #10296, #2112, #13651, #8163, #591, #5250, #8424, #6103, #734, #12369, #9451, #9127, #11189, #4915, #12627, #13319, #7388, #11601, #4988, #4841, #7953, #9055, #6360, #2902, #13252, #12165, #6915, #3799, #11332, #12229, #2763 ) ),
 .UNSPECIFIED., .T., .F., .T. ) 
 B_SPLINE_SURFACE_WITH_KNOTS ( ( 4, 3, 4 ),
 ( 3, 2, 2, 2, 2, 2, 2, 2, 2, 2, 2, 2, 2, 2, 2, 2, 2, 2, 2, 2, 2, 2, 2, 2, 2, 2, 2, 2, 2, 2, 2, 2, 2, 2, 2, 2, 2, 2, 2, 2, 2, 2, 2, 2, 2, 2, 2, 2, 2, 2, 2, 2, 2, 2, 2, 2, 2, 2, 2, 2, 2, 2, 2, 2, 2, 2, 2, 2, 2, 2, 2, 2, 2, 2, 2, 2, 2, 2, 2, 2, 2, 2, 2, 2, 2, 2, 2, 2, 2, 2, 2, 2, 2, 2, 2, 2, 2, 2, 2, 2, 3 ),
 ( 0.000000000000000000, 0.5000000000000000000, 1.000000000000000000 ),
 ( 0.000000000000000000, 0.01000000000000000021, 0.02000000000000000042, 0.02999999999999999889, 0.04000000000000000083, 0.05000000000000000278, 0.05999999999999999778, 0.07000000000000000666, 0.08000000000000000167, 0.08999999999999999667, 0.1000000000000000056, 0.1100000000000000006, 0.1199999999999999956, 0.1300000000000000044, 0.1400000000000000133, 0.1499999999999999944, 0.1600000000000000033, 0.1700000000000000122, 0.1799999999999999933, 0.1900000000000000022, 0.2000000000000000111, 0.2099999999999999922, 0.2200000000000000011, 0.2300000000000000100, 0.2399999999999999911, 0.2500000000000000000, 0.2600000000000000089, 0.2700000000000000178, 0.2800000000000000266, 0.2899999999999999800, 0.2999999999999999889, 0.3099999999999999978, 0.3200000000000000067, 0.3300000000000000155, 0.3400000000000000244, 0.3499999999999999778, 0.3599999999999999867, 0.3699999999999999956, 0.3800000000000000044, 0.3900000000000000133, 0.4000000000000000222, 0.4099999999999999756, 0.4199999999999999845, 0.4299999999999999933, 0.4400000000000000022, 0.4500000000000000111, 0.4600000000000000200, 0.4699999999999999734, 0.4799999999999999822, 0.4899999999999999911, 0.5000000000000000000, 0.5100000000000000089, 0.5200000000000000178, 0.5300000000000000266, 0.5400000000000000355, 0.5500000000000000444, 0.5600000000000000533, 0.5699999999999999512, 0.5799999999999999600, 0.5899999999999999689, 0.5999999999999999778, 0.6099999999999999867, 0.6199999999999999956, 0.6300000000000000044, 0.6400000000000000133, 0.6500000000000000222, 0.6600000000000000311, 0.6700000000000000400, 0.6800000000000000488, 0.6899999999999999467, 0.6999999999999999556, 0.7099999999999999645, 0.7199999999999999734, 0.7299999999999999822, 0.7399999999999999911, 0.7500000000000000000, 0.7600000000000000089, 0.7700000000000000178, 0.7800000000000000266, 0.7900000000000000355, 0.8000000000000000444, 0.8100000000000000533, 0.8199999999999999512, 0.8299999999999999600, 0.8399999999999999689, 0.8499999999999999778, 0.8599999999999999867, 0.8699999999999999956, 0.8800000000000000044, 0.8900000000000000133, 0.9000000000000000222, 0.9100000000000000311, 0.9200000000000000400, 0.9300000000000000488, 0.9399999999999999467, 0.9499999999999999556, 0.9599999999999999645, 0.9699999999999999734, 0.9799999999999999822, 0.9899999999999999911, 1.000000000000000000 ),
 .UNSPECIFIED. ) 
 GEOMETRIC_REPRESENTATION_ITEM ( )  RATIONAL_B_SPLINE_SURFACE ( (
 ( 1.000000000000000000, 0.9510565162951535312, 1.000000000000000000, 0.9510565162951535312, 1.000000000000000000, 0.9510565162951535312, 1.000000000000000000, 0.9510565162951535312, 1.000000000000000000, 0.9510565162951535312, 1.000000000000000000, 0.9510565162951535312, 1.000000000000000000, 0.9510565162951535312, 1.000000000000000000, 0.9510565162951535312, 1.000000000000000000, 0.9510565162951535312, 1.000000000000000000, 0.9510565162951535312, 1.000000000000000000, 0.9510565162951535312, 1.000000000000000000, 0.9510565162951535312, 1.000000000000000000, 0.9510565162951535312, 1.000000000000000000, 0.9510565162951535312, 1.000000000000000000, 0.9510565162951535312, 1.000000000000000000, 0.9510565162951535312, 1.000000000000000000, 0.9510565162951535312, 1.000000000000000000, 0.9510565162951535312, 1.000000000000000000, 0.9510565162951535312, 1.000000000000000000, 0.9510565162951535312, 1.000000000000000000, 0.9510565162951535312, 1.000000000000000000, 0.9510565162951535312, 1.000000000000000000, 0.9510565162951535312, 1.000000000000000000, 0.9510565162951535312, 1.000000000000000000, 0.9510565162951535312, 1.000000000000000000, 0.9510565162951535312, 1.000000000000000000, 0.9510565162951535312, 1.000000000000000000, 0.9510565162951535312, 1.000000000000000000, 0.9510565162951535312, 1.000000000000000000, 0.9510565162951535312, 1.000000000000000000, 0.9510565162951535312, 1.000000000000000000, 0.9510565162951535312, 1.000000000000000000, 0.9510565162951535312, 1.000000000000000000, 0.9510565162951535312, 1.000000000000000000, 0.9510565162951535312, 1.000000000000000000, 0.9510565162951535312, 1.000000000000000000, 0.9510565162951535312, 1.000000000000000000, 0.9510565162951535312, 1.000000000000000000, 0.9510565162951535312, 1.000000000000000000, 0.9510565162951535312, 1.000000000000000000, 0.9510565162951535312, 1.000000000000000000, 0.9510565162951535312, 1.000000000000000000, 0.9510565162951535312, 1.000000000000000000, 0.9510565162951535312, 1.000000000000000000, 0.9510565162951535312, 1.000000000000000000, 0.9510565162951535312, 1.000000000000000000, 0.9510565162951535312, 1.000000000000000000, 0.9510565162951535312, 1.000000000000000000, 0.9510565162951535312, 1.000000000000000000, 0.9510565162951535312, 1.000000000000000000, 0.9510565162951535312, 1.000000000000000000, 0.9510565162951535312, 1.000000000000000000, 0.9510565162951535312, 1.000000000000000000, 0.9510565162951535312, 1.000000000000000000, 0.9510565162951535312, 1.000000000000000000, 0.9510565162951535312, 1.000000000000000000, 0.9510565162951535312, 1.000000000000000000, 0.9510565162951535312, 1.000000000000000000, 0.9510565162951535312, 1.000000000000000000, 0.9510565162951535312, 1.000000000000000000, 0.9510565162951535312, 1.000000000000000000, 0.9510565162951535312, 1.000000000000000000, 0.9510565162951535312, 1.000000000000000000, 0.9510565162951535312, 1.000000000000000000, 0.9510565162951535312, 1.000000000000000000, 0.9510565162951535312, 1.000000000000000000, 0.9510565162951535312, 1.000000000000000000, 0.9510565162951535312, 1.000000000000000000, 0.9510565162951535312, 1.000000000000000000, 0.9510565162951535312, 1.000000000000000000, 0.9510565162951535312, 1.000000000000000000, 0.9510565162951535312, 1.000000000000000000, 0.9510565162951535312, 1.000000000000000000, 0.9510565162951535312, 1.000000000000000000, 0.9510565162951535312, 1.000000000000000000, 0.9510565162951535312, 1.000000000000000000, 0.9510565162951535312, 1.000000000000000000, 0.9510565162951535312, 1.000000000000000000, 0.9510565162951535312, 1.000000000000000000, 0.9510565162951535312, 1.000000000000000000, 0.9510565162951535312, 1.000000000000000000, 0.9510565162951535312, 1.000000000000000000, 0.9510565162951535312, 1.000000000000000000, 0.9510565162951535312, 1.000000000000000000, 0.9510565162951535312, 1.000000000000000000, 0.9510565162951535312, 1.000000000000000000, 0.9510565162951535312, 1.000000000000000000, 0.9510565162951535312, 1.000000000000000000, 0.9510565162951535312, 1.000000000000000000, 0.9510565162951535312, 1.000000000000000000, 0.9510565162951535312, 1.000000000000000000, 0.9510565162951535312, 1.000000000000000000, 0.9510565162951535312, 1.000000000000000000, 0.9510565162951535312, 1.000000000000000000, 0.9510565162951535312, 1.000000000000000000, 0.9510565162951535312, 1.000000000000000000, 0.9510565162951535312, 1.000000000000000000, 0.9510565162951535312, 1.000000000000000000, 0.9510565162951535312, 1.000000000000000000, 0.9510565162951535312, 1.000000000000000000),
 ( 0.3333333333333333703, 0.3170188387650512141, 0.3333333333333333703, 0.3170188387650512141, 0.3333333333333333703, 0.3170188387650512141, 0.3333333333333333703, 0.3170188387650512141, 0.3333333333333333703, 0.3170188387650512141, 0.3333333333333333703, 0.3170188387650512141, 0.3333333333333333703, 0.3170188387650512141, 0.3333333333333333703, 0.3170188387650512141, 0.3333333333333333703, 0.3170188387650512141, 0.3333333333333333703, 0.3170188387650512141, 0.3333333333333333703, 0.3170188387650512141, 0.3333333333333333703, 0.3170188387650512141, 0.3333333333333333703, 0.3170188387650512141, 0.3333333333333333703, 0.3170188387650512141, 0.3333333333333333703, 0.3170188387650512141, 0.3333333333333333703, 0.3170188387650512141, 0.3333333333333333703, 0.3170188387650512141, 0.3333333333333333703, 0.3170188387650512141, 0.3333333333333333703, 0.3170188387650512141, 0.3333333333333333703, 0.3170188387650512141, 0.3333333333333333703, 0.3170188387650512141, 0.3333333333333333703, 0.3170188387650512141, 0.3333333333333333703, 0.3170188387650512141, 0.3333333333333333703, 0.3170188387650512141, 0.3333333333333333703, 0.3170188387650512141, 0.3333333333333333703, 0.3170188387650512141, 0.3333333333333333703, 0.3170188387650512141, 0.3333333333333333703, 0.3170188387650512141, 0.3333333333333333703, 0.3170188387650512141, 0.3333333333333333703, 0.3170188387650512141, 0.3333333333333333703, 0.3170188387650512141, 0.3333333333333333703, 0.3170188387650512141, 0.3333333333333333703, 0.3170188387650512141, 0.3333333333333333703, 0.3170188387650512141, 0.3333333333333333703, 0.3170188387650512141, 0.3333333333333333703, 0.3170188387650512141, 0.3333333333333333703, 0.3170188387650512141, 0.3333333333333333703, 0.3170188387650512141, 0.3333333333333333703, 0.3170188387650512141, 0.3333333333333333703, 0.3170188387650512141, 0.3333333333333333703, 0.3170188387650512141, 0.3333333333333333703, 0.3170188387650512141, 0.3333333333333333703, 0.3170188387650512141, 0.3333333333333333703, 0.3170188387650512141, 0.3333333333333333703, 0.3170188387650512141, 0.3333333333333333703, 0.3170188387650512141, 0.3333333333333333703, 0.3170188387650512141, 0.3333333333333333703, 0.3170188387650512141, 0.3333333333333333703, 0.3170188387650512141, 0.3333333333333333703, 0.3170188387650512141, 0.3333333333333333703, 0.3170188387650512141, 0.3333333333333333703, 0.3170188387650512141, 0.3333333333333333703, 0.3170188387650512141, 0.3333333333333333703, 0.3170188387650512141, 0.3333333333333333703, 0.3170188387650512141, 0.3333333333333333703, 0.3170188387650512141, 0.3333333333333333703, 0.3170188387650512141, 0.3333333333333333703, 0.3170188387650512141, 0.3333333333333333703, 0.3170188387650512141, 0.3333333333333333703, 0.3170188387650512141, 0.3333333333333333703, 0.3170188387650512141, 0.3333333333333333703, 0.3170188387650512141, 0.3333333333333333703, 0.3170188387650512141, 0.3333333333333333703, 0.3170188387650512141, 0.3333333333333333703, 0.3170188387650512141, 0.3333333333333333703, 0.3170188387650512141, 0.3333333333333333703, 0.3170188387650512141, 0.3333333333333333703, 0.3170188387650512141, 0.3333333333333333703, 0.3170188387650512141, 0.3333333333333333703, 0.3170188387650512141, 0.3333333333333333703, 0.3170188387650512141, 0.3333333333333333703, 0.3170188387650512141, 0.3333333333333333703, 0.3170188387650512141, 0.3333333333333333703, 0.3170188387650512141, 0.3333333333333333703, 0.3170188387650512141, 0.3333333333333333703, 0.3170188387650512141, 0.3333333333333333703, 0.3170188387650512141, 0.3333333333333333703, 0.3170188387650512141, 0.3333333333333333703, 0.3170188387650512141, 0.3333333333333333703, 0.3170188387650512141, 0.3333333333333333703, 0.3170188387650512141, 0.3333333333333333703, 0.3170188387650512141, 0.3333333333333333703, 0.3170188387650512141, 0.3333333333333333703, 0.3170188387650512141, 0.3333333333333333703, 0.3170188387650512141, 0.3333333333333333703, 0.3170188387650512141, 0.3333333333333333703, 0.3170188387650512141, 0.3333333333333333703, 0.3170188387650512141, 0.3333333333333333703, 0.3170188387650512141, 0.3333333333333333703, 0.3170188387650512141, 0.3333333333333333703, 0.3170188387650512141, 0.3333333333333333703, 0.3170188387650512141, 0.3333333333333333703, 0.3170188387650512141, 0.3333333333333333703, 0.3170188387650512141, 0.3333333333333333703, 0.3170188387650512141, 0.3333333333333333703, 0.3170188387650512141, 0.3333333333333333703, 0.3170188387650512141, 0.3333333333333333703, 0.3170188387650512141, 0.3333333333333333703, 0.3170188387650512141, 0.3333333333333333703, 0.3170188387650512141, 0.3333333333333333703),
 ( 0.3333333333333333703, 0.3170188387650512141, 0.3333333333333333703, 0.3170188387650512141, 0.3333333333333333703, 0.3170188387650512141, 0.3333333333333333703, 0.3170188387650512141, 0.3333333333333333703, 0.3170188387650512141, 0.3333333333333333703, 0.3170188387650512141, 0.3333333333333333703, 0.3170188387650512141, 0.3333333333333333703, 0.3170188387650512141, 0.3333333333333333703, 0.3170188387650512141, 0.3333333333333333703, 0.3170188387650512141, 0.3333333333333333703, 0.3170188387650512141, 0.3333333333333333703, 0.3170188387650512141, 0.3333333333333333703, 0.3170188387650512141, 0.3333333333333333703, 0.3170188387650512141, 0.3333333333333333703, 0.3170188387650512141, 0.3333333333333333703, 0.3170188387650512141, 0.3333333333333333703, 0.3170188387650512141, 0.3333333333333333703, 0.3170188387650512141, 0.3333333333333333703, 0.3170188387650512141, 0.3333333333333333703, 0.3170188387650512141, 0.3333333333333333703, 0.3170188387650512141, 0.3333333333333333703, 0.3170188387650512141, 0.3333333333333333703, 0.3170188387650512141, 0.3333333333333333703, 0.3170188387650512141, 0.3333333333333333703, 0.3170188387650512141, 0.3333333333333333703, 0.3170188387650512141, 0.3333333333333333703, 0.3170188387650512141, 0.3333333333333333703, 0.3170188387650512141, 0.3333333333333333703, 0.3170188387650512141, 0.3333333333333333703, 0.3170188387650512141, 0.3333333333333333703, 0.3170188387650512141, 0.3333333333333333703, 0.3170188387650512141, 0.3333333333333333703, 0.3170188387650512141, 0.3333333333333333703, 0.3170188387650512141, 0.3333333333333333703, 0.3170188387650512141, 0.3333333333333333703, 0.3170188387650512141, 0.3333333333333333703, 0.3170188387650512141, 0.3333333333333333703, 0.3170188387650512141, 0.3333333333333333703, 0.3170188387650512141, 0.3333333333333333703, 0.3170188387650512141, 0.3333333333333333703, 0.3170188387650512141, 0.3333333333333333703, 0.3170188387650512141, 0.3333333333333333703, 0.3170188387650512141, 0.3333333333333333703, 0.3170188387650512141, 0.3333333333333333703, 0.3170188387650512141, 0.3333333333333333703, 0.3170188387650512141, 0.3333333333333333703, 0.3170188387650512141, 0.3333333333333333703, 0.3170188387650512141, 0.3333333333333333703, 0.3170188387650512141, 0.3333333333333333703, 0.3170188387650512141, 0.3333333333333333703, 0.3170188387650512141, 0.3333333333333333703, 0.3170188387650512141, 0.3333333333333333703, 0.3170188387650512141, 0.3333333333333333703, 0.3170188387650512141, 0.3333333333333333703, 0.3170188387650512141, 0.3333333333333333703, 0.3170188387650512141, 0.3333333333333333703, 0.3170188387650512141, 0.3333333333333333703, 0.3170188387650512141, 0.3333333333333333703, 0.3170188387650512141, 0.3333333333333333703, 0.3170188387650512141, 0.3333333333333333703, 0.3170188387650512141, 0.3333333333333333703, 0.3170188387650512141, 0.3333333333333333703, 0.3170188387650512141, 0.3333333333333333703, 0.3170188387650512141, 0.3333333333333333703, 0.3170188387650512141, 0.3333333333333333703, 0.3170188387650512141, 0.3333333333333333703, 0.3170188387650512141, 0.3333333333333333703, 0.3170188387650512141, 0.3333333333333333703, 0.3170188387650512141, 0.3333333333333333703, 0.3170188387650512141, 0.3333333333333333703, 0.3170188387650512141, 0.3333333333333333703, 0.3170188387650512141, 0.3333333333333333703, 0.3170188387650512141, 0.3333333333333333703, 0.3170188387650512141, 0.3333333333333333703, 0.3170188387650512141, 0.3333333333333333703, 0.3170188387650512141, 0.3333333333333333703, 0.3170188387650512141, 0.3333333333333333703, 0.3170188387650512141, 0.3333333333333333703, 0.3170188387650512141, 0.3333333333333333703, 0.3170188387650512141, 0.3333333333333333703, 0.3170188387650512141, 0.3333333333333333703, 0.3170188387650512141, 0.3333333333333333703, 0.3170188387650512141, 0.3333333333333333703, 0.3170188387650512141, 0.3333333333333333703, 0.3170188387650512141, 0.3333333333333333703, 0.3170188387650512141, 0.3333333333333333703, 0.3170188387650512141, 0.3333333333333333703, 0.3170188387650512141, 0.3333333333333333703, 0.3170188387650512141, 0.3333333333333333703, 0.3170188387650512141, 0.3333333333333333703, 0.3170188387650512141, 0.3333333333333333703, 0.3170188387650512141, 0.3333333333333333703, 0.3170188387650512141, 0.3333333333333333703, 0.3170188387650512141, 0.3333333333333333703, 0.3170188387650512141, 0.3333333333333333703, 0.3170188387650512141, 0.3333333333333333703, 0.3170188387650512141, 0.3333333333333333703, 0.3170188387650512141, 0.3333333333333333703, 0.3170188387650512141, 0.3333333333333333703, 0.3170188387650512141, 0.3333333333333333703),
 ( 1.000000000000000000, 0.9510565162951535312, 1.000000000000000000, 0.9510565162951535312, 1.000000000000000000, 0.9510565162951535312, 1.000000000000000000, 0.9510565162951535312, 1.000000000000000000, 0.9510565162951535312, 1.000000000000000000, 0.9510565162951535312, 1.000000000000000000, 0.9510565162951535312, 1.000000000000000000, 0.9510565162951535312, 1.000000000000000000, 0.9510565162951535312, 1.000000000000000000, 0.9510565162951535312, 1.000000000000000000, 0.9510565162951535312, 1.000000000000000000, 0.9510565162951535312, 1.000000000000000000, 0.9510565162951535312, 1.000000000000000000, 0.9510565162951535312, 1.000000000000000000, 0.9510565162951535312, 1.000000000000000000, 0.9510565162951535312, 1.000000000000000000, 0.9510565162951535312, 1.000000000000000000, 0.9510565162951535312, 1.000000000000000000, 0.9510565162951535312, 1.000000000000000000, 0.9510565162951535312, 1.000000000000000000, 0.9510565162951535312, 1.000000000000000000, 0.9510565162951535312, 1.000000000000000000, 0.9510565162951535312, 1.000000000000000000, 0.9510565162951535312, 1.000000000000000000, 0.9510565162951535312, 1.000000000000000000, 0.9510565162951535312, 1.000000000000000000, 0.9510565162951535312, 1.000000000000000000, 0.9510565162951535312, 1.000000000000000000, 0.9510565162951535312, 1.000000000000000000, 0.9510565162951535312, 1.000000000000000000, 0.9510565162951535312, 1.000000000000000000, 0.9510565162951535312, 1.000000000000000000, 0.9510565162951535312, 1.000000000000000000, 0.9510565162951535312, 1.000000000000000000, 0.9510565162951535312, 1.000000000000000000, 0.9510565162951535312, 1.000000000000000000, 0.9510565162951535312, 1.000000000000000000, 0.9510565162951535312, 1.000000000000000000, 0.9510565162951535312, 1.000000000000000000, 0.9510565162951535312, 1.000000000000000000, 0.9510565162951535312, 1.000000000000000000, 0.9510565162951535312, 1.000000000000000000, 0.9510565162951535312, 1.000000000000000000, 0.9510565162951535312, 1.000000000000000000, 0.9510565162951535312, 1.000000000000000000, 0.9510565162951535312, 1.000000000000000000, 0.9510565162951535312, 1.000000000000000000, 0.9510565162951535312, 1.000000000000000000, 0.9510565162951535312, 1.000000000000000000, 0.9510565162951535312, 1.000000000000000000, 0.9510565162951535312, 1.000000000000000000, 0.9510565162951535312, 1.000000000000000000, 0.9510565162951535312, 1.000000000000000000, 0.9510565162951535312, 1.000000000000000000, 0.9510565162951535312, 1.000000000000000000, 0.9510565162951535312, 1.000000000000000000, 0.9510565162951535312, 1.000000000000000000, 0.9510565162951535312, 1.000000000000000000, 0.9510565162951535312, 1.000000000000000000, 0.9510565162951535312, 1.000000000000000000, 0.9510565162951535312, 1.000000000000000000, 0.9510565162951535312, 1.000000000000000000, 0.9510565162951535312, 1.000000000000000000, 0.9510565162951535312, 1.000000000000000000, 0.9510565162951535312, 1.000000000000000000, 0.9510565162951535312, 1.000000000000000000, 0.9510565162951535312, 1.000000000000000000, 0.9510565162951535312, 1.000000000000000000, 0.9510565162951535312, 1.000000000000000000, 0.9510565162951535312, 1.000000000000000000, 0.9510565162951535312, 1.000000000000000000, 0.9510565162951535312, 1.000000000000000000, 0.9510565162951535312, 1.000000000000000000, 0.9510565162951535312, 1.000000000000000000, 0.9510565162951535312, 1.000000000000000000, 0.9510565162951535312, 1.000000000000000000, 0.9510565162951535312, 1.000000000000000000, 0.9510565162951535312, 1.000000000000000000, 0.9510565162951535312, 1.000000000000000000, 0.9510565162951535312, 1.000000000000000000, 0.9510565162951535312, 1.000000000000000000, 0.9510565162951535312, 1.000000000000000000, 0.9510565162951535312, 1.000000000000000000, 0.9510565162951535312, 1.000000000000000000, 0.9510565162951535312, 1.000000000000000000, 0.9510565162951535312, 1.000000000000000000, 0.9510565162951535312, 1.000000000000000000, 0.9510565162951535312, 1.000000000000000000, 0.9510565162951535312, 1.000000000000000000, 0.9510565162951535312, 1.000000000000000000, 0.9510565162951535312, 1.000000000000000000, 0.9510565162951535312, 1.000000000000000000, 0.9510565162951535312, 1.000000000000000000, 0.9510565162951535312, 1.000000000000000000, 0.9510565162951535312, 1.000000000000000000, 0.9510565162951535312, 1.000000000000000000, 0.9510565162951535312, 1.000000000000000000, 0.9510565162951535312, 1.000000000000000000, 0.9510565162951535312, 1.000000000000000000, 0.9510565162951535312, 1.000000000000000000),
 ( 0.3333333333333333703, 0.3170188387650512141, 0.3333333333333333703, 0.3170188387650512141, 0.3333333333333333703, 0.3170188387650512141, 0.3333333333333333703, 0.3170188387650512141, 0.3333333333333333703, 0.3170188387650512141, 0.3333333333333333703, 0.3170188387650512141, 0.3333333333333333703, 0.3170188387650512141, 0.3333333333333333703, 0.3170188387650512141, 0.3333333333333333703, 0.3170188387650512141, 0.3333333333333333703, 0.3170188387650512141, 0.3333333333333333703, 0.3170188387650512141, 0.3333333333333333703, 0.3170188387650512141, 0.3333333333333333703, 0.3170188387650512141, 0.3333333333333333703, 0.3170188387650512141, 0.3333333333333333703, 0.3170188387650512141, 0.3333333333333333703, 0.3170188387650512141, 0.3333333333333333703, 0.3170188387650512141, 0.3333333333333333703, 0.3170188387650512141, 0.3333333333333333703, 0.3170188387650512141, 0.3333333333333333703, 0.3170188387650512141, 0.3333333333333333703, 0.3170188387650512141, 0.3333333333333333703, 0.3170188387650512141, 0.3333333333333333703, 0.3170188387650512141, 0.3333333333333333703, 0.3170188387650512141, 0.3333333333333333703, 0.3170188387650512141, 0.3333333333333333703, 0.3170188387650512141, 0.3333333333333333703, 0.3170188387650512141, 0.3333333333333333703, 0.3170188387650512141, 0.3333333333333333703, 0.3170188387650512141, 0.3333333333333333703, 0.3170188387650512141, 0.3333333333333333703, 0.3170188387650512141, 0.3333333333333333703, 0.3170188387650512141, 0.3333333333333333703, 0.3170188387650512141, 0.3333333333333333703, 0.3170188387650512141, 0.3333333333333333703, 0.3170188387650512141, 0.3333333333333333703, 0.3170188387650512141, 0.3333333333333333703, 0.3170188387650512141, 0.3333333333333333703, 0.3170188387650512141, 0.3333333333333333703, 0.3170188387650512141, 0.3333333333333333703, 0.3170188387650512141, 0.3333333333333333703, 0.3170188387650512141, 0.3333333333333333703, 0.3170188387650512141, 0.3333333333333333703, 0.3170188387650512141, 0.3333333333333333703, 0.3170188387650512141, 0.3333333333333333703, 0.3170188387650512141, 0.3333333333333333703, 0.3170188387650512141, 0.3333333333333333703, 0.3170188387650512141, 0.3333333333333333703, 0.3170188387650512141, 0.3333333333333333703, 0.3170188387650512141, 0.3333333333333333703, 0.3170188387650512141, 0.3333333333333333703, 0.3170188387650512141, 0.3333333333333333703, 0.3170188387650512141, 0.3333333333333333703, 0.3170188387650512141, 0.3333333333333333703, 0.3170188387650512141, 0.3333333333333333703, 0.3170188387650512141, 0.3333333333333333703, 0.3170188387650512141, 0.3333333333333333703, 0.3170188387650512141, 0.3333333333333333703, 0.3170188387650512141, 0.3333333333333333703, 0.3170188387650512141, 0.3333333333333333703, 0.3170188387650512141, 0.3333333333333333703, 0.3170188387650512141, 0.3333333333333333703, 0.3170188387650512141, 0.3333333333333333703, 0.3170188387650512141, 0.3333333333333333703, 0.3170188387650512141, 0.3333333333333333703, 0.3170188387650512141, 0.3333333333333333703, 0.3170188387650512141, 0.3333333333333333703, 0.3170188387650512141, 0.3333333333333333703, 0.3170188387650512141, 0.3333333333333333703, 0.3170188387650512141, 0.3333333333333333703, 0.3170188387650512141, 0.3333333333333333703, 0.3170188387650512141, 0.3333333333333333703, 0.3170188387650512141, 0.3333333333333333703, 0.3170188387650512141, 0.3333333333333333703, 0.3170188387650512141, 0.3333333333333333703, 0.3170188387650512141, 0.3333333333333333703, 0.3170188387650512141, 0.3333333333333333703, 0.3170188387650512141, 0.3333333333333333703, 0.3170188387650512141, 0.3333333333333333703, 0.3170188387650512141, 0.3333333333333333703, 0.3170188387650512141, 0.3333333333333333703, 0.3170188387650512141, 0.3333333333333333703, 0.3170188387650512141, 0.3333333333333333703, 0.3170188387650512141, 0.3333333333333333703, 0.3170188387650512141, 0.3333333333333333703, 0.3170188387650512141, 0.3333333333333333703, 0.3170188387650512141, 0.3333333333333333703, 0.3170188387650512141, 0.3333333333333333703, 0.3170188387650512141, 0.3333333333333333703, 0.3170188387650512141, 0.3333333333333333703, 0.3170188387650512141, 0.3333333333333333703, 0.3170188387650512141, 0.3333333333333333703, 0.3170188387650512141, 0.3333333333333333703, 0.3170188387650512141, 0.3333333333333333703, 0.3170188387650512141, 0.3333333333333333703, 0.3170188387650512141, 0.3333333333333333703, 0.3170188387650512141, 0.3333333333333333703, 0.3170188387650512141, 0.3333333333333333703, 0.3170188387650512141, 0.3333333333333333703, 0.3170188387650512141, 0.3333333333333333703, 0.3170188387650512141, 0.3333333333333333703),
 ( 0.3333333333333333703, 0.3170188387650512141, 0.3333333333333333703, 0.3170188387650512141, 0.3333333333333333703, 0.3170188387650512141, 0.3333333333333333703, 0.3170188387650512141, 0.3333333333333333703, 0.3170188387650512141, 0.3333333333333333703, 0.3170188387650512141, 0.3333333333333333703, 0.3170188387650512141, 0.3333333333333333703, 0.3170188387650512141, 0.3333333333333333703, 0.3170188387650512141, 0.3333333333333333703, 0.3170188387650512141, 0.3333333333333333703, 0.3170188387650512141, 0.3333333333333333703, 0.3170188387650512141, 0.3333333333333333703, 0.3170188387650512141, 0.3333333333333333703, 0.3170188387650512141, 0.3333333333333333703, 0.3170188387650512141, 0.3333333333333333703, 0.3170188387650512141, 0.3333333333333333703, 0.3170188387650512141, 0.3333333333333333703, 0.3170188387650512141, 0.3333333333333333703, 0.3170188387650512141, 0.3333333333333333703, 0.3170188387650512141, 0.3333333333333333703, 0.3170188387650512141, 0.3333333333333333703, 0.3170188387650512141, 0.3333333333333333703, 0.3170188387650512141, 0.3333333333333333703, 0.3170188387650512141, 0.3333333333333333703, 0.3170188387650512141, 0.3333333333333333703, 0.3170188387650512141, 0.3333333333333333703, 0.3170188387650512141, 0.3333333333333333703, 0.3170188387650512141, 0.3333333333333333703, 0.3170188387650512141, 0.3333333333333333703, 0.3170188387650512141, 0.3333333333333333703, 0.3170188387650512141, 0.3333333333333333703, 0.3170188387650512141, 0.3333333333333333703, 0.3170188387650512141, 0.3333333333333333703, 0.3170188387650512141, 0.3333333333333333703, 0.3170188387650512141, 0.3333333333333333703, 0.3170188387650512141, 0.3333333333333333703, 0.3170188387650512141, 0.3333333333333333703, 0.3170188387650512141, 0.3333333333333333703, 0.3170188387650512141, 0.3333333333333333703, 0.3170188387650512141, 0.3333333333333333703, 0.3170188387650512141, 0.3333333333333333703, 0.3170188387650512141, 0.3333333333333333703, 0.3170188387650512141, 0.3333333333333333703, 0.3170188387650512141, 0.3333333333333333703, 0.3170188387650512141, 0.3333333333333333703, 0.3170188387650512141, 0.3333333333333333703, 0.3170188387650512141, 0.3333333333333333703, 0.3170188387650512141, 0.3333333333333333703, 0.3170188387650512141, 0.3333333333333333703, 0.3170188387650512141, 0.3333333333333333703, 0.3170188387650512141, 0.3333333333333333703, 0.3170188387650512141, 0.3333333333333333703, 0.3170188387650512141, 0.3333333333333333703, 0.3170188387650512141, 0.3333333333333333703, 0.3170188387650512141, 0.3333333333333333703, 0.3170188387650512141, 0.3333333333333333703, 0.3170188387650512141, 0.3333333333333333703, 0.3170188387650512141, 0.3333333333333333703, 0.3170188387650512141, 0.3333333333333333703, 0.3170188387650512141, 0.3333333333333333703, 0.3170188387650512141, 0.3333333333333333703, 0.3170188387650512141, 0.3333333333333333703, 0.3170188387650512141, 0.3333333333333333703, 0.3170188387650512141, 0.3333333333333333703, 0.3170188387650512141, 0.3333333333333333703, 0.3170188387650512141, 0.3333333333333333703, 0.3170188387650512141, 0.3333333333333333703, 0.3170188387650512141, 0.3333333333333333703, 0.3170188387650512141, 0.3333333333333333703, 0.3170188387650512141, 0.3333333333333333703, 0.3170188387650512141, 0.3333333333333333703, 0.3170188387650512141, 0.3333333333333333703, 0.3170188387650512141, 0.3333333333333333703, 0.3170188387650512141, 0.3333333333333333703, 0.3170188387650512141, 0.3333333333333333703, 0.3170188387650512141, 0.3333333333333333703, 0.3170188387650512141, 0.3333333333333333703, 0.3170188387650512141, 0.3333333333333333703, 0.3170188387650512141, 0.3333333333333333703, 0.3170188387650512141, 0.3333333333333333703, 0.3170188387650512141, 0.3333333333333333703, 0.3170188387650512141, 0.3333333333333333703, 0.3170188387650512141, 0.3333333333333333703, 0.3170188387650512141, 0.3333333333333333703, 0.3170188387650512141, 0.3333333333333333703, 0.3170188387650512141, 0.3333333333333333703, 0.3170188387650512141, 0.3333333333333333703, 0.3170188387650512141, 0.3333333333333333703, 0.3170188387650512141, 0.3333333333333333703, 0.3170188387650512141, 0.3333333333333333703, 0.3170188387650512141, 0.3333333333333333703, 0.3170188387650512141, 0.3333333333333333703, 0.3170188387650512141, 0.3333333333333333703, 0.3170188387650512141, 0.3333333333333333703, 0.3170188387650512141, 0.3333333333333333703, 0.3170188387650512141, 0.3333333333333333703, 0.3170188387650512141, 0.3333333333333333703, 0.3170188387650512141, 0.3333333333333333703, 0.3170188387650512141, 0.3333333333333333703, 0.3170188387650512141, 0.3333333333333333703),
 ( 1.000000000000000000, 0.9510565162951535312, 1.000000000000000000, 0.9510565162951535312, 1.000000000000000000, 0.9510565162951535312, 1.000000000000000000, 0.9510565162951535312, 1.000000000000000000, 0.9510565162951535312, 1.000000000000000000, 0.9510565162951535312, 1.000000000000000000, 0.9510565162951535312, 1.000000000000000000, 0.9510565162951535312, 1.000000000000000000, 0.9510565162951535312, 1.000000000000000000, 0.9510565162951535312, 1.000000000000000000, 0.9510565162951535312, 1.000000000000000000, 0.9510565162951535312, 1.000000000000000000, 0.9510565162951535312, 1.000000000000000000, 0.9510565162951535312, 1.000000000000000000, 0.9510565162951535312, 1.000000000000000000, 0.9510565162951535312, 1.000000000000000000, 0.9510565162951535312, 1.000000000000000000, 0.9510565162951535312, 1.000000000000000000, 0.9510565162951535312, 1.000000000000000000, 0.9510565162951535312, 1.000000000000000000, 0.9510565162951535312, 1.000000000000000000, 0.9510565162951535312, 1.000000000000000000, 0.9510565162951535312, 1.000000000000000000, 0.9510565162951535312, 1.000000000000000000, 0.9510565162951535312, 1.000000000000000000, 0.9510565162951535312, 1.000000000000000000, 0.9510565162951535312, 1.000000000000000000, 0.9510565162951535312, 1.000000000000000000, 0.9510565162951535312, 1.000000000000000000, 0.9510565162951535312, 1.000000000000000000, 0.9510565162951535312, 1.000000000000000000, 0.9510565162951535312, 1.000000000000000000, 0.9510565162951535312, 1.000000000000000000, 0.9510565162951535312, 1.000000000000000000, 0.9510565162951535312, 1.000000000000000000, 0.9510565162951535312, 1.000000000000000000, 0.9510565162951535312, 1.000000000000000000, 0.9510565162951535312, 1.000000000000000000, 0.9510565162951535312, 1.000000000000000000, 0.9510565162951535312, 1.000000000000000000, 0.9510565162951535312, 1.000000000000000000, 0.9510565162951535312, 1.000000000000000000, 0.9510565162951535312, 1.000000000000000000, 0.9510565162951535312, 1.000000000000000000, 0.9510565162951535312, 1.000000000000000000, 0.9510565162951535312, 1.000000000000000000, 0.9510565162951535312, 1.000000000000000000, 0.9510565162951535312, 1.000000000000000000, 0.9510565162951535312, 1.000000000000000000, 0.9510565162951535312, 1.000000000000000000, 0.9510565162951535312, 1.000000000000000000, 0.9510565162951535312, 1.000000000000000000, 0.9510565162951535312, 1.000000000000000000, 0.9510565162951535312, 1.000000000000000000, 0.9510565162951535312, 1.000000000000000000, 0.9510565162951535312, 1.000000000000000000, 0.9510565162951535312, 1.000000000000000000, 0.9510565162951535312, 1.000000000000000000, 0.9510565162951535312, 1.000000000000000000, 0.9510565162951535312, 1.000000000000000000, 0.9510565162951535312, 1.000000000000000000, 0.9510565162951535312, 1.000000000000000000, 0.9510565162951535312, 1.000000000000000000, 0.9510565162951535312, 1.000000000000000000, 0.9510565162951535312, 1.000000000000000000, 0.9510565162951535312, 1.000000000000000000, 0.9510565162951535312, 1.000000000000000000, 0.9510565162951535312, 1.000000000000000000, 0.9510565162951535312, 1.000000000000000000, 0.9510565162951535312, 1.000000000000000000, 0.9510565162951535312, 1.000000000000000000, 0.9510565162951535312, 1.000000000000000000, 0.9510565162951535312, 1.000000000000000000, 0.9510565162951535312, 1.000000000000000000, 0.9510565162951535312, 1.000000000000000000, 0.9510565162951535312, 1.000000000000000000, 0.9510565162951535312, 1.000000000000000000, 0.9510565162951535312, 1.000000000000000000, 0.9510565162951535312, 1.000000000000000000, 0.9510565162951535312, 1.000000000000000000, 0.9510565162951535312, 1.000000000000000000, 0.9510565162951535312, 1.000000000000000000, 0.9510565162951535312, 1.000000000000000000, 0.9510565162951535312, 1.000000000000000000, 0.9510565162951535312, 1.000000000000000000, 0.9510565162951535312, 1.000000000000000000, 0.9510565162951535312, 1.000000000000000000, 0.9510565162951535312, 1.000000000000000000, 0.9510565162951535312, 1.000000000000000000, 0.9510565162951535312, 1.000000000000000000, 0.9510565162951535312, 1.000000000000000000, 0.9510565162951535312, 1.000000000000000000, 0.9510565162951535312, 1.000000000000000000, 0.9510565162951535312, 1.000000000000000000, 0.9510565162951535312, 1.000000000000000000, 0.9510565162951535312, 1.000000000000000000, 0.9510565162951535312, 1.000000000000000000, 0.9510565162951535312, 1.000000000000000000, 0.9510565162951535312, 1.000000000000000000, 0.9510565162951535312, 1.000000000000000000) ) ) 
 REPRESENTATION_ITEM ( '' )  SURFACE ( )  );
#12544=CARTESIAN_POINT ( 'NONE',  ( 49.97728705011495265, 51.50051614449765935, 7.000000000000000888 ) ) ;
#12545=CARTESIAN_POINT ( 'NONE',  ( 43.69122665457040000, 58.99948385550239749, 0.02388180880521036456 ) ) ;
#12558=CARTESIAN_POINT ( 'NONE',  ( 44.88205777487401349, 53.80051614449766362, 3.688883143319584779 ) ) ;
#12560=CARTESIAN_POINT ( 'NONE',  ( 47.74827507625478518, 62.59948385550240602, 7.007379884777227730 ) ) ;
#12561=CARTESIAN_POINT ( 'NONE',  ( 45.86712807150323812, 51.29948385550240175, -5.649768623646098220 ) ) ;
#12571=CARTESIAN_POINT ( 'NONE',  ( 49.97728705011488159, 45.49948385550240459, -7.000000000000000888 ) ) ;
#12572=CARTESIAN_POINT ( 'NONE',  ( 56.65037692655921120, 49.10051614449766078, 2.184720259617097593 ) ) ;
#12574=CARTESIAN_POINT ( 'NONE',  ( 55.96859303347804371, 46.19948385550238612, 4.306917132069425946 ) ) ;
#12576=CARTESIAN_POINT ( 'NONE',  ( 47.42335538002188144, 54.59948385550240602, 8.007379884777233059 ) ) ;
#12579=ORIENTED_EDGE ( 'NONE', *, *, #8305, .T. ) ;
#12583=( NAMED_UNIT ( * ) PLANE_ANGLE_UNIT ( ) SI_UNIT ( $, .RADIAN. ) );
#12587=CARTESIAN_POINT ( 'NONE',  ( 55.11794222512599362, 46.80051614449766362, -3.688883143319583446 ) ) ;
#12588=CARTESIAN_POINT ( 'NONE',  ( 54.09612160359792199, 61.30051614449766362, 5.676469297603124353 ) ) ;
#12590=CARTESIAN_POINT ( 'NONE',  ( 52.57664461997821093, 63.40051614449765083, 8.007379884777206414 ) ) ;
#12592=CARTESIAN_POINT ( 'NONE',  ( 57.61547081786810764, 58.90051614449766504, -2.450534656007114176 ) ) ;
#12598=DIRECTION ( 'NONE',  ( -0.04542589977017699732, 0.9989677110047501252, 0.000000000000000000 ) ) ;
#12604=CARTESIAN_POINT ( 'NONE',  ( 56.30877334542961421, 49.99948385550240459, -0.02388180880520959434 ) ) ;
#12606=CARTESIAN_POINT ( 'NONE',  ( 45.27934281921082516, 45.70051614449766220, 6.458785618021089192 ) ) ;
#12610=CARTESIAN_POINT ( 'NONE',  ( 54.13287192849671214, 48.70051614449766220, -5.649768623646139964 ) ) ;
#12611=CARTESIAN_POINT ( 'NONE',  ( 44.91013252490152752, 58.79948385550240175, 3.727524721679198461 ) ) ;
#12622=CARTESIAN_POINT ( 'NONE',  ( 52.25172492374522903, 53.59948385550241312, -7.007379884777225953 ) ) ;
#12624=CARTESIAN_POINT ( 'NONE',  ( 48.02776887271750184, 53.60051614449765367, 5.992620115222795363 ) ) ;
#12626=CARTESIAN_POINT ( 'NONE',  ( 43.33558569842703179, 65.09948385550239891, -2.141517661632099223 ) ) ;
#12627=CARTESIAN_POINT ( 'NONE',  ( 56.65037692655918988, 63.89948385550239607, -2.184720259617163762 ) ) ;
#12628=CARTESIAN_POINT ( 'NONE',  ( 43.34962307344081012, 56.89948385550240317, 2.184720259617164650 ) ) ;
#12640=CARTESIAN_POINT ( 'NONE',  ( 47.74827507625469281, 50.40051614449764372, -7.007379884777203749 ) ) ;
#12642=CARTESIAN_POINT ( 'NONE',  ( 56.65037692655918988, 47.89948385550240317, -2.184720259617163762 ) ) ;
#12644=CARTESIAN_POINT ( 'NONE',  ( 52.62207051974839089, 56.39948385550241028, 7.992620115222770494 ) ) ;
#12651=CARTESIAN_POINT ( 'NONE',  ( 49.97728705011494554, 49.50051614449766646, 6.000000000000000888 ) ) ;
#12652=CARTESIAN_POINT ( 'NONE',  ( 44.03140696652198471, 57.80051614449766362, 4.306917132069485454 ) ) ;
#12653=CARTESIAN_POINT ( 'NONE',  ( 47.37792948025162332, 49.39948385550241028, -7.992620115222770494 ) ) ;
#12655=CARTESIAN_POINT ( 'NONE',  ( 52.57664461997821093, 59.40051614449765793, 8.007379884777206414 ) ) ;
#12665=CARTESIAN_POINT ( 'NONE',  ( 46.45491332379572924, 53.29948385550240886, -4.840751629271157874 ) ) ;
#12666=CARTESIAN_POINT ( 'NONE',  ( 44.03140696652193498, 65.19948385550240744, -4.306917132069424170 ) ) ;
#12667=CARTESIAN_POINT ( 'NONE',  ( 54.68390685589039890, 45.30051614449766362, 6.485486291978072693 ) ) ;
#12671=CARTESIAN_POINT ( 'NONE',  ( 45.86712807150329496, 59.70051614449766220, 5.649768623646139964 ) ) ;
#12672=CARTESIAN_POINT ( 'NONE',  ( 56.30877334542961421, 57.99948385550241170, -0.02388180880520959434 ) ) ;
#12684=CARTESIAN_POINT ( 'NONE',  ( 57.36023556966787851, 51.99948385550238328, -0.02388180880522424582 ) ) ;
#12687=CARTESIAN_POINT ( 'NONE',  ( 56.30877334542961421, 55.00051614449766646, 0.02388180880515774693 ) ) ;
#12690=CARTESIAN_POINT ( 'NONE',  ( 44.03140696652192787, 63.19948385550240744, -4.306917132069425058 ) ) ;
#12692=CARTESIAN_POINT ( 'NONE',  ( 43.34962307344081012, 62.89948385550241028, 2.184720259617164650 ) ) ;
#12702=CARTESIAN_POINT ( 'NONE',  ( 56.65037692655918988, 47.89948385550240317, -2.184720259617163762 ) ) ;
#12703=CARTESIAN_POINT ( 'NONE',  ( 49.97728705011495265, 45.50051614449765935, 7.000000000000000888 ) ) ;
#12705=CARTESIAN_POINT ( 'NONE',  ( 47.42335538002188144, 64.59948385550241312, 8.007379884777233059 ) ) ;
#12707=CARTESIAN_POINT ( 'NONE',  ( 52.57664461997811856, 53.59948385550240602, -8.007379884777229506 ) ) ;
#12716=CARTESIAN_POINT ( 'NONE',  ( 48.02776887271750184, 45.60051614449765367, 5.992620115222795363 ) ) ;
#12717=CARTESIAN_POINT ( 'NONE',  ( 57.36023556966787851, 61.00051614449765935, 0.02388180880515038476 ) ) ;
#12718=CARTESIAN_POINT ( 'NONE',  ( 54.72065718078924590, 48.29948385550240175, 6.458785618021043895 ) ) ;
#12720=CARTESIAN_POINT ( 'NONE',  ( 58.41169779390614281, 59.00051614449766646, 0.02388180880515032231 ) ) ;
#12729=CARTESIAN_POINT ( 'NONE',  ( 51.92680522751233951, 49.59948385550241312, -6.007379884777223289 ) ) ;
#12731=CARTESIAN_POINT ( 'NONE',  ( 54.72065718078918906, 46.70051614449766220, -6.458785618021089192 ) ) ;
#12734=CARTESIAN_POINT ( 'NONE',  ( 52.29715082351538769, 54.60051614449766788, -6.992620115222796251 ) ) ;
#12735=CARTESIAN_POINT ( 'NONE',  ( 49.97728705011488870, 59.49948385550240459, -6.000000000000000888 ) ) ;
#12743=CARTESIAN_POINT ( 'NONE',  ( 49.97728705011488159, 53.49948385550240459, -7.000000000000000888 ) ) ;
#12745=CARTESIAN_POINT ( 'NONE',  ( 46.45491332379576477, 49.70051614449766220, 4.840751629271188961 ) ) ;
#12750=CARTESIAN_POINT ( 'NONE',  ( 54.09612160359786515, 61.69948385550240744, -5.676469297603166098 ) ) ;
#12764=CARTESIAN_POINT ( 'NONE',  ( 55.96859303347805081, 50.19948385550240744, 4.306917132069425058 ) ) ;
#12765=CARTESIAN_POINT ( 'NONE',  ( 43.34962307344078880, 46.10051614449766078, -2.184720259617096705 ) ) ;
#12769=CARTESIAN_POINT ( 'NONE',  ( 43.34962307344081012, 46.89948385550240317, 2.184720259617164650 ) ) ;
#12771=CARTESIAN_POINT ( 'NONE',  ( 45.31609314410967926, 54.69948385550240033, 6.485486291978119766 ) ) ;
#12779=CARTESIAN_POINT ( 'NONE',  ( 50.02271294988506156, 50.50051614449765935, -6.000000000000000888 ) ) ;
#12780=CARTESIAN_POINT ( 'NONE',  ( 49.97728705011495265, 61.50051614449765935, 7.000000000000000888 ) ) ;
#12781=CARTESIAN_POINT ( 'NONE',  ( 56.79116909180259398, 63.20051614449766220, 4.963592699178938972 ) ) ;
#12784=CARTESIAN_POINT ( 'NONE',  ( 56.81924384183006538, 54.80051614449764941, -4.924951120819380357 ) ) ;
#12789=CARTESIAN_POINT ( 'NONE',  ( 50.02271294988505446, 44.50051614449765935, -7.000000000000000888 ) ) ;
#12797=CARTESIAN_POINT ( 'NONE',  ( 53.50833635130540955, 47.69948385550240744, -4.867452303228209765 ) ) ;
#12799=CARTESIAN_POINT ( 'NONE',  ( 43.18075615816994173, 45.80051614449766362, 4.924951120819380357 ) ) ;
#12802=CARTESIAN_POINT ( 'NONE',  ( 43.33558569842706021, 55.90051614449765793, 2.141517661632167169 ) ) ;
#12803=CARTESIAN_POINT ( 'NONE',  ( 51.97223112728254790, 58.39948385550241028, 5.992620115222778487 ) ) ;
#12811=CARTESIAN_POINT ( 'NONE',  ( 50.02271294988512551, 50.49948385550240459, 7.000000000000000888 ) ) ;
#12814=CARTESIAN_POINT ( 'NONE',  ( 51.97223112728249816, 52.60051614449765367, -5.992620115222793586 ) ) ;
#12818=CARTESIAN_POINT ( 'NONE',  ( 44.05948171654949874, 60.79948385550240886, 4.345558710429105354 ) ) ;
#12831=CARTESIAN_POINT ( 'NONE',  ( 54.13287192849676188, 50.29948385550240175, 5.649768623646098220 ) ) ;
#12833=CARTESIAN_POINT ( 'NONE',  ( 49.97728705011495265, 55.50051614449766646, 7.000000000000000888 ) ) ;
#12834=CARTESIAN_POINT ( 'NONE',  ( 55.48859070151218020, 45.00000000000002132, -4.999999999999993783 ) ) ;
#12837=CARTESIAN_POINT ( 'NONE',  ( 56.66441430157296821, 50.09948385550240602, 2.141517661632100111 ) ) ;
#12839=CARTESIAN_POINT ( 'NONE',  ( 47.37792948025162332, 53.39948385550241028, -7.992620115222770494 ) ) ;
#12845=CARTESIAN_POINT ( 'NONE',  ( 46.45491332379576477, 57.70051614449766930, 4.840751629271188961 ) ) ;
#12846=CARTESIAN_POINT ( 'NONE',  ( 55.94051828345054389, 63.20051614449764799, 4.345558710429044957 ) ) ;
#12847=CARTESIAN_POINT ( 'NONE',  ( 45.27934281921075410, 49.29948385550240886, -6.458785618021043895 ) ) ;
#12849=CARTESIAN_POINT ( 'NONE',  ( 57.60143344285435774, 57.10051614449766788, 2.493737253992045044 ) ) ;
#12863=CARTESIAN_POINT ( 'NONE',  ( 50.02271294988511841, 52.49948385550241170, 6.000000000000000888 ) ) ;
#12864=CARTESIAN_POINT ( 'NONE',  ( 43.34962307344078880, 46.10051614449766078, -2.184720259617096705 ) ) ;
#12865=CARTESIAN_POINT ( 'NONE',  ( 58.41169779390614281, 49.00051614449765935, 0.02388180880515032231 ) ) ;
#12868=CARTESIAN_POINT ( 'NONE',  ( 45.90387839640208512, 58.30051614449766362, -5.676469297603124353 ) ) ;
#12869=CARTESIAN_POINT ( 'NONE',  ( 43.69122665457040000, 62.99948385550241170, 0.02388180880521036456 ) ) ;
#12877=CARTESIAN_POINT ( 'NONE',  ( 49.97728705011488159, 51.49948385550240459, -7.000000000000000888 ) ) ;
#12880=CARTESIAN_POINT ( 'NONE',  ( 46.45491332379576477, 55.70051614449766220, 4.840751629271188961 ) ) ;
#12885=CARTESIAN_POINT ( 'NONE',  ( 42.63976443033212860, 56.99948385550241170, 0.02388180880522514787 ) ) ;
#12898=CARTESIAN_POINT ( 'NONE',  ( 52.25172492374522903, 53.59948385550241312, -7.007379884777227730 ) ) ;
#12900=CARTESIAN_POINT ( 'NONE',  ( 55.96859303347802239, 56.80051614449764230, -4.306917132069484566 ) ) ;
#12902=CARTESIAN_POINT ( 'NONE',  ( 49.97728705011488159, 51.49948385550240459, -7.000000000000000888 ) ) ;
#12906=CARTESIAN_POINT ( 'NONE',  ( 50.02271294988513972, 60.49948385550240459, 8.000000000000001776 ) ) ;
#12912=CARTESIAN_POINT ( 'NONE',  ( 53.54508667620424234, 52.70051614449766220, -4.840751629271188961 ) ) ;
#12914=CARTESIAN_POINT ( 'NONE',  ( 52.57664461997811856, 53.59948385550240602, -8.007379884777229506 ) ) ;
#12915=CARTESIAN_POINT ( 'NONE',  ( 45.86712807150323812, 59.29948385550240175, -5.649768623646098220 ) ) ;
#12918=CARTESIAN_POINT ( 'NONE',  ( 57.61547081786812896, 46.09948385550240602, 2.450534656007040901 ) ) ;
#12927=CARTESIAN_POINT ( 'NONE',  ( 53.50833635130540955, 55.69948385550240744, -4.867452303228209765 ) ) ;
#12928=CARTESIAN_POINT ( 'NONE',  ( 45.90387839640208512, 48.30051614449765651, -5.676469297603124353 ) ) ;
#12930=CARTESIAN_POINT ( 'NONE',  ( 47.42335538002180328, 54.40051614449765793, -8.007379884777206414 ) ) ;
#12936=CARTESIAN_POINT ( 'NONE',  ( 56.66441430157294690, 56.90051614449766504, -2.141517661632166281 ) ) ;
#12943=CARTESIAN_POINT ( 'NONE',  ( 50.02271294988512551, 56.49948385550240459, 7.000000000000000888 ) ) ;
#12947=CARTESIAN_POINT ( 'NONE',  ( 53.50833635130544508, 57.30051614449767072, 4.867452303228181343 ) ) ;
#12950=CARTESIAN_POINT ( 'NONE',  ( 50.02271294988511841, 46.49948385550240459, 6.000000000000000888 ) ) ;
#12962=CARTESIAN_POINT ( 'NONE',  ( 44.03140696652193498, 53.19948385550240033, -4.306917132069424170 ) ) ;
#12964=CARTESIAN_POINT ( 'NONE',  ( 57.36023556966787851, 55.00051614449765225, 0.02388180880515038476 ) ) ;
#12967=CARTESIAN_POINT ( 'NONE',  ( 43.34962307344081012, 52.89948385550240317, 2.184720259617164650 ) ) ;
#12968=CARTESIAN_POINT ( 'NONE',  ( 43.34962307344081012, 48.89948385550240317, 2.184720259617164650 ) ) ;
#12970=CARTESIAN_POINT ( 'NONE',  ( 47.42335538002188144, 64.59948385550241312, 8.007379884777233059 ) ) ;
#12980=CARTESIAN_POINT ( 'NONE',  ( 55.69932041026405045, 53.10051614449767499, 1.875703265242156359 ) ) ;
#12982=CARTESIAN_POINT ( 'NONE',  ( 41.58830220609386430, 50.99948385550241170, 0.02388180880523263147 ) ) ;
#12983=CARTESIAN_POINT ( 'NONE',  ( 56.65037692655918988, 53.89948385550240317, -2.184720259617163762 ) ) ;
#12985=CARTESIAN_POINT ( 'NONE',  ( 56.79116909180259398, 61.20051614449766220, 4.963592699178938972 ) ) ;
#12998=CARTESIAN_POINT ( 'NONE',  ( 44.28664221472220675, 59.09948385550240602, -1.832500667257165317 ) ) ;
#12999=CARTESIAN_POINT ( 'NONE',  ( 55.96859303347802239, 46.80051614449766362, -4.306917132069484566 ) ) ;
#13000=CARTESIAN_POINT ( 'NONE',  ( 45.27934281921082516, 55.70051614449766220, 6.458785618021089192 ) ) ;
#13003=CARTESIAN_POINT ( 'NONE',  ( 56.66441430157294690, 62.90051614449765083, -2.141517661632166281 ) ) ;
#13015=CARTESIAN_POINT ( 'NONE',  ( 57.36023556966787851, 55.99948385550239038, -0.02388180880522424582 ) ) ;
#13018=CARTESIAN_POINT ( 'NONE',  ( 44.91013252490150620, 56.20051614449766220, -3.727524721679154940 ) ) ;
#13021=CARTESIAN_POINT ( 'NONE',  ( 55.96859303347802239, 46.80051614449767072, -4.306917132069484566 ) ) ;
#13022=CARTESIAN_POINT ( 'NONE',  ( 43.33558569842703179, 63.09948385550240602, -2.141517661632099223 ) ) ;
#13035=CARTESIAN_POINT ( 'NONE',  ( 49.97728705011495265, 53.50051614449765935, 7.000000000000000888 ) ) ;
#13037=CARTESIAN_POINT ( 'NONE',  ( 57.36023556966787851, 51.99948385550238328, -0.02388180880522424582 ) ) ;
#13040=CARTESIAN_POINT ( 'NONE',  ( 56.79116909180255135, 63.79948385550241596, -4.963592699179005585 ) ) ;
#13049=CARTESIAN_POINT ( 'NONE',  ( 53.50833635130544508, 55.30051614449765651, 4.867452303228181343 ) ) ;
#13051=CARTESIAN_POINT ( 'NONE',  ( 58.41169779390614281, 53.99948385550241170, -0.02388180880523160798 ) ) ;
#13052=CARTESIAN_POINT ( 'NONE',  ( 44.05948171654949874, 54.79948385550241596, 4.345558710429105354 ) ) ;
#13054=CARTESIAN_POINT ( 'NONE',  ( 43.20883090819742023, 64.20051614449766930, -4.963592699178938972 ) ) ;
#13069=CARTESIAN_POINT ( 'NONE',  ( 53.54508667620428497, 54.29948385550241596, 4.840751629271157874 ) ) ;
#13070=CARTESIAN_POINT ( 'NONE',  ( 50.02271294988505446, 52.50051614449766646, -8.000000000000001776 ) ) ;
#13075=CARTESIAN_POINT ( 'NONE',  ( 54.72065718078918906, 44.70051614449765509, -6.458785618021089192 ) ) ;
#13083=CARTESIAN_POINT ( 'NONE',  ( 47.74827507625478518, 60.59948385550239891, 7.007379884777227730 ) ) ;
#13085=CARTESIAN_POINT ( 'NONE',  ( 50.02271294988506156, 60.50051614449766646, -6.000000000000000888 ) ) ;
#13087=DIRECTION ( 'NONE',  ( 0.000000000000000000, -0.000000000000000000, 1.000000000000000000 ) ) ;
#13088=CARTESIAN_POINT ( 'NONE',  ( 48.07319477248762496, 62.40051614449765793, -6.007379884777208190 ) ) ;
#13089=CARTESIAN_POINT ( 'NONE',  ( 44.88205777487398507, 47.19948385550240744, -3.688883143319540814 ) ) ;
#13101=ADVANCED_FACE ( 'NONE', ( #4732 ), #2717, .T. ) ;
#13103=CARTESIAN_POINT ( 'NONE',  ( 44.03140696652198471, 53.80051614449766362, 4.306917132069485454 ) ) ;
#13106=CARTESIAN_POINT ( 'NONE',  ( 56.66441430157296821, 52.09948385550240602, 2.141517661632100111 ) ) ;
#13110=CARTESIAN_POINT ( 'NONE',  ( 47.42335538002188144, 60.59948385550240602, 8.007379884777233059 ) ) ;
#13120=CARTESIAN_POINT ( 'NONE',  ( 44.91013252490150620, 52.20051614449766220, -3.727524721679154940 ) ) ;
#13123=CARTESIAN_POINT ( 'NONE',  ( 47.37792948025162332, 51.39948385550241028, -7.992620115222770494 ) ) ;
#13124=CARTESIAN_POINT ( 'NONE',  ( 50.02271294988512551, 56.49948385550240459, 7.000000000000000888 ) ) ;
#13126=CARTESIAN_POINT ( 'NONE',  ( 56.81924384183011512, 46.19948385550240744, 4.924951120819313743 ) ) ;
#13137=CARTESIAN_POINT ( 'NONE',  ( 44.88205777487398507, 57.19948385550241454, -3.688883143319540814 ) ) ;
#13138=CARTESIAN_POINT ( 'NONE',  ( 52.29715082351539479, 48.60051614449766078, -6.992620115222796251 ) ) ;
#13139=CARTESIAN_POINT ( 'NONE',  ( 52.57664461997821093, 51.40051614449767214, 8.007379884777206414 ) ) ;
#13141=CARTESIAN_POINT ( 'NONE',  ( 54.23491683972284960, 45.00000000000001421, -4.999999999999999112 ) ) ;
#13142=CARTESIAN_POINT ( 'NONE',  ( 52.62207051974829852, 46.60051614449764656, -7.992620115222797139 ) ) ;
#13150=CARTESIAN_POINT ( 'NONE',  ( 55.94051828345050836, 57.79948385550238754, -4.345558710429104465 ) ) ;
#13151=CARTESIAN_POINT ( 'NONE',  ( 46.49166364869456913, 56.30051614449766362, -4.867452303228181343 ) ) ;
#13154=CARTESIAN_POINT ( 'NONE',  ( 45.86712807150329496, 47.70051614449766220, 5.649768623646139964 ) ) ;
#13155=CARTESIAN_POINT ( 'NONE',  ( 44.03140696652192787, 63.19948385550240744, -4.306917132069425058 ) ) ;
#13166=CARTESIAN_POINT ( 'NONE',  ( 47.70284917648459100, 59.60051614449765367, 6.992620115222796251 ) ) ;
#13169=CARTESIAN_POINT ( 'NONE',  ( 49.97728705011488159, 55.49948385550240459, -7.000000000000000888 ) ) ;
#13170=CARTESIAN_POINT ( 'NONE',  ( 45.90387839640214196, 48.69948385550240744, 5.676469297603166098 ) ) ;
#13171=CARTESIAN_POINT ( 'NONE',  ( 57.61547081786812896, 62.09948385550240602, 2.450534656007040901 ) ) ;
#13181=CARTESIAN_POINT ( 'NONE',  ( 55.71335778527780036, 58.90051614449766504, -1.832500667257213056 ) ) ;
#13183=CARTESIAN_POINT ( 'NONE',  ( 52.62207051974839089, 52.39948385550241028, 7.992620115222770494 ) ) ;
#13184=CARTESIAN_POINT ( 'NONE',  ( 50.02271294988512551, 54.49948385550240459, 7.000000000000000888 ) ) ;
#13186=CARTESIAN_POINT ( 'NONE',  ( 47.42335538002180328, 62.40051614449765793, -8.007379884777206414 ) ) ;
#13196=CARTESIAN_POINT ( 'NONE',  ( 55.69932041026404335, 53.89948385550240317, -1.875703265242203432 ) ) ;
#13197=CARTESIAN_POINT ( 'NONE',  ( 55.96859303347802239, 54.80051614449764941, -4.306917132069484566 ) ) ;
#13198=CARTESIAN_POINT ( 'NONE',  ( 43.18075615816994173, 51.80051614449766362, 4.924951120819380357 ) ) ;
#13201=CARTESIAN_POINT ( 'NONE',  ( 56.81924384183006538, 44.80051614449766362, -4.924951120819380357 ) ) ;
#13211=CARTESIAN_POINT ( 'NONE',  ( 43.34962307344081012, 56.89948385550240317, 2.184720259617164650 ) ) ;
#13213=CARTESIAN_POINT ( 'NONE',  ( 43.34962307344081012, 50.89948385550241028, 2.184720259617164650 ) ) ;
#13218=CARTESIAN_POINT ( 'NONE',  ( 52.25172492374527877, 45.40051614449766504, 7.007379884777203749 ) ) ;
#13219=CARTESIAN_POINT ( 'NONE',  ( 56.66441430157296821, 64.09948385550239891, 2.141517661632100111 ) ) ;
#13230=SHAPE_REPRESENTATION_RELATIONSHIP ( 'NONE' , 'NONE' ,  #4503, #383 ) ;
#13233=CARTESIAN_POINT ( 'NONE',  ( 43.33558569842706021, 57.90051614449766504, 2.141517661632167169 ) ) ;
#13236=CARTESIAN_POINT ( 'NONE',  ( 43.34962307344081012, 60.89948385550241028, 2.184720259617164650 ) ) ;
#13237=CARTESIAN_POINT ( 'NONE',  ( 45.86712807150323812, 49.29948385550240175, -5.649768623646098220 ) ) ;
#13239=CARTESIAN_POINT ( 'NONE',  ( 49.97728705011488159, 49.49948385550240459, -7.000000000000000888 ) ) ;
#13241=CIRCLE ( 'NONE', #11934, 0.4999999999999972244 ) ;
#13248=CARTESIAN_POINT ( 'NONE',  ( 44.30067958973594955, 64.10051614449766078, -1.875703265242155693 ) ) ;
#13251=CARTESIAN_POINT ( 'NONE',  ( 49.97728705011486738, 57.49948385550241170, -8.000000000000001776 ) ) ;
#13252=CARTESIAN_POINT ( 'NONE',  ( 43.34962307344081012, 64.89948385550239607, 2.184720259617164650 ) ) ;
#13254=CARTESIAN_POINT ( 'NONE',  ( 42.38452918213188525, 53.09948385550240602, -2.450534656007040013 ) ) ;
#13267=CARTESIAN_POINT ( 'NONE',  ( 48.07319477248768180, 60.59948385550240602, 6.007379884777225953 ) ) ;
#13268=CARTESIAN_POINT ( 'NONE',  ( 47.70284917648459810, 55.60051614449765367, 6.992620115222797139 ) ) ;
#13269=CARTESIAN_POINT ( 'NONE',  ( 43.20883090819742023, 58.20051614449766220, -4.963592699178938972 ) ) ;
#13276=CARTESIAN_POINT ( 'NONE',  ( 44.05948171654945611, 62.20051614449764799, -4.345558710429044069 ) ) ;
#13286=CARTESIAN_POINT ( 'NONE',  ( 50.02271294988511841, 46.49948385550240459, 6.000000000000000888 ) ) ;
#13287=CARTESIAN_POINT ( 'NONE',  ( 43.34962307344081012, 60.89948385550241028, 2.184720259617164650 ) ) ;
#13291=CARTESIAN_POINT ( 'NONE',  ( 48.07319477248762496, 64.40051614449764372, -6.007379884777208190 ) ) ;
#13292=CARTESIAN_POINT ( 'NONE',  ( 55.08986747509847248, 51.79948385550240175, -3.727524721679197572 ) ) ;
#13303=CARTESIAN_POINT ( 'NONE',  ( 54.09612160359792199, 59.30051614449766362, 5.676469297603124353 ) ) ;
#13305=CARTESIAN_POINT ( 'NONE',  ( 49.97728705011494554, 45.50051614449766646, 6.000000000000000888 ) ) ;
#13307=CARTESIAN_POINT ( 'NONE',  ( 49.97728705011488159, 61.49948385550240459, -7.000000000000000888 ) ) ;
#13308=CARTESIAN_POINT ( 'NONE',  ( 43.34962307344081012, 52.89948385550240317, 2.184720259617164650 ) ) ;
#13309=CARTESIAN_POINT ( 'NONE',  ( 43.33558569842703179, 51.09948385550240602, -2.141517661632099223 ) ) ;
#13316=CARTESIAN_POINT ( 'NONE',  ( 44.30067958973594955, 58.10051614449765367, -1.875703265242155693 ) ) ;
#13318=CARTESIAN_POINT ( 'NONE',  ( 54.68390685589033495, 59.69948385550240744, -6.485486291978119766 ) ) ;
#13319=CARTESIAN_POINT ( 'NONE',  ( 57.36023556966787851, 63.99948385550241881, -0.02388180880522424582 ) ) ;
#13321=CARTESIAN_POINT ( 'NONE',  ( 43.20883090819745576, 48.79948385550240175, 4.963592699179006473 ) ) ;
#13334=CARTESIAN_POINT ( 'NONE',  ( 55.11794222512601493, 60.19948385550240744, 3.688883143319541702 ) ) ;
#13335=CARTESIAN_POINT ( 'NONE',  ( 42.63976443033212149, 56.00051614449765225, -0.02388180880514948964 ) ) ;
#13338=CARTESIAN_POINT ( 'NONE',  ( 50.02271294988505446, 56.50051614449767357, -8.000000000000001776 ) ) ;
#13340=CARTESIAN_POINT ( 'NONE',  ( 54.72065718078918906, 52.70051614449766220, -6.458785618021089192 ) ) ;
#13353=CARTESIAN_POINT ( 'NONE',  ( 55.08986747509847248, 45.79948385550240886, -3.727524721679197572 ) ) ;
#13354=CARTESIAN_POINT ( 'NONE',  ( 42.63976443033212149, 56.99948385550241170, 0.02388180880522514787 ) ) ;
#13359=CARTESIAN_POINT ( 'NONE',  ( 45.86712807150329496, 51.70051614449766220, 5.649768623646139964 ) ) ;
#13360=CARTESIAN_POINT ( 'NONE',  ( 43.69122665457040000, 50.99948385550241170, 0.02388180880521036456 ) ) ;
#13370=CARTESIAN_POINT ( 'NONE',  ( 47.74827507625478518, 46.59948385550239891, 7.007379884777227730 ) ) ;
#13373=CARTESIAN_POINT ( 'NONE',  ( 53.54508667620424234, 46.70051614449766220, -4.840751629271188961 ) ) ;
#13375=CARTESIAN_POINT ( 'NONE',  ( 50.02271294988512551, 60.49948385550240459, 7.000000000000000888 ) ) ;
#13376=CARTESIAN_POINT ( 'NONE',  ( 52.25172492374522903, 53.59948385550241312, -7.007379884777225953 ) ) ;
#13378=CARTESIAN_POINT ( 'NONE',  ( 44.03140696652192787, 47.19948385550240744, -4.306917132069425058 ) ) ;
#13388=CARTESIAN_POINT ( 'NONE',  ( 43.69122665457040000, 62.00051614449766646, -0.02388180880515696977 ) ) ;
#13390=CARTESIAN_POINT ( 'NONE',  ( 47.37792948025162332, 59.39948385550240317, -7.992620115222770494 ) ) ;
#13391=CARTESIAN_POINT ( 'NONE',  ( 52.25172492374522903, 61.59948385550239891, -7.007379884777225953 ) ) ;
#13392=CARTESIAN_POINT ( 'NONE',  ( 50.02271294988505446, 64.50051614449765225, -7.000000000000000888 ) ) ;
#13393=CARTESIAN_POINT ( 'NONE',  ( 43.18075615816989199, 49.19948385550240744, -4.924951120819313743 ) ) ;
#13402=CARTESIAN_POINT ( 'NONE',  ( 44.91013252490152752, 60.79948385550241596, 3.727524721679198461 ) ) ;
#13403=CARTESIAN_POINT ( 'NONE',  ( 45.90387839640208512, 56.30051614449765651, -5.676469297603124353 ) ) ;
#13404=CARTESIAN_POINT ( 'NONE',  ( 52.62207051974829852, 58.60051614449766788, -7.992620115222797139 ) ) ;
#13407=CARTESIAN_POINT ( 'NONE',  ( 57.61547081786810764, 46.90051614449766504, -2.450534656007114176 ) ) ;
#13420=CARTESIAN_POINT ( 'NONE',  ( 47.70284917648453415, 61.39948385550241738, -6.992620115222774047 ) ) ;
#13422=CARTESIAN_POINT ( 'NONE',  ( 52.25172492374522903, 59.59948385550239891, -7.007379884777227730 ) ) ;
#13427=CARTESIAN_POINT ( 'NONE',  ( 43.33558569842706021, 47.90051614449765793, 2.141517661632167169 ) ) ;
#13428=CARTESIAN_POINT ( 'NONE',  ( 51.92680522751233951, 51.59948385550240602, -6.007379884777223289 ) ) ;
#13439=CARTESIAN_POINT ( 'NONE',  ( 55.71335778527780036, 46.90051614449766504, -1.832500667257213056 ) ) ;
#13441=CARTESIAN_POINT ( 'NONE',  ( 47.70284917648453415, 57.39948385550241028, -6.992620115222774047 ) ) ;
#13442=CARTESIAN_POINT ( 'NONE',  ( 49.97728705011488159, 53.49948385550240459, -7.000000000000000888 ) ) ;
#13445=CARTESIAN_POINT ( 'NONE',  ( 45.90387839640214196, 50.69948385550240744, 5.676469297603166098 ) ) ;
#13454=CARTESIAN_POINT ( 'NONE',  ( 52.25172492374522903, 47.59948385550240602, -7.007379884777227730 ) ) ;
#13455=CARTESIAN_POINT ( 'NONE',  ( 44.91013252490150620, 58.20051614449766220, -3.727524721679154940 ) ) ;
#13457=CARTESIAN_POINT ( 'NONE',  ( 47.42335538002188144, 58.59948385550239891, 8.007379884777233059 ) ) ;
#13461=CARTESIAN_POINT ( 'NONE',  ( 57.60143344285433642, 51.89948385550241028, -2.493737253992118319 ) ) ;
#13463=ORIENTED_EDGE ( 'NONE', *, *, #8044, .F. ) ;
#13471=CARTESIAN_POINT ( 'NONE',  ( 55.69932041026404335, 59.89948385550240317, -1.875703265242203432 ) ) ;
#13472=CARTESIAN_POINT ( 'NONE',  ( 52.25172492374528588, 51.40051614449767214, 7.007379884777204637 ) ) ;
#13473=CARTESIAN_POINT ( 'NONE',  ( 43.18075615816994173, 57.80051614449766362, 4.924951120819380357 ) ) ;
#13476=CARTESIAN_POINT ( 'NONE',  ( 50.02271294988505446, 48.50051614449765935, -8.000000000000001776 ) ) ;
#13488=CARTESIAN_POINT ( 'NONE',  ( 55.71335778527780747, 46.09948385550240602, 1.832500667257165983 ) ) ;
#13490=CARTESIAN_POINT ( 'NONE',  ( 50.02271294988512551, 58.49948385550241170, 7.000000000000000888 ) ) ;
#13495=CARTESIAN_POINT ( 'NONE',  ( 57.36023556966787851, 51.00051614449763804, 0.02388180880515038476 ) ) ;
#13496=CARTESIAN_POINT ( 'NONE',  ( 48.02776887271745210, 55.39948385550240317, -5.992620115222778487 ) ) ;
#13510=CARTESIAN_POINT ( 'NONE',  ( 44.91013252490150620, 46.20051614449766220, -3.727524721679154940 ) ) ;
#13512=CARTESIAN_POINT ( 'NONE',  ( 55.94051828345050836, 63.79948385550240886, -4.345558710429104465 ) ) ;
#13513=CARTESIAN_POINT ( 'NONE',  ( 52.29715082351547295, 56.39948385550238896, 6.992620115222774047 ) ) ;
#13517=CARTESIAN_POINT ( 'NONE',  ( 44.05948171654949874, 48.79948385550238754, 4.345558710429105354 ) ) ;
#13526=CARTESIAN_POINT ( 'NONE',  ( 44.05948171654949874, 48.79948385550239465, 4.345558710429104465 ) ) ;
#13528=CARTESIAN_POINT ( 'NONE',  ( 42.63976443033212860, 50.00051614449766646, -0.02388180880514948964 ) ) ;
#13531=CARTESIAN_POINT ( 'NONE',  ( 42.39856655714566358, 60.89948385550241028, 2.493737253992119207 ) ) ;
#13536=CARTESIAN_POINT ( 'NONE',  ( 54.72065718078924590, 48.29948385550240175, 6.458785618021043895 ) ) ;
#13545=CARTESIAN_POINT ( 'NONE',  ( 51.97223112728254790, 62.39948385550240317, 5.992620115222778487 ) ) ;
#13546=CARTESIAN_POINT ( 'NONE',  ( 42.63976443033212149, 60.00051614449765225, -0.02388180880514948964 ) ) ;
#13548=CARTESIAN_POINT ( 'NONE',  ( 56.79116909180259398, 57.20051614449766220, 4.963592699178938972 ) ) ;
#13551=CARTESIAN_POINT ( 'NONE',  ( 43.20883090819742023, 50.20051614449766220, -4.963592699178938972 ) ) ;
#13563=CARTESIAN_POINT ( 'NONE',  ( 57.36023556966787851, 61.99948385550241170, -0.02388180880522424582 ) ) ;
#13565=CARTESIAN_POINT ( 'NONE',  ( 55.96859303347805081, 60.19948385550240033, 4.306917132069425058 ) ) ;
#13566=CARTESIAN_POINT ( 'NONE',  ( 47.74827507625469281, 60.40051614449767214, -7.007379884777203749 ) ) ;
#13571=CARTESIAN_POINT ( 'NONE',  ( 55.94051828345053679, 51.20051614449766220, 4.345558710429044069 ) ) ;
#13572=CARTESIAN_POINT ( 'NONE',  ( 55.69932041026404335, 51.89948385550241028, -1.875703265242203432 ) ) ;
#13582=CARTESIAN_POINT ( 'NONE',  ( 57.36023556966787851, 45.99948385550238328, -0.02388180880522424582 ) ) ;
#13584=CARTESIAN_POINT ( 'NONE',  ( 56.30877334542961421, 53.00051614449765935, 0.02388180880515774693 ) ) ;
#13587=CARTESIAN_POINT ( 'NONE',  ( 54.13287192849676188, 54.29948385550240886, 5.649768623646098220 ) ) ;
#13590=CARTESIAN_POINT ( 'NONE',  ( 43.33558569842703179, 53.09948385550240602, -2.141517661632099223 ) ) ;
#13598=CARTESIAN_POINT ( 'NONE',  ( 57.36023556966787851, 49.00051614449763804, 0.02388180880515038476 ) ) ;
#13599=PRODUCT ( 'spring', 'spring', '', ( #2859 ) ) ;
#13601=CARTESIAN_POINT ( 'NONE',  ( 57.60143344285433642, 63.89948385550240317, -2.493737253992118319 ) ) ;
#13605=CARTESIAN_POINT ( 'NONE',  ( 54.68390685589033495, 53.69948385550240744, -6.485486291978119766 ) ) ;
#13610=CARTESIAN_POINT ( 'NONE',  ( 54.23491683972284960, 45.00000000000001421, -4.999999999999999112 ) ) ;
#13614=CARTESIAN_POINT ( 'NONE',  ( 53.54508667620424234, 48.70051614449766930, -4.840751629271188961 ) ) ;
#13615=CARTESIAN_POINT ( 'NONE',  ( 56.66441430157294690, 62.90051614449765083, -2.141517661632166281 ) ) ;
#13616=CARTESIAN_POINT ( 'NONE',  ( 52.62207051974839089, 46.39948385550240317, 7.992620115222770494 ) ) ;
#13618=CARTESIAN_POINT ( 'NONE',  ( 43.20883090819742023, 48.20051614449766930, -4.963592699178938972 ) ) ;
#13626=CARTESIAN_POINT ( 'NONE',  ( 53.50833635130540955, 49.69948385550240744, -4.867452303228209765 ) ) ;
#13627=CARTESIAN_POINT ( 'NONE',  ( 47.70284917648453415, 63.39948385550239607, -6.992620115222774047 ) ) ;
#13628=CARTESIAN_POINT ( 'NONE',  ( 47.70284917648459100, 61.60051614449764656, 6.992620115222796251 ) ) ;
#13633=CARTESIAN_POINT ( 'NONE',  ( 55.96859303347802239, 52.80051614449764941, -4.306917132069484566 ) ) ;
#13634=CARTESIAN_POINT ( 'NONE',  ( 53.54508667620428497, 56.29948385550240886, 4.840751629271157874 ) ) ;
#13645=CARTESIAN_POINT ( 'NONE',  ( 43.34962307344081012, 52.89948385550240317, 2.184720259617164650 ) ) ;
#13647=CARTESIAN_POINT ( 'NONE',  ( 44.88205777487401349, 49.80051614449765651, 3.688883143319584779 ) ) ;
#13651=CARTESIAN_POINT ( 'NONE',  ( 45.90387839640214196, 62.69948385550240744, 5.676469297603166098 ) ) ;
#13652=CARTESIAN_POINT ( 'NONE',  ( 54.13287192849676188, 62.29948385550240886, 5.649768623646098220 ) ) ;
#13661=CARTESIAN_POINT ( 'NONE',  ( 45.90387839640214196, 48.69948385550240744, 5.676469297603166098 ) ) ;
#13699=COLOUR_RGB('Grey',0.48,0.52,0.57);
#13700=FILL_AREA_STYLE_COLOUR('',#13699);
#13701=FILL_AREA_STYLE('',(#13700));
#13702=SURFACE_STYLE_FILL_AREA(#13701);
#13703=SURFACE_SIDE_STYLE('',(#13702));
#13704=SURFACE_STYLE_USAGE(.BOTH.,#13703);
#13705=PRESENTATION_STYLE_ASSIGNMENT((#13704));
ENDSEC;
END-ISO-10303-21;
